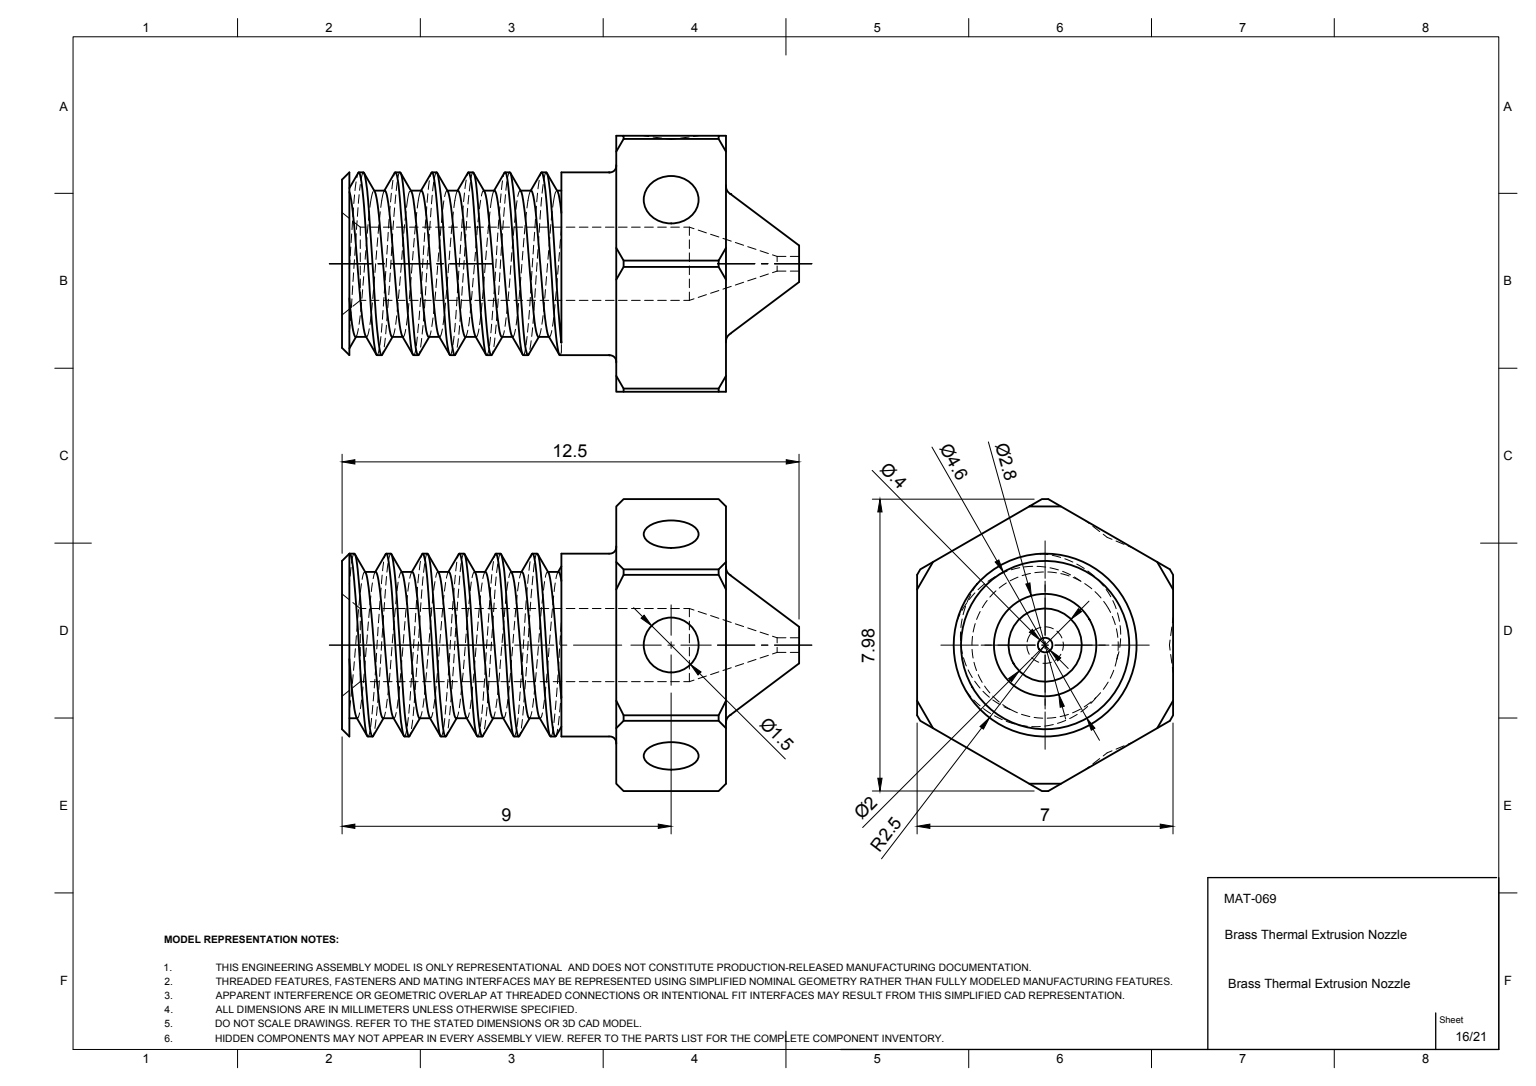
ISO-10303-21;
HEADER;
/* Generated by software containing ST-Developer
 * from STEP Tools, Inc. (www.steptools.com) 
 */

FILE_DESCRIPTION(
/* description */ ('CAx-IF Rec.Pracs.---Representation and Presentation of Product Manufa
cturing Information (PMI)---4.0---2014-10-13'),
/* implementation_level */ '2;1');

FILE_NAME(
/* name */ 'Brass Thermal Extrusion Nozzle.step',
/* time_stamp */ '2026-10-24T15:08:39-07:00',
/* author */ (''),
/* organization */ (''),
/* preprocessor_version */ 'ST-DEVELOPER v20.2',
/* originating_system */ 'Autodesk Translation Framework v15.17.0.0',
/* authorisation */ '');

FILE_SCHEMA (('AP242_MANAGED_MODEL_BASED_3D_ENGINEERING_MIM_LF { 1 0 10303 442 2 1 4 }'));
ENDSEC;

DATA;
#10=MECHANICAL_DESIGN_GEOMETRIC_PRESENTATION_REPRESENTATION('',(#833),#50081);
#110=B_SPLINE_SURFACE_WITH_KNOTS('',3,3,((#42024,#42025,#42026,#42027,#42028,
#42029,#42030,#42031,#42032,#42033),(#42034,#42035,#42036,#42037,#42038,
#42039,#42040,#42041,#42042,#42043),(#42044,#42045,#42046,#42047,#42048,
#42049,#42050,#42051,#42052,#42053),(#42054,#42055,#42056,#42057,#42058,
#42059,#42060,#42061,#42062,#42063),(#42064,#42065,#42066,#42067,#42068,
#42069,#42070,#42071,#42072,#42073),(#42074,#42075,#42076,#42077,#42078,
#42079,#42080,#42081,#42082,#42083),(#42084,#42085,#42086,#42087,#42088,
#42089,#42090,#42091,#42092,#42093)),.UNSPECIFIED.,.F.,.T.,.F.,(4,1,1,1,
4),(4,1,1,1,1,1,1,4),(-5.25936583692706E-5,0.285714285714286,0.5,0.785714285714286,
1.0342278679463),(-3.14159265358979,-2.24399475256414,-1.34639685153848,
-0.448798950512828,0.448798950512828,1.34639685153848,2.24399475256414,
3.14159265358979),.UNSPECIFIED.);
#111=B_SPLINE_SURFACE_WITH_KNOTS('',3,3,((#43523,#43524,#43525,#43526,#43527,
#43528,#43529,#43530,#43531,#43532),(#43533,#43534,#43535,#43536,#43537,
#43538,#43539,#43540,#43541,#43542),(#43543,#43544,#43545,#43546,#43547,
#43548,#43549,#43550,#43551,#43552),(#43553,#43554,#43555,#43556,#43557,
#43558,#43559,#43560,#43561,#43562),(#43563,#43564,#43565,#43566,#43567,
#43568,#43569,#43570,#43571,#43572),(#43573,#43574,#43575,#43576,#43577,
#43578,#43579,#43580,#43581,#43582),(#43583,#43584,#43585,#43586,#43587,
#43588,#43589,#43590,#43591,#43592)),.UNSPECIFIED.,.F.,.T.,.F.,(4,1,1,1,
4),(4,1,1,1,1,1,1,4),(0.,0.285714285714286,0.5,0.785714285714286,1.0345115737164),
(-9.42477796076937,-8.52718005974372,-7.62958215871806,-6.73198425769241,
-5.83438635666675,-4.9367884556411,-4.03919055461544,-3.14159265358979),
 .UNSPECIFIED.);
#112=B_SPLINE_SURFACE_WITH_KNOTS('',3,3,((#43768,#43769,#43770,#43771,#43772,
#43773,#43774,#43775,#43776,#43777),(#43778,#43779,#43780,#43781,#43782,
#43783,#43784,#43785,#43786,#43787),(#43788,#43789,#43790,#43791,#43792,
#43793,#43794,#43795,#43796,#43797),(#43798,#43799,#43800,#43801,#43802,
#43803,#43804,#43805,#43806,#43807),(#43808,#43809,#43810,#43811,#43812,
#43813,#43814,#43815,#43816,#43817),(#43818,#43819,#43820,#43821,#43822,
#43823,#43824,#43825,#43826,#43827),(#43828,#43829,#43830,#43831,#43832,
#43833,#43834,#43835,#43836,#43837)),.UNSPECIFIED.,.F.,.T.,.F.,(4,1,1,1,
4),(4,1,1,1,1,1,1,4),(-0.0291943928156984,0.285714285714286,0.571428571428571,
0.785714285714286,1.),(-3.14159265358979,-2.24399475256414,-1.34639685153848,
-0.448798950512828,0.448798950512828,1.34639685153848,2.24399475256414,
3.14159265358979),.UNSPECIFIED.);
#113=B_SPLINE_SURFACE_WITH_KNOTS('',3,3,((#43991,#43992,#43993,#43994,#43995,
#43996,#43997,#43998,#43999,#44000,#44001,#44002,#44003,#44004,#44005,#44006,
#44007,#44008,#44009,#44010,#44011,#44012,#44013,#44014,#44015,#44016,#44017,
#44018,#44019,#44020,#44021,#44022,#44023,#44024,#44025,#44026,#44027,#44028,
#44029,#44030,#44031,#44032),(#44033,#44034,#44035,#44036,#44037,#44038,
#44039,#44040,#44041,#44042,#44043,#44044,#44045,#44046,#44047,#44048,#44049,
#44050,#44051,#44052,#44053,#44054,#44055,#44056,#44057,#44058,#44059,#44060,
#44061,#44062,#44063,#44064,#44065,#44066,#44067,#44068,#44069,#44070,#44071,
#44072,#44073,#44074),(#44075,#44076,#44077,#44078,#44079,#44080,#44081,
#44082,#44083,#44084,#44085,#44086,#44087,#44088,#44089,#44090,#44091,#44092,
#44093,#44094,#44095,#44096,#44097,#44098,#44099,#44100,#44101,#44102,#44103,
#44104,#44105,#44106,#44107,#44108,#44109,#44110,#44111,#44112,#44113,#44114,
#44115,#44116),(#44117,#44118,#44119,#44120,#44121,#44122,#44123,#44124,
#44125,#44126,#44127,#44128,#44129,#44130,#44131,#44132,#44133,#44134,#44135,
#44136,#44137,#44138,#44139,#44140,#44141,#44142,#44143,#44144,#44145,#44146,
#44147,#44148,#44149,#44150,#44151,#44152,#44153,#44154,#44155,#44156,#44157,
#44158)),.UNSPECIFIED.,.F.,.F.,.F.,(4,4),(4,1,1,1,1,1,1,1,1,1,1,1,1,1,1,
1,1,1,1,1,1,1,1,1,1,1,1,1,1,1,1,1,1,1,1,1,1,1,1,4),(-0.000319347032471544,
0.058673081183855),(8.32512525661541,9.30615063831745,10.287080744622,11.2680108509265,
12.248940957231,13.2298710635355,14.21080116984,15.1917312761445,16.172661382449,
17.1535914887535,18.134521595058,19.1154517013625,20.096381807667,21.0773119139715,
22.0582420202761,23.0391721265806,24.0201022328851,25.0010323391896,25.9819624454941,
26.9628925517986,27.9438226581031,28.9247527644076,29.9056828707121,30.8866129770166,
31.8675430833211,32.8484731896256,33.8294032959301,34.8103334022347,35.7912635085392,
36.7721936148437,37.7531237211482,38.7340538274527,39.7149839337572,40.6959140400617,
41.6768441463662,42.6577742526707,43.6387043589752,44.6196344652797,45.6005645715842,
46.5816623403953),.UNSPECIFIED.);
#114=B_SPLINE_SURFACE_WITH_KNOTS('',3,3,((#44258,#44259,#44260,#44261,#44262,
#44263,#44264,#44265,#44266,#44267,#44268,#44269,#44270,#44271,#44272,#44273,
#44274,#44275,#44276,#44277,#44278,#44279,#44280,#44281,#44282,#44283,#44284,
#44285,#44286,#44287,#44288,#44289,#44290,#44291,#44292,#44293,#44294,#44295,
#44296,#44297,#44298,#44299),(#44300,#44301,#44302,#44303,#44304,#44305,
#44306,#44307,#44308,#44309,#44310,#44311,#44312,#44313,#44314,#44315,#44316,
#44317,#44318,#44319,#44320,#44321,#44322,#44323,#44324,#44325,#44326,#44327,
#44328,#44329,#44330,#44331,#44332,#44333,#44334,#44335,#44336,#44337,#44338,
#44339,#44340,#44341),(#44342,#44343,#44344,#44345,#44346,#44347,#44348,
#44349,#44350,#44351,#44352,#44353,#44354,#44355,#44356,#44357,#44358,#44359,
#44360,#44361,#44362,#44363,#44364,#44365,#44366,#44367,#44368,#44369,#44370,
#44371,#44372,#44373,#44374,#44375,#44376,#44377,#44378,#44379,#44380,#44381,
#44382,#44383),(#44384,#44385,#44386,#44387,#44388,#44389,#44390,#44391,
#44392,#44393,#44394,#44395,#44396,#44397,#44398,#44399,#44400,#44401,#44402,
#44403,#44404,#44405,#44406,#44407,#44408,#44409,#44410,#44411,#44412,#44413,
#44414,#44415,#44416,#44417,#44418,#44419,#44420,#44421,#44422,#44423,#44424,
#44425)),.UNSPECIFIED.,.F.,.F.,.F.,(4,4),(4,1,1,1,1,1,1,1,1,1,1,1,1,1,1,
1,1,1,1,1,1,1,1,1,1,1,1,1,1,1,1,1,1,1,1,1,1,1,1,4),(-0.000918461422766351,
0.0581489398467419),(12.0088396942433,12.9901384178654,13.9710685241699,
14.9519986304744,15.9329287367789,16.9138588430834,17.8947889493879,18.8757190556924,
19.8566491619969,20.8375792683014,21.8185093746059,22.7994394809105,23.780369587215,
24.7612996935195,25.742229799824,26.7231599061285,27.704090012433,28.6850201187375,
29.665950225042,30.6468803313465,31.627810437651,32.6087405439555,33.58967065026,
34.5706007565645,35.5515308628691,36.5324609691736,37.5133910754781,38.4943211817826,
39.4752512880871,40.4561813943916,41.4371115006961,42.4180416070006,43.3989717133051,
44.3799018196096,45.3608319259141,46.3417620322186,47.3226921385232,48.3036222448277,
49.2845523511322,50.2660355937093),.UNSPECIFIED.);
#457=B_SPLINE_CURVE_WITH_KNOTS('',3,(#40497,#40498,#40499,#40500,#40501,
#40502,#40503,#40504,#40505,#40506,#40507,#40508,#40509,#40510,#40511,#40512,
#40513,#40514,#40515,#40516,#40517,#40518,#40519,#40520,#40521,#40522,#40523,
#40524,#40525,#40526,#40527,#40528,#40529,#40530,#40531,#40532,#40533,#40534,
#40535,#40536,#40537,#40538,#40539,#40540,#40541,#40542,#40543,#40544,#40545,
#40546),.UNSPECIFIED.,.F.,.F.,(4,2,2,2,2,2,2,2,2,2,2,2,2,2,2,2,2,2,2,2,
2,2,2,2,4),(0.000209493712794322,0.0422872913938982,0.0542226665498989,
0.0656299001912059,0.0761984914852202,0.0887188350368748,0.144055532882821,
0.166979316880622,0.181775163552867,0.188803136528792,0.194952964302586,
0.204776397594916,0.236321457818492,0.28877412063129,0.301515346905665,
0.312233055563606,0.323797735338658,0.344187219178032,0.372232761612485,
0.42043174817154,0.429529383616972,0.435416861196921,0.440637222272047,
0.447327481728966,0.472483010091814),.UNSPECIFIED.);
#458=B_SPLINE_CURVE_WITH_KNOTS('',3,(#40549,#40550,#40551,#40552,#40553,
#40554,#40555,#40556,#40557,#40558,#40559,#40560,#40561,#40562,#40563,#40564,
#40565,#40566,#40567,#40568,#40569,#40570,#40571,#40572,#40573,#40574,#40575,
#40576,#40577,#40578),.UNSPECIFIED.,.F.,.F.,(4,2,2,2,2,2,2,2,2,2,2,2,2,
2,4),(9.99999999571378E-7,0.00565775487530941,0.0129173728394934,0.0519474282669346,
0.0924692038786361,0.106536967386471,0.118140574424233,0.132780272231367,
0.172415521622109,0.222944405297024,0.236545301367104,0.243410862645757,
0.249272230574711,0.258478354896224,0.275556593261106),.UNSPECIFIED.);
#459=B_SPLINE_CURVE_WITH_KNOTS('',3,(#40584,#40585,#40586,#40587,#40588,
#40589,#40590,#40591,#40592,#40593,#40594,#40595,#40596,#40597,#40598,#40599,
#40600,#40601,#40602,#40603,#40604,#40605,#40606,#40607,#40608,#40609,#40610,
#40611,#40612,#40613,#40614,#40615,#40616,#40617,#40618,#40619,#40620,#40621,
#40622,#40623,#40624,#40625,#40626,#40627,#40628,#40629,#40630,#40631,#40632,
#40633,#40634,#40635,#40636,#40637,#40638,#40639,#40640,#40641,#40642,#40643,
#40644,#40645,#40646,#40647,#40648,#40649,#40650,#40651,#40652,#40653,#40654,
#40655,#40656,#40657,#40658,#40659,#40660,#40661,#40662,#40663,#40664,#40665,
#40666,#40667,#40668,#40669,#40670,#40671,#40672,#40673,#40674,#40675,#40676,
#40677,#40678,#40679,#40680,#40681,#40682,#40683,#40684,#40685,#40686,#40687,
#40688,#40689,#40690,#40691,#40692,#40693,#40694,#40695,#40696,#40697,#40698,
#40699,#40700,#40701,#40702,#40703,#40704,#40705,#40706,#40707,#40708,#40709,
#40710,#40711,#40712,#40713,#40714,#40715,#40716,#40717,#40718,#40719,#40720,
#40721,#40722,#40723,#40724,#40725,#40726,#40727,#40728,#40729,#40730,#40731,
#40732,#40733,#40734,#40735,#40736,#40737,#40738,#40739,#40740,#40741),
 .UNSPECIFIED.,.F.,.F.,(4,2,2,2,2,2,2,2,2,2,2,2,2,2,2,2,2,2,2,2,2,2,2,2,
2,2,2,2,2,2,2,2,2,2,2,2,2,2,2,2,2,2,2,2,2,2,2,2,2,2,2,2,2,2,2,2,2,2,2,2,
2,2,2,2,2,2,2,2,2,2,2,2,2,2,2,2,2,2,4),(6.30435270860889,6.33486878320123,
6.34366974614675,6.34966324284323,6.35703713755435,6.37420620250057,6.40375264025194,
6.4470390695231,6.46203191150256,6.47264308026978,6.48406809681009,6.50407751685343,
6.53144912706435,6.58091498964814,6.58971900104101,6.59571521178631,6.60309649351356,
6.62029862705322,6.64995101906424,6.693024043224,6.708012300807,6.71862649719076,
6.73006138331729,6.75011057786636,6.7775645954391,6.82685633546438,6.83568099086117,
6.84167591283988,6.8490295334854,6.8660798204813,6.89526589896446,6.93907381839847,
6.9540616271593,6.96466389709236,6.97607323881813,6.99603127669263,7.02329568207772,
7.07302291161279,7.08179288524694,7.087779399277,7.09516137744094,7.11239908891738,
7.14215363461921,7.18521725183071,7.20021562855414,7.21082892841909,7.22225457039669,
7.24226256268532,7.26963720002217,7.31902650273789,7.3278387071296,7.3338469765065,
7.34126629547086,7.35864634523377,7.3888709987462,7.43087825960643,7.44583940029455,
7.45646854729715,7.46795493496144,7.48821541141176,7.51611323660128,7.56446287865684,
7.57339841015601,7.57939406940583,7.586623356302,7.60299394716167,7.63017917440611,
7.67742899532298,7.69229453732945,7.70282865451226,7.71416963637204,7.73398882738903,
7.76099878006726,7.81118536759106,7.81992573892269,7.82589410585711,7.83325762804537,
7.84165606901659,7.87995889022397),.UNSPECIFIED.);
#460=B_SPLINE_CURVE_WITH_KNOTS('',3,(#40742,#40743,#40744,#40745),
 .UNSPECIFIED.,.F.,.F.,(4,4),(1.01357413598985E-6,0.000209493712794322),
 .UNSPECIFIED.);
#461=B_SPLINE_CURVE_WITH_KNOTS('',3,(#40746,#40747,#40748,#40749,#40750,
#40751,#40752,#40753,#40754,#40755,#40756,#40757,#40758,#40759,#40760,#40761,
#40762,#40763,#40764,#40765,#40766,#40767,#40768,#40769,#40770,#40771,#40772,
#40773,#40774,#40775,#40776,#40777,#40778,#40779,#40780,#40781,#40782,#40783,
#40784,#40785,#40786,#40787,#40788,#40789,#40790,#40791,#40792,#40793,#40794,
#40795,#40796,#40797,#40798,#40799,#40800,#40801,#40802,#40803,#40804,#40805,
#40806,#40807,#40808,#40809,#40810,#40811,#40812,#40813,#40814,#40815,#40816,
#40817,#40818,#40819,#40820,#40821,#40822,#40823,#40824,#40825,#40826,#40827,
#40828,#40829,#40830,#40831,#40832,#40833,#40834,#40835,#40836,#40837,#40838,
#40839,#40840,#40841,#40842,#40843,#40844,#40845,#40846,#40847,#40848,#40849,
#40850,#40851,#40852,#40853,#40854,#40855,#40856,#40857,#40858,#40859,#40860,
#40861,#40862,#40863,#40864,#40865,#40866,#40867,#40868,#40869,#40870,#40871,
#40872,#40873,#40874,#40875,#40876,#40877,#40878,#40879,#40880,#40881,#40882,
#40883,#40884,#40885,#40886,#40887,#40888,#40889,#40890,#40891,#40892,#40893,
#40894,#40895,#40896,#40897,#40898,#40899,#40900,#40901),.UNSPECIFIED.,
 .F.,.F.,(4,2,2,2,2,2,2,2,2,2,2,2,2,2,2,2,2,2,2,2,2,2,2,2,2,2,2,2,2,2,2,
2,2,2,2,2,2,2,2,2,2,2,2,2,2,2,2,2,2,2,2,2,2,2,2,2,2,2,2,2,2,2,2,2,2,2,2,
2,2,2,2,2,2,2,2,2,2,4),(0.275556593261106,0.302257716093375,0.332145449002062,
0.353019638320446,0.364182811346166,0.374094054396295,0.387016365935024,
0.424468399690209,0.474784838723073,0.486382245753939,0.49262015904604,
0.498086515168979,0.507668815230086,0.549849706736197,0.580898810950735,
0.602581422114444,0.614391844510637,0.625103828088379,0.639873751023731,
0.68612813271093,0.712253967143993,0.728243775062982,0.73554602991629,0.741707481959803,
0.751244469819963,0.794030213469046,0.824223859030593,0.845430043251126,
0.857061734857099,0.867632782348189,0.882182911159433,0.941047537998989,
0.96150213928913,0.97527996369794,0.982123309918813,0.98815353536044,0.997879223181914,
1.04633441080135,1.07317249406427,1.09290377583721,1.10421640948278,1.11473376705714,
1.12958982902173,1.17659174660286,1.20386064199112,1.22025213524982,1.22747630986562,
1.23345821413433,1.24235725539788,1.29095061193003,1.3187384153877,1.33893993740818,
1.35040225813014,1.36101160205548,1.37594642745454,1.41769551255673,1.4480412350592,
1.46544943938522,1.47286386661574,1.47885850768789,1.4876337927126,1.5372593554286,
1.56452795041183,1.58447799162328,1.59587951676874,1.60647281319572,1.62144445402929,
1.66411223318268,1.69407854731155,1.7113737724098,1.7187549102345,1.72472703980151,
1.73345363173632,1.78346592748571,1.81060244195952,1.83049217765482,1.84187542645257,
1.85022063120531),.UNSPECIFIED.);
#462=B_SPLINE_CURVE_WITH_KNOTS('',3,(#40906,#40907,#40908,#40909,#40910,
#40911,#40912,#40913,#40914,#40915,#40916,#40917,#40918,#40919,#40920,#40921,
#40922,#40923,#40924,#40925,#40926,#40927,#40928,#40929,#40930,#40931,#40932,
#40933,#40934,#40935,#40936,#40937,#40938,#40939,#40940,#40941,#40942,#40943,
#40944,#40945,#40946,#40947,#40948,#40949,#40950,#40951,#40952,#40953,#40954,
#40955,#40956,#40957,#40958,#40959,#40960,#40961,#40962,#40963,#40964,#40965,
#40966,#40967,#40968,#40969,#40970,#40971,#40972,#40973,#40974,#40975,#40976,
#40977,#40978,#40979,#40980,#40981,#40982,#40983,#40984,#40985,#40986,#40987,
#40988,#40989,#40990,#40991,#40992,#40993,#40994,#40995,#40996,#40997,#40998,
#40999,#41000,#41001,#41002,#41003,#41004,#41005,#41006,#41007,#41008,#41009,
#41010,#41011,#41012,#41013,#41014,#41015,#41016,#41017,#41018,#41019,#41020,
#41021,#41022,#41023,#41024,#41025,#41026,#41027,#41028,#41029,#41030,#41031,
#41032,#41033,#41034,#41035,#41036,#41037,#41038,#41039,#41040,#41041,#41042,
#41043,#41044,#41045,#41046,#41047,#41048,#41049,#41050,#41051,#41052,#41053,
#41054,#41055,#41056,#41057,#41058,#41059,#41060,#41061,#41062,#41063),
 .UNSPECIFIED.,.F.,.F.,(4,2,2,2,2,2,2,2,2,2,2,2,2,2,2,2,2,2,2,2,2,2,2,2,
2,2,2,2,2,2,2,2,2,2,2,2,2,2,2,2,2,2,2,2,2,2,2,2,2,2,2,2,2,2,2,2,2,2,2,2,
2,2,2,2,2,2,2,2,2,2,2,2,2,2,2,2,2,2,4),(4.72819048267577,4.73950795185586,
4.75012210979889,4.76155086895958,4.78156836809081,4.80895190741352,4.85843117911358,
4.86723766046422,4.87323362414742,4.88060942980026,4.89778064245953,4.92732947790588,
4.97061576111725,4.98561061430102,4.99622420623809,5.00765283970181,5.02767158171161,
5.05505859474814,5.10452501033381,5.11333238041157,5.119328288513,5.12670325752487,
5.14386935222794,5.17340318557322,5.21670622262401,5.23170062699955,5.24231393095466,
5.25374230849599,5.27376083811829,5.30114790257251,5.35061005460223,5.35941738370218,
5.3654130554825,5.37278737207586,5.38995088389089,5.41947774454824,5.46278794072297,
5.47778169663862,5.4883943710803,5.49982188080286,5.51983816805462,5.54722109224304,
5.59668877283127,5.6054948237148,5.61149004333747,5.61886426512492,5.63602890233187,
5.6655599240848,5.70886382307828,5.72385725358769,5.73446957571265,5.74589658496825,
5.76591167794044,5.79329281107251,5.84275834566241,5.85156409224043,5.85755945109383,
5.86493479128113,5.88210548756745,5.91165646761162,5.95492013716683,5.9699124918867,
5.98052501497582,5.99195326255171,6.0119740552566,6.03936750252539,6.08880259339068,
6.09761148824992,6.10360662335611,6.11097785502081,6.1281262103999,6.15760933171281,
6.20097342104773,6.21596522841018,6.22657577246508,6.23800016613919,6.25800788400909,
6.28537444195454,6.30435270860889),.UNSPECIFIED.);
#463=B_SPLINE_CURVE_WITH_KNOTS('',3,(#41064,#41065,#41066,#41067,#41068,
#41069,#41070,#41071,#41072,#41073,#41074,#41075,#41076,#41077,#41078,#41079,
#41080,#41081,#41082,#41083,#41084,#41085,#41086,#41087,#41088,#41089,#41090,
#41091,#41092,#41093,#41094,#41095,#41096,#41097,#41098,#41099,#41100,#41101,
#41102,#41103,#41104,#41105,#41106,#41107,#41108,#41109,#41110,#41111,#41112,
#41113,#41114,#41115,#41116,#41117,#41118,#41119,#41120,#41121,#41122,#41123,
#41124,#41125,#41126,#41127,#41128,#41129,#41130,#41131,#41132,#41133,#41134,
#41135,#41136,#41137,#41138,#41139,#41140,#41141,#41142,#41143,#41144,#41145,
#41146,#41147,#41148,#41149,#41150,#41151,#41152,#41153,#41154,#41155,#41156,
#41157,#41158,#41159,#41160,#41161,#41162,#41163,#41164,#41165,#41166,#41167,
#41168,#41169,#41170,#41171,#41172,#41173,#41174,#41175,#41176,#41177,#41178,
#41179,#41180,#41181,#41182,#41183,#41184,#41185,#41186,#41187,#41188,#41189,
#41190,#41191,#41192,#41193,#41194,#41195,#41196,#41197,#41198,#41199,#41200,
#41201,#41202,#41203,#41204,#41205,#41206,#41207,#41208,#41209,#41210,#41211,
#41212,#41213,#41214,#41215,#41216,#41217,#41218,#41219),.UNSPECIFIED.,
 .F.,.F.,(4,2,2,2,2,2,2,2,2,2,2,2,2,2,2,2,2,2,2,2,2,2,2,2,2,2,2,2,2,2,2,
2,2,2,2,2,2,2,2,2,2,2,2,2,2,2,2,2,2,2,2,2,2,2,2,2,2,2,2,2,2,2,2,2,2,2,2,
2,2,2,2,2,2,2,2,2,2,4),(1.85022063120531,1.85245803545648,1.86742343567781,
1.91092677999263,1.94025068089833,1.95733584714856,1.9646854274236,1.97066601700574,
1.97945105943726,2.02899469267185,2.05633207510499,2.07631803047564,2.08772733025059,
2.09832096608194,2.11328308319158,2.15603372225511,2.18584052738125,2.20308163037672,
2.21045914351855,2.21644079802621,2.22520415870899,2.27492501537538,2.30217744978419,
2.32212212808228,2.33352104296743,2.34411139064825,2.35907813354066,2.40202494263366,
2.43173414326021,2.448944807865,2.45631516411609,2.46229382809607,2.47105314309451,
2.5208064963315,2.54805044763132,2.56799158078089,2.57938927809238,2.58997869927616,
2.60494442056477,2.64798095380983,2.67761542931793,2.69480159722625,2.70216859579123,
2.7081487224768,2.71691624692997,2.76660392905713,2.79387563535955,2.81382999658193,
2.82523127782325,2.83582222281463,2.85078748140468,2.89371885123636,2.92342331327636,
2.94063208540719,2.94800303400513,2.95398316784399,2.96274709136088,3.0124644483609,
3.03972253770116,3.05967032655013,3.07106994252096,3.08166033426212,3.09662625340397,
3.13959336916278,3.1692785866773,3.18648130065975,3.19385096254273,3.19983073143358,
3.20859451245861,3.2583134518259,3.28557185055764,3.3055198931902,3.31691956705066,
3.32750995083086,3.34247577477007,3.38545424338359,3.41512952594777,3.42490669701472),
 .UNSPECIFIED.);
#464=B_SPLINE_CURVE_WITH_KNOTS('',3,(#41224,#41225,#41226,#41227,#41228,
#41229,#41230,#41231,#41232,#41233,#41234,#41235,#41236,#41237,#41238,#41239,
#41240,#41241,#41242,#41243,#41244,#41245,#41246,#41247,#41248,#41249,#41250,
#41251,#41252,#41253,#41254,#41255,#41256,#41257,#41258,#41259,#41260,#41261,
#41262,#41263,#41264,#41265,#41266,#41267,#41268,#41269,#41270,#41271,#41272,
#41273,#41274,#41275,#41276,#41277,#41278,#41279,#41280,#41281,#41282,#41283,
#41284,#41285,#41286,#41287,#41288,#41289,#41290,#41291,#41292,#41293,#41294,
#41295,#41296,#41297,#41298,#41299,#41300,#41301,#41302,#41303,#41304,#41305,
#41306,#41307,#41308,#41309,#41310,#41311,#41312,#41313,#41314,#41315,#41316,
#41317,#41318,#41319,#41320,#41321,#41322,#41323,#41324,#41325,#41326,#41327,
#41328,#41329,#41330,#41331,#41332,#41333,#41334,#41335,#41336,#41337,#41338,
#41339,#41340,#41341,#41342,#41343,#41344,#41345,#41346,#41347,#41348,#41349,
#41350,#41351,#41352,#41353,#41354,#41355,#41356,#41357,#41358,#41359,#41360,
#41361,#41362,#41363,#41364,#41365,#41366,#41367,#41368,#41369,#41370,#41371,
#41372,#41373,#41374,#41375,#41376,#41377,#41378,#41379),.UNSPECIFIED.,
 .F.,.F.,(4,2,2,2,2,2,2,2,2,2,2,2,2,2,2,2,2,2,2,2,2,2,2,2,2,2,2,2,2,2,2,
2,2,2,2,2,2,2,2,2,2,2,2,2,2,2,2,2,2,2,2,2,2,2,2,2,2,2,2,2,2,2,2,2,2,2,2,
2,2,2,2,2,2,2,2,2,2,4),(3.15163477931716,3.15298897800685,3.16238915291939,
3.20652316777823,3.23631453510694,3.25737596078581,3.26897275867627,3.27952566483782,
3.29407041532064,3.35235036865309,3.3728309815977,3.3866151299212,3.39346659347139,
3.39954852935888,3.40941344026376,3.44468995601634,3.47940486850441,3.5023744208504,
3.51426586598204,3.52474840048023,3.53842769924747,3.59544554110014,3.61777418371048,
3.6323332685606,3.63931464019944,3.64534505137541,3.65487513183864,3.69766251601296,
3.72811334463534,3.74944920047817,3.76109086059298,3.77163275342468,3.78607775600029,
3.8449932390036,3.86524842884655,3.87893564142306,3.88577126146191,3.8918620139421,
3.90177670873891,3.93886568365411,3.98643481968158,4.00130483072224,4.01190269193801,
4.02337820046101,4.04367536038818,4.07168373699399,4.11973819691762,4.12870546523491,
4.13471998074014,4.14200401683087,4.15852421519058,4.18610554687911,4.23240953690924,
4.24734931712728,4.25795632477907,4.26940615582526,4.28954829302094,4.31720844817241,
4.3660547580922,4.37493356713054,4.3809377544045,4.38827163283667,4.4051410940172,
4.43376174987304,4.47841465989933,4.49340541599483,4.50401914264897,4.5154505679836,
4.53548223967792,4.56289658186719,4.61230833309369,4.62112304563995,4.6271200943582,
4.6344914860604,4.65162945556555,4.68107395400867,4.7245115038362,4.72819048267577),
 .UNSPECIFIED.);
#465=B_SPLINE_CURVE_WITH_KNOTS('',3,(#41380,#41381,#41382,#41383,#41384,
#41385,#41386,#41387,#41388,#41389,#41390,#41391,#41392,#41393,#41394,#41395,
#41396,#41397,#41398,#41399,#41400,#41401,#41402,#41403,#41404,#41405,#41406,
#41407,#41408,#41409,#41410,#41411,#41412,#41413,#41414,#41415,#41416,#41417,
#41418,#41419,#41420,#41421,#41422,#41423,#41424,#41425,#41426,#41427,#41428,
#41429,#41430,#41431,#41432,#41433,#41434,#41435,#41436,#41437,#41438,#41439,
#41440,#41441,#41442,#41443,#41444,#41445,#41446,#41447,#41448,#41449,#41450,
#41451,#41452,#41453,#41454,#41455,#41456,#41457,#41458,#41459,#41460,#41461,
#41462,#41463,#41464,#41465,#41466,#41467,#41468,#41469,#41470,#41471,#41472,
#41473,#41474,#41475,#41476,#41477,#41478,#41479,#41480,#41481,#41482,#41483,
#41484,#41485,#41486,#41487,#41488,#41489,#41490,#41491,#41492,#41493,#41494,
#41495,#41496,#41497,#41498,#41499,#41500,#41501,#41502,#41503,#41504,#41505,
#41506,#41507,#41508,#41509,#41510,#41511,#41512,#41513,#41514,#41515,#41516,
#41517,#41518,#41519,#41520,#41521,#41522,#41523,#41524,#41525,#41526,#41527,
#41528,#41529,#41530,#41531,#41532,#41533,#41534,#41535,#41536,#41537,#41538,
#41539),.UNSPECIFIED.,.F.,.F.,(4,2,2,2,2,2,2,2,2,2,2,2,2,2,2,2,2,2,2,2,
2,2,2,2,2,2,2,2,2,2,2,2,2,2,2,2,2,2,2,2,2,2,2,2,2,2,2,2,2,2,2,2,2,2,2,2,
2,2,2,2,2,2,2,2,2,2,2,2,2,2,2,2,2,2,2,2,2,2,2,4),(3.42490669701472,3.43232900937426,
3.43969829801849,3.44567833743907,3.45444340772131,3.50415231677713,3.53141504241583,
3.55136514504334,3.56276536765941,3.5733559672353,3.58832164819124,3.63127353358472,
3.66096759078479,3.6781731340077,3.68554337761954,3.69152334799716,3.70028723094562,
3.75000664143778,3.77726495614238,3.79721303103668,3.80861285460821,3.81920347093602,
3.83416980904366,3.87717038552534,3.90683077511809,3.92402561123087,3.9313943222146,
3.9373744942306,3.94614063170833,3.9958408787074,4.02310765778037,4.04305960357326,
4.05446010444556,4.06505052396108,4.08001514446103,4.1228808607337,4.15263751223124,
4.16986304230536,4.17723603423089,4.18321554998337,4.19197490861075,4.24173491283261,
4.26897644454247,4.28891702452145,4.30031571146024,4.31090697332087,4.32587722245906,
4.36937895902415,4.39868650088571,4.41576813047898,4.4231211723634,4.42910412598506,
4.43646726570338,4.45971562472414,4.50520763102599,4.53139557445127,4.54371433568145,
4.5541180054599,4.56730274768906,4.60218149192356,4.65148806356465,4.66391775308509,
4.67052045405102,4.67679960714132,4.68750057680989,4.7015915514247,4.74262703357355,
4.77468881107418,4.78787526656112,4.79827946517432,4.81059788314442,4.83678448185971,
4.88228453828832,4.90548434936197,4.91284436066545,4.91882714926359,4.92618309784467,
4.94328338218393,4.97264560048608,4.99969446742076),.UNSPECIFIED.);
#466=B_SPLINE_CURVE_WITH_KNOTS('',3,(#41544,#41545,#41546,#41547,#41548,
#41549,#41550,#41551,#41552,#41553,#41554,#41555,#41556,#41557,#41558,#41559,
#41560,#41561,#41562,#41563,#41564,#41565,#41566,#41567,#41568,#41569,#41570,
#41571,#41572,#41573,#41574,#41575,#41576,#41577,#41578,#41579,#41580,#41581,
#41582,#41583,#41584,#41585,#41586,#41587,#41588,#41589,#41590,#41591,#41592,
#41593,#41594,#41595,#41596,#41597,#41598,#41599,#41600,#41601,#41602,#41603,
#41604,#41605,#41606,#41607,#41608,#41609,#41610,#41611,#41612,#41613,#41614,
#41615,#41616,#41617,#41618,#41619,#41620,#41621,#41622,#41623,#41624,#41625,
#41626,#41627,#41628,#41629,#41630,#41631,#41632,#41633,#41634,#41635,#41636,
#41637,#41638,#41639,#41640,#41641,#41642,#41643,#41644,#41645,#41646,#41647,
#41648,#41649,#41650,#41651,#41652,#41653,#41654,#41655,#41656,#41657,#41658,
#41659,#41660,#41661,#41662,#41663,#41664,#41665,#41666,#41667,#41668,#41669,
#41670,#41671,#41672,#41673,#41674,#41675,#41676,#41677,#41678,#41679,#41680,
#41681,#41682,#41683,#41684,#41685,#41686,#41687,#41688,#41689,#41690,#41691,
#41692,#41693,#41694,#41695,#41696,#41697,#41698,#41699),.UNSPECIFIED.,
 .F.,.F.,(4,2,2,2,2,2,2,2,2,2,2,2,2,2,2,2,2,2,2,2,2,2,2,2,2,2,2,2,2,2,2,
2,2,2,2,2,2,2,2,2,2,2,2,2,2,2,2,2,2,2,2,2,2,2,2,2,2,2,2,2,2,2,2,2,2,2,2,
2,2,2,2,2,2,2,2,2,2,4),(1.57573377077494,1.62765792826645,1.64959536187562,
1.66399107840287,1.67094216055766,1.67697668986032,1.68655851418989,1.72842730949596,
1.75932678332557,1.78083900036542,1.79250216644476,1.80302743167571,1.81739114789624,
1.87670562810885,1.89678969429371,1.91039884999513,1.91721772124075,1.92331003450725,
1.93325191685743,1.97089147230866,2.00397410831103,2.0263397248044,2.03813683621378,
2.04863311602486,2.06272342571438,2.1176522354464,2.14083124951818,2.15572836792034,
2.16276251929583,2.16877142344457,2.17816783765395,2.22229373429271,2.25207163880422,
2.27312448195018,2.28471713128469,2.29526654080658,2.30980688182928,2.36806871883366,
2.38854354444909,2.40232357767318,2.4091727629334,2.41525246645886,2.42511327097463,
2.4584377159878,2.49440636690439,2.5178117205551,2.52976442851919,2.54023191880453,
2.55379343767083,2.6116463098907,2.63362193023033,2.6480349291388,2.65499078921074,
2.66102769979372,2.67061121068673,2.7125346838191,2.74342068747608,2.76493078745306,
2.77659726502315,2.78712790206586,2.80150309322966,2.86079835467284,2.88090211573173,
2.89452170521694,2.90134430867959,2.90743827759055,2.91738134281159,2.95499587952527,
2.98811449016284,3.01049649694549,3.02229829801593,3.03279684452293,3.04688704308136,
3.10187416891229,3.12504668052472,3.13994304117261,3.14697820988748,3.15163477931716),
 .UNSPECIFIED.);
#467=B_SPLINE_CURVE_WITH_KNOTS('',3,(#41700,#41701,#41702,#41703,#41704,
#41705,#41706,#41707,#41708,#41709,#41710,#41711,#41712,#41713,#41714,#41715,
#41716,#41717,#41718,#41719,#41720,#41721,#41722,#41723,#41724,#41725,#41726,
#41727,#41728,#41729,#41730,#41731,#41732,#41733,#41734,#41735,#41736,#41737,
#41738,#41739,#41740,#41741,#41742,#41743,#41744,#41745,#41746,#41747,#41748,
#41749,#41750,#41751,#41752,#41753,#41754,#41755,#41756,#41757,#41758,#41759,
#41760,#41761,#41762,#41763,#41764,#41765,#41766,#41767,#41768,#41769,#41770,
#41771,#41772,#41773,#41774,#41775,#41776,#41777,#41778,#41779,#41780,#41781,
#41782,#41783,#41784,#41785,#41786,#41787,#41788,#41789,#41790,#41791,#41792,
#41793,#41794,#41795,#41796,#41797,#41798,#41799,#41800,#41801,#41802,#41803,
#41804,#41805,#41806,#41807,#41808,#41809,#41810,#41811,#41812,#41813,#41814,
#41815,#41816,#41817,#41818,#41819,#41820,#41821,#41822,#41823,#41824,#41825,
#41826,#41827,#41828,#41829,#41830,#41831,#41832,#41833,#41834,#41835,#41836,
#41837,#41838,#41839,#41840,#41841,#41842,#41843,#41844,#41845,#41846,#41847,
#41848,#41849,#41850,#41851,#41852,#41853,#41854,#41855,#41856,#41857),
 .UNSPECIFIED.,.F.,.F.,(4,2,2,2,2,2,2,2,2,2,2,2,2,2,2,2,2,2,2,2,2,2,2,2,
2,2,2,2,2,2,2,2,2,2,2,2,2,2,2,2,2,2,2,2,2,2,2,2,2,2,2,2,2,2,2,2,2,2,2,2,
2,2,2,2,2,2,2,2,2,2,2,2,2,2,2,2,2,2,4),(4.99969446742076,5.01612222627699,
5.03109516348412,5.04168706966171,5.05308518898519,5.07302229762032,5.1002546627482,
5.14997692512985,5.15873609088758,5.1647157027327,5.17208878556789,5.1893137796041,
5.2190661229799,5.26198773137693,5.27695508294564,5.28754590343637,5.29894534460231,
5.31889228788194,5.34614704355636,5.3958124203372,5.40457756099,5.41055759285015,
5.41792650755612,5.43512281958154,5.46478613974075,5.50782924203427,5.52279756377833,
5.53338817485161,5.5447866086011,5.56472941162079,5.59197565421998,5.64165680760733,
5.65041958749698,5.65639916459359,5.66376897940814,5.68097325410772,5.71066239908315,
5.75366657805781,5.76863392821428,5.77922407496883,5.79062219761345,5.81056502390953,
5.83781199515832,5.88748687860816,5.89624982930673,5.90222928343406,5.90959871406835,
5.92680106382864,5.95648509297602,5.99949210260467,6.01445893700445,6.02504880009767,
6.03644671594783,6.05638954826976,6.08363702364114,6.13330675622669,6.14206979428491,
6.14804903332223,6.1554177543789,6.17261703184667,6.20229247583851,6.24530894913595,
6.26027522555275,6.27086448881313,6.28226153981436,6.30220205280319,6.32944519668532,
6.37912113982749,6.38788283983767,6.39386163221232,6.40123032730111,6.41843116490278,
6.44811212107449,6.49112058930372,6.50608651709517,6.51667543994895,6.52807202836461,
6.54801148982236,6.57429106571742),.UNSPECIFIED.);
#468=B_SPLINE_CURVE_WITH_KNOTS('',3,(#41860,#41861,#41862,#41863,#41864,
#41865,#41866,#41867,#41868,#41869,#41870,#41871,#41872,#41873,#41874,#41875,
#41876,#41877,#41878,#41879,#41880,#41881,#41882,#41883,#41884,#41885,#41886,
#41887,#41888,#41889),.UNSPECIFIED.,.T.,.F.,(4,2,2,2,2,2,2,2,2,2,2,2,2,
2,4),(0.,0.125,0.14292295086177,0.25,0.285800104977707,0.375,0.42861930011293,
0.5,0.571377117830905,0.625,0.714197774307772,0.75,0.857087735980742,0.875,
1.),.UNSPECIFIED.);
#469=B_SPLINE_CURVE_WITH_KNOTS('',3,(#41895,#41896,#41897,#41898,#41899,
#41900,#41901,#41902,#41903,#41904,#41905,#41906,#41907,#41908,#41909,#41910,
#41911,#41912,#41913,#41914,#41915,#41916,#41917,#41918,#41919),
 .UNSPECIFIED.,.F.,.F.,(4,3,3,3,3,3,3,3,4),(8.08098624460284E-14,0.185589856128629,
0.25,0.432168172320759,0.5,0.682168172320751,0.75,0.935589856128578,1.),
 .UNSPECIFIED.);
#470=B_SPLINE_CURVE_WITH_KNOTS('',3,(#41923,#41924,#41925,#41926,#41927,
#41928,#41929,#41930,#41931,#41932,#41933,#41934,#41935,#41936,#41937,#41938,
#41939,#41940,#41941,#41942,#41943,#41944,#41945,#41946,#41947,#41948,#41949,
#41950,#41951,#41952,#41953,#41954,#41955,#41956,#41957,#41958,#41959,#41960,
#41961,#41962,#41963,#41964,#41965,#41966,#41967,#41968,#41969,#41970,#41971,
#41972,#41973,#41974,#41975,#41976,#41977,#41978,#41979,#41980,#41981,#41982,
#41983,#41984,#41985,#41986,#41987,#41988,#41989,#41990,#41991,#41992,#41993,
#41994,#41995,#41996,#41997,#41998,#41999,#42000,#42001,#42002,#42003,#42004,
#42005,#42006,#42007,#42008,#42009,#42010,#42011,#42012,#42013,#42014,#42015,
#42016,#42017,#42018,#42019,#42020,#42021,#42022),.UNSPECIFIED.,.F.,.F.,
(4,2,2,2,2,2,2,2,2,2,2,2,2,2,2,2,2,2,2,2,2,2,2,2,2,2,2,2,2,2,2,2,2,2,2,
2,2,2,2,2,2,2,2,2,2,2,2,2,2,4),(8.14853860778369,8.16952826439388,8.21130376441472,
8.22623517802908,8.2368405400259,8.2482970281195,8.26848496361379,8.29624866877044,
8.34478884818763,8.35368295116283,8.35966224525979,8.36688375521984,8.38327081527719,
8.41053459302116,8.45755714724689,8.47240884484075,8.48292186841738,8.49422859899152,
8.51394716165414,8.54076356003648,8.58918975381341,8.59889384251938,8.60491862652603,
8.61176490778234,8.62557233139796,8.64610175919149,8.70476844526811,8.71934725585207,
8.72991779791933,8.74152915216654,8.76263341682554,8.79259020149926,8.83575324613513,
8.84524474377202,8.85139811770872,8.85871560890523,8.87482363784368,8.90129418975491,
8.94695055904045,8.96175119473661,8.97246257761506,8.98425125307571,9.00582359482735,
9.03661281625652,9.079277716991,9.08877611000028,9.09422577303682,9.10048321199873,
9.10729564609716,9.13371097451824),.UNSPECIFIED.);
#471=B_SPLINE_CURVE_WITH_KNOTS('',3,(#42096,#42097,#42098,#42099,#42100,
#42101,#42102),.UNSPECIFIED.,.F.,.F.,(4,1,1,1,4),(-1.00000000003634,-0.785714285714286,
-0.5,-0.285714285714286,0.),.UNSPECIFIED.);
#472=B_SPLINE_CURVE_WITH_KNOTS('',3,(#42106,#42107,#42108,#42109,#42110,
#42111,#42112,#42113,#42114,#42115,#42116,#42117,#42118),.UNSPECIFIED.,
 .F.,.F.,(4,3,3,3,4),(-1.00728892207246,-0.785714285714271,-0.499999999999975,
-0.285714285714254,-0.00388490843767506),.UNSPECIFIED.);
#473=B_SPLINE_CURVE_WITH_KNOTS('',3,(#42119,#42120,#42121,#42122,#42123,
#42124,#42125,#42126,#42127,#42128,#42129,#42130,#42131,#42132,#42133,#42134),
 .UNSPECIFIED.,.F.,.F.,(4,2,2,2,2,2,2,4),(0.,0.125,0.142930238992666,0.25,
0.285797996648243,0.375,0.428625070295843,0.5),.UNSPECIFIED.);
#474=B_SPLINE_CURVE_WITH_KNOTS('',3,(#42136,#42137,#42138,#42139,#42140,
#42141,#42142,#42143,#42144,#42145,#42146,#42147,#42148,#42149,#42150,#42151,
#42152,#42153,#42154,#42155,#42156,#42157,#42158,#42159,#42160,#42161,#42162,
#42163,#42164,#42165,#42166,#42167,#42168,#42169,#42170,#42171,#42172,#42173,
#42174,#42175,#42176,#42177,#42178,#42179,#42180,#42181,#42182,#42183,#42184,
#42185,#42186,#42187,#42188,#42189,#42190,#42191,#42192,#42193,#42194,#42195,
#42196,#42197,#42198,#42199,#42200,#42201,#42202,#42203,#42204,#42205,#42206,
#42207,#42208,#42209,#42210,#42211,#42212,#42213,#42214,#42215,#42216,#42217,
#42218,#42219,#42220,#42221,#42222,#42223,#42224,#42225,#42226,#42227,#42228,
#42229,#42230,#42231,#42232,#42233,#42234,#42235,#42236,#42237,#42238,#42239,
#42240,#42241,#42242,#42243,#42244,#42245,#42246,#42247,#42248,#42249,#42250,
#42251,#42252,#42253,#42254,#42255,#42256,#42257,#42258,#42259,#42260,#42261,
#42262,#42263,#42264,#42265,#42266,#42267,#42268,#42269,#42270,#42271,#42272,
#42273,#42274,#42275,#42276,#42277,#42278,#42279,#42280,#42281,#42282,#42283,
#42284,#42285,#42286,#42287,#42288,#42289,#42290,#42291,#42292,#42293),
 .UNSPECIFIED.,.F.,.F.,(4,2,2,2,2,2,2,2,2,2,2,2,2,2,2,2,2,2,2,2,2,2,2,2,
2,2,2,2,2,2,2,2,2,2,2,2,2,2,2,2,2,2,2,2,2,2,2,2,2,2,2,2,2,2,2,2,2,2,2,2,
2,2,2,2,2,2,2,2,2,2,2,2,2,2,2,2,2,2,4),(0.000492563516689082,0.0341773825702078,
0.0575679327368054,0.0695405979140284,0.080049251897907,0.0937029164043512,
0.151407163606198,0.173705220541313,0.188260994861637,0.195239466532897,
0.201229835610513,0.210651604612185,0.254192847398101,0.284228886612211,
0.305357526206893,0.316905967924253,0.327360354313765,0.341661949166553,
0.401357262672953,0.421409295931973,0.434990789447019,0.441773538848331,
0.447845020942935,0.457705587063812,0.491936437561936,0.527323937432171,
0.550541172588345,0.562482488398015,0.572980379233105,0.586646844990631,
0.643384374021231,0.665625338642604,0.680145545196282,0.687132637128509,
0.693179422881149,0.702781210952997,0.744025731518034,0.77522830088162,
0.796856261903557,0.808537183417919,0.819058257864295,0.833383886246761,
0.893022300843321,0.913019973709865,0.92659117754553,0.933400964082066,
0.939487126547021,0.949422006253815,0.9876332057857,1.02034457517022,1.0425628713401,
1.05432752661319,1.06481341692,1.0789159362931,1.13367863289971,1.15693108349076,
1.17185362339831,1.17888626616877,1.1848894220167,1.19426317033574,1.23857413766376,
1.26825527692179,1.28926748143279,1.30085452805911,1.31140795327241,1.32597043241504,
1.3840113167314,1.40453338966003,1.4183327500512,1.42518637685489,1.43126538812174,
1.4411230076461,1.47423916106134,1.51032084223349,1.53376037562423,1.54571514203592,
1.55617812384814,1.56972476147254,1.57573377077494),.UNSPECIFIED.);
#475=B_SPLINE_CURVE_WITH_KNOTS('',3,(#42294,#42295,#42296,#42297,#42298,
#42299,#42300,#42301,#42302,#42303,#42304,#42305,#42306,#42307,#42308,#42309,
#42310,#42311,#42312,#42313,#42314,#42315,#42316,#42317,#42318,#42319,#42320,
#42321,#42322,#42323,#42324,#42325,#42326,#42327,#42328,#42329,#42330,#42331,
#42332,#42333,#42334,#42335,#42336,#42337,#42338,#42339,#42340,#42341,#42342,
#42343,#42344,#42345,#42346,#42347,#42348,#42349,#42350,#42351,#42352,#42353,
#42354,#42355,#42356,#42357,#42358,#42359,#42360,#42361,#42362,#42363,#42364,
#42365,#42366,#42367,#42368,#42369,#42370,#42371,#42372,#42373,#42374,#42375,
#42376,#42377,#42378,#42379,#42380,#42381,#42382,#42383,#42384,#42385,#42386,
#42387,#42388,#42389,#42390,#42391,#42392,#42393,#42394,#42395,#42396,#42397,
#42398,#42399,#42400,#42401,#42402,#42403,#42404,#42405,#42406,#42407,#42408,
#42409,#42410,#42411,#42412,#42413,#42414,#42415,#42416,#42417,#42418,#42419,
#42420,#42421,#42422,#42423,#42424,#42425,#42426,#42427,#42428,#42429,#42430,
#42431,#42432,#42433,#42434,#42435,#42436,#42437,#42438,#42439,#42440,#42441,
#42442,#42443,#42444,#42445,#42446,#42447,#42448,#42449,#42450,#42451,#42452,
#42453),.UNSPECIFIED.,.F.,.F.,(4,2,2,2,2,2,2,2,2,2,2,2,2,2,2,2,2,2,2,2,
2,2,2,2,2,2,2,2,2,2,2,2,2,2,2,2,2,2,2,2,2,2,2,2,2,2,2,2,2,2,2,2,2,2,2,2,
2,2,2,2,2,2,2,2,2,2,2,2,2,2,2,2,2,2,2,2,2,2,2,4),(6.57429106571742,6.57525312780825,
6.62492647305338,6.63368794510889,6.63966689284873,6.64703667225612,6.664243319311,
6.69394354699268,6.73691334989607,6.75187810133236,6.76246721858811,6.7738650909055,
6.79381047113821,6.82106484856978,6.8707067458127,6.87947153249801,6.88545027371608,
6.89281584938557,6.90999927630054,6.93962843610894,6.98270214150769,6.99766683268721,
7.00825406798716,7.01964798195614,7.03957951401267,7.0668053321817,7.11651096144781,
7.12526727912624,7.13124435902373,7.13861302368273,7.15582021492245,7.18552258815762,
7.2285057924792,7.24347103047062,7.25405883896717,7.26545357522281,7.2853879155563,
7.31262115632881,7.36229296993982,7.37105299601105,7.37703285822145,7.38440845393583,
7.40164566696,7.43144510282038,7.47422987238597,7.48919000344632,7.49978074330808,
7.51118546323947,7.53116031983854,7.55847739348733,7.60797073119219,7.61675207961588,
7.62273067714667,7.63007813321545,7.64715914178237,7.67647586609909,7.72001071707904,
7.73497347848119,7.74555282386888,7.7569311847097,7.77680955932541,7.80392574551293,
7.85388397829139,7.86260685946152,7.86857681560139,7.87595541755871,7.89324468633585,
7.92319870849767,7.96590180693535,7.98087055981519,7.99146026296552,8.00285641024184,
8.02279382133068,8.05003986018625,8.09961288982266,8.10838377760247,8.1143759906819,
8.12178784521217,8.13919108703434,8.14853860778369),.UNSPECIFIED.);
#476=B_SPLINE_CURVE_WITH_KNOTS('',3,(#42457,#42458,#42459,#42460,#42461,
#42462,#42463,#42464,#42465,#42466,#42467,#42468,#42469,#42470,#42471,#42472,
#42473,#42474,#42475,#42476,#42477,#42478,#42479,#42480,#42481,#42482,#42483,
#42484,#42485,#42486,#42487,#42488,#42489,#42490,#42491,#42492,#42493,#42494,
#42495,#42496,#42497,#42498,#42499,#42500,#42501,#42502,#42503,#42504,#42505,
#42506,#42507,#42508,#42509,#42510,#42511,#42512,#42513,#42514,#42515,#42516,
#42517,#42518,#42519,#42520,#42521,#42522,#42523,#42524,#42525,#42526,#42527,
#42528,#42529,#42530,#42531,#42532,#42533,#42534,#42535,#42536,#42537,#42538,
#42539,#42540,#42541,#42542,#42543,#42544,#42545,#42546,#42547,#42548,#42549,
#42550,#42551,#42552,#42553,#42554,#42555,#42556,#42557,#42558,#42559,#42560,
#42561,#42562,#42563,#42564,#42565,#42566,#42567,#42568,#42569,#42570,#42571,
#42572,#42573,#42574,#42575,#42576,#42577,#42578,#42579,#42580,#42581,#42582,
#42583,#42584,#42585,#42586,#42587,#42588,#42589,#42590,#42591,#42592,#42593,
#42594,#42595,#42596,#42597,#42598,#42599,#42600,#42601,#42602,#42603,#42604,
#42605,#42606,#42607,#42608,#42609,#42610,#42611,#42612,#42613,#42614,#42615,
#42616,#42617,#42618,#42619,#42620,#42621,#42622,#42623,#42624,#42625,#42626,
#42627,#42628,#42629,#42630,#42631,#42632,#42633,#42634,#42635,#42636,#42637,
#42638,#42639,#42640,#42641,#42642,#42643,#42644,#42645,#42646,#42647,#42648,
#42649,#42650,#42651,#42652,#42653,#42654,#42655,#42656,#42657,#42658,#42659,
#42660,#42661,#42662,#42663,#42664,#42665,#42666,#42667,#42668,#42669,#42670,
#42671,#42672,#42673,#42674,#42675,#42676,#42677,#42678,#42679,#42680,#42681,
#42682,#42683,#42684,#42685,#42686,#42687,#42688,#42689,#42690,#42691,#42692,
#42693,#42694,#42695,#42696,#42697,#42698,#42699,#42700,#42701,#42702,#42703,
#42704,#42705,#42706,#42707,#42708,#42709,#42710,#42711,#42712,#42713,#42714,
#42715,#42716,#42717,#42718,#42719,#42720,#42721,#42722,#42723,#42724,#42725,
#42726,#42727,#42728,#42729,#42730,#42731,#42732,#42733,#42734,#42735,#42736,
#42737,#42738,#42739,#42740,#42741,#42742,#42743,#42744,#42745,#42746,#42747,
#42748,#42749,#42750,#42751,#42752,#42753,#42754,#42755,#42756,#42757,#42758,
#42759,#42760,#42761,#42762,#42763,#42764,#42765,#42766,#42767,#42768,#42769,
#42770,#42771,#42772,#42773,#42774,#42775,#42776,#42777,#42778,#42779,#42780,
#42781,#42782,#42783,#42784,#42785,#42786,#42787,#42788,#42789,#42790,#42791,
#42792,#42793,#42794,#42795,#42796,#42797,#42798,#42799,#42800,#42801,#42802,
#42803,#42804,#42805,#42806,#42807,#42808,#42809,#42810,#42811,#42812,#42813,
#42814,#42815,#42816,#42817,#42818,#42819,#42820,#42821,#42822,#42823,#42824,
#42825,#42826,#42827,#42828,#42829,#42830,#42831,#42832,#42833,#42834,#42835,
#42836,#42837,#42838,#42839,#42840,#42841,#42842,#42843,#42844,#42845,#42846,
#42847,#42848,#42849,#42850,#42851,#42852,#42853,#42854,#42855,#42856,#42857,
#42858,#42859,#42860,#42861,#42862,#42863,#42864,#42865,#42866,#42867,#42868,
#42869,#42870,#42871,#42872,#42873,#42874,#42875,#42876,#42877,#42878,#42879,
#42880,#42881,#42882,#42883,#42884,#42885,#42886,#42887,#42888,#42889,#42890,
#42891,#42892,#42893,#42894,#42895,#42896,#42897,#42898,#42899,#42900,#42901,
#42902,#42903,#42904,#42905,#42906,#42907,#42908,#42909,#42910,#42911,#42912,
#42913,#42914,#42915,#42916,#42917,#42918,#42919,#42920,#42921,#42922,#42923,
#42924,#42925,#42926,#42927,#42928,#42929,#42930,#42931,#42932,#42933,#42934,
#42935,#42936,#42937,#42938,#42939,#42940,#42941,#42942,#42943,#42944,#42945,
#42946,#42947,#42948,#42949,#42950,#42951,#42952,#42953,#42954,#42955,#42956,
#42957,#42958,#42959,#42960,#42961,#42962,#42963,#42964,#42965,#42966,#42967,
#42968,#42969,#42970,#42971,#42972,#42973,#42974,#42975,#42976,#42977,#42978,
#42979,#42980,#42981,#42982,#42983,#42984,#42985,#42986,#42987,#42988,#42989,
#42990,#42991,#42992,#42993,#42994,#42995,#42996,#42997,#42998,#42999,#43000,
#43001,#43002,#43003,#43004,#43005,#43006,#43007,#43008,#43009,#43010,#43011,
#43012),.UNSPECIFIED.,.F.,.F.,(4,2,2,2,2,2,2,2,2,2,2,2,2,2,2,2,2,2,2,2,
2,2,2,2,2,2,2,2,2,2,2,2,2,2,2,2,2,2,2,2,2,2,2,2,2,2,2,2,2,2,2,2,2,2,2,2,
2,2,2,2,2,2,2,2,2,2,2,2,2,2,2,2,2,2,2,2,2,2,2,2,2,2,2,2,2,2,2,2,2,2,2,2,
2,2,2,2,2,2,2,2,2,2,2,2,2,2,2,2,2,2,2,2,2,2,2,2,2,2,2,2,2,2,2,2,2,2,2,2,
2,2,2,2,2,2,2,2,2,2,2,2,2,2,2,2,2,2,2,2,2,2,2,2,2,2,2,2,2,2,2,2,2,2,2,2,
2,2,2,2,2,2,2,2,2,2,2,2,2,2,2,2,2,2,2,2,2,2,2,2,2,2,2,2,2,2,2,2,2,2,2,2,
2,2,2,2,2,2,2,2,2,2,2,2,2,2,2,2,2,2,2,2,2,2,2,2,2,2,2,2,2,2,2,2,2,2,2,2,
2,2,2,2,2,2,2,2,2,2,2,2,2,2,2,2,2,2,2,2,2,2,2,2,2,2,2,2,2,2,2,2,2,2,2,2,
2,2,2,2,2,4),(-5.04396562385481,-4.9980997399527,-4.98517304167195,-4.97475139559582,
-4.96166371518258,-4.921775707794,-4.89290076511485,-4.88456488860594,-4.8785680730564,
-4.87008445784522,-4.83672939119426,-4.80028885219112,-4.78769996080878,
-4.77726507703883,-4.76400838452873,-4.73054630709276,-4.70650394910092,
-4.69619601034013,-4.68780851051061,-4.68181156156318,-4.67337915758532,
-4.63945495070001,-4.60358755870111,-4.59096148088791,-4.58052971024975,
-4.56732186964725,-4.53109971760608,-4.50881566590829,-4.49888645340053,
-4.49071720534244,-4.48471608964361,-4.47604780804978,-4.449005747584,-4.42070634761022,
-4.40666120058398,-4.39407596545333,-4.38364158980256,-4.37038253566392,
-4.33664883357748,-4.31279127262899,-4.30252191157765,-4.29415656481433,
-4.28815973320411,-4.27970570955559,-4.24601432125875,-4.20997688873402,
-4.19734388266647,-4.18691194094929,-4.17371104356827,-4.1373312314936,
-4.11513893028465,-4.10523004910812,-4.09707249032982,-4.09107049916221,
-4.08238714555653,-4.05800788480088,-4.02801990766354,-4.01362476225451,
-4.00083425924956,-3.99040814439592,-3.97716614184849,-3.93912396593494,
-3.90886908488587,-3.90050508873323,-3.89450792470256,-3.88605161859358,
-3.85237892225237,-3.8161886131112,-3.80360056947496,-3.79316571460693,
-3.77990845723896,-3.74538679304435,-3.7220542950279,-3.71189576584705,
-3.70359387915126,-3.69759597423091,-3.6890744283436,-3.6561820560895,-3.62025958972076,
-3.60735638871829,-3.59693228420076,-3.58381383094242,-3.54424147308057,
-3.51462519149695,-3.5065095921122,-3.5005051263756,-3.49177010707168,-3.45349842000022,
-3.42710425054575,-3.41273120962491,-3.40223261938362,-3.39019823640823,
-3.36569740343653,-3.36147034427012,-3.3312092116069,-3.31975449511956,
-3.3107256902233,-3.3047578718194,-3.29704216671289,-3.27225427536476,-3.24121717728329,
-3.22661595293402,-3.21370516322041,-3.20328097974073,-3.19017015830589,
-3.15050920248891,-3.12150449765795,-3.11314613088155,-3.10714867910601,
-3.09868585411656,-3.06508118920166,-3.02882775500764,-3.01624126270455,
-3.00580589278111,-2.99254559742156,-2.95879977160056,-2.93494661651809,
-2.9246777145481,-2.91631240787225,-2.91031506206288,-2.90185953622638,
-2.86817471840147,-2.8319924711787,-2.81940412294166,-2.80896896003358,
-2.79571122867243,-2.76225320730671,-2.73820079857532,-2.72789038512483,
-2.71950135489018,-2.71350420950499,-2.70507313391826,-2.67112288763767,
-2.63526778873467,-2.62264100548169,-2.61220811636895,-2.59899810347981,
-2.56279740603495,-2.54049800602625,-2.53056489713006,-2.5223931372204,
-2.51639138478821,-2.50772378236512,-2.48256899715478,-2.43843788980511,
-2.42580407415773,-2.41547151391196,-2.40210417538893,-2.37329609545325,
-2.33491239210544,-2.32618692988061,-2.32018294755467,-2.31205947587147,
-2.28219692540875,-2.24302609734378,-2.22987849102719,-2.21945384116751,
-2.20657735072229,-2.17223538648604,-2.13721553536805,-2.12888216918187,
-2.12288452532769,-2.11439581859475,-2.10391216418375,-2.07900238538826,
-2.0467674883918,-2.03354220280478,-2.0231084357258,-2.01049363347507,-1.97501370751928,
-1.94048055212601,-1.93209907102176,-1.92610170015708,-1.91766255644763,
-1.88821372113992,-1.84940963752081,-1.83623016330586,-1.82580453163593,
-1.81295620316917,-1.77753687330015,-1.74377447611805,-1.7353200520767,
-1.72932199350505,-1.72095323761138,-1.71068045451249,-1.68680241944228,
-1.6531429601866,-1.63988492492727,-1.62944829646414,-1.61685643626237,
-1.58091333839126,-1.54687011339687,-1.53844096501795,-1.53244338339867,
-1.52405137812602,-1.51373760576268,-1.4896619176958,-1.45627914048263,
-1.44302413175325,-1.432589131087,-1.41999897114718,-1.40594419482603,-1.3776177180808,
-1.35055266625314,-1.34188042274638,-1.33587876477466,-1.32771234378527,
-1.31779034355513,-1.29553657129119,-1.25928909807849,-1.24608278548942,
-1.23564916667892,-1.22301736637024,-1.18711148810971,-1.15317872555741,
-1.14473908814109,-1.13873846837883,-1.13034569787102,-1.10070203595733,
-1.0620413769319,-1.04885022177276,-1.03841875808444,-1.02556551691472,
-0.988322305896801,-0.956665726743883,-0.948072596609712,-0.942074562471509,
-0.933844274676115,-0.904768749791148,-0.864856542057289,-0.851776633085321,
-0.841361068612671,-0.828444460549937,-0.813826751526624,-0.782708281311359,
-0.757983219586049,-0.750266579081623,-0.744303167463873,-0.735295079569443,
-0.723880916128707,-0.693868839046441,-0.665207196242956,-0.653033399552585,
-0.642552720577251,-0.62842387841274,-0.611669104989387,-0.565617573062991,
-0.55561770717174,-0.549543765701532,-0.542170263894716,-0.522951951329844,
-0.476594372838271,-0.461268813403962,-0.450642607100512,-0.438951849204563,
-0.415321945435501,-0.370261879634943,-0.359532031488147,-0.353921591201462,
-0.347213117971576,-0.333193810459605,-0.3102448063465,-0.274955635025903,
-0.261740926979313,-0.251374343263263,-0.238931025985625,-0.202432263450545,
-0.168717182801042,-0.160282113829637,-0.154303257202801,-0.1459900731177,
-0.135821813315604,-0.112500651658126,-0.077610350198274,-0.0642890983207978,
-0.053806453088995,-0.0411553443408391,-0.000209718449385024),
 .UNSPECIFIED.);
#477=B_SPLINE_CURVE_WITH_KNOTS('',3,(#43014,#43015,#43016,#43017,#43018,
#43019,#43020,#43021,#43022,#43023,#43024,#43025,#43026),.UNSPECIFIED.,
 .F.,.F.,(4,3,3,3,4),(0.,0.465944417146252,0.5,0.965944417145535,0.99999951939385),
 .UNSPECIFIED.);
#478=B_SPLINE_CURVE_WITH_KNOTS('',3,(#43030,#43031,#43032,#43033,#43034,
#43035,#43036,#43037,#43038,#43039,#43040,#43041,#43042,#43043,#43044,#43045,
#43046,#43047,#43048,#43049,#43050,#43051,#43052,#43053,#43054,#43055,#43056,
#43057,#43058,#43059,#43060,#43061,#43062,#43063,#43064,#43065,#43066,#43067,
#43068,#43069,#43070,#43071,#43072,#43073,#43074,#43075,#43076,#43077,#43078,
#43079,#43080,#43081,#43082,#43083,#43084,#43085,#43086,#43087,#43088,#43089,
#43090,#43091,#43092,#43093),.UNSPECIFIED.,.F.,.F.,(4,3,3,3,3,3,3,3,3,3,
3,3,3,3,3,3,3,3,3,3,3,4),(0.,0.107672209678887,0.125,0.170875355635446,
0.231002904544599,0.25,0.341726464788695,0.356352682078381,0.375,0.481320543933706,
0.5,0.512656877147315,0.606320543933732,0.625,0.683466200655585,0.731352682078384,
0.75,0.854340962716065,0.856002904544577,0.875,0.98267220967895,1.),
 .UNSPECIFIED.);
#479=B_SPLINE_CURVE_WITH_KNOTS('',3,(#43095,#43096,#43097,#43098,#43099,
#43100,#43101,#43102,#43103,#43104,#43105,#43106,#43107,#43108,#43109,#43110,
#43111,#43112,#43113,#43114,#43115,#43116,#43117,#43118,#43119,#43120,#43121,
#43122,#43123,#43124,#43125,#43126,#43127,#43128,#43129,#43130,#43131,#43132,
#43133,#43134,#43135,#43136,#43137,#43138,#43139,#43140,#43141,#43142,#43143),
 .UNSPECIFIED.,.F.,.F.,(4,3,3,3,3,3,3,3,3,3,3,3,3,3,3,3,4),(0.,0.0980957321441499,
0.125,0.221288934213747,0.25,0.346645006971691,0.375,0.471626821224367,
0.5,0.596626821224286,0.625,0.721645006972078,0.75,0.846288934213863,0.875,
0.973095732143744,1.),.UNSPECIFIED.);
#480=B_SPLINE_CURVE_WITH_KNOTS('',3,(#43145,#43146,#43147,#43148,#43149,
#43150,#43151,#43152,#43153,#43154,#43155,#43156,#43157,#43158,#43159,#43160,
#43161,#43162,#43163,#43164,#43165,#43166,#43167,#43168,#43169,#43170,#43171,
#43172,#43173,#43174,#43175,#43176,#43177,#43178,#43179,#43180,#43181,#43182,
#43183,#43184,#43185,#43186,#43187,#43188,#43189,#43190,#43191,#43192,#43193),
 .UNSPECIFIED.,.F.,.F.,(4,3,3,3,3,3,3,3,3,3,3,3,3,3,3,3,4),(3.47866587965213E-7,
0.0980732301818695,0.125,0.221270685953323,0.25,0.346629928815369,0.375,
0.471532576649637,0.5,0.596793963593996,0.625,0.721485590978993,0.75,0.846265350404548,
0.875,0.973064073364032,0.999998966090638),.UNSPECIFIED.);
#481=B_SPLINE_CURVE_WITH_KNOTS('',3,(#43195,#43196,#43197,#43198,#43199,
#43200,#43201,#43202,#43203,#43204,#43205,#43206,#43207,#43208,#43209,#43210,
#43211,#43212,#43213,#43214,#43215,#43216,#43217,#43218,#43219,#43220,#43221,
#43222,#43223,#43224,#43225,#43226,#43227,#43228,#43229,#43230,#43231,#43232,
#43233,#43234,#43235,#43236,#43237,#43238,#43239,#43240,#43241,#43242,#43243),
 .UNSPECIFIED.,.F.,.F.,(4,3,3,3,3,3,3,3,3,3,3,3,3,3,3,3,4),(0.,0.0980882716237501,
0.125,0.221281359117661,0.25,0.346637434313584,0.375,0.471619261957286,
0.5,0.596619261956614,0.625,0.721637434313737,0.75,0.84628135911775,0.875,
0.973088271625478,1.),.UNSPECIFIED.);
#482=B_SPLINE_CURVE_WITH_KNOTS('',3,(#43245,#43246,#43247,#43248,#43249,
#43250,#43251,#43252,#43253,#43254,#43255,#43256,#43257,#43258,#43259,#43260,
#43261,#43262,#43263,#43264,#43265,#43266,#43267,#43268,#43269,#43270,#43271,
#43272,#43273,#43274,#43275,#43276,#43277,#43278,#43279,#43280,#43281,#43282,
#43283,#43284,#43285,#43286,#43287,#43288,#43289,#43290,#43291,#43292,#43293),
 .UNSPECIFIED.,.F.,.F.,(4,3,3,3,3,3,3,3,3,3,3,3,3,3,3,3,4),(0.,0.0980731050085886,
0.125,0.221265959541012,0.25,0.346622039677989,0.375,0.471603894557442,
0.5,0.596603894557873,0.625,0.721622039678259,0.75,0.846265959541324,0.875,
0.973073105008618,1.),.UNSPECIFIED.);
#483=B_SPLINE_CURVE_WITH_KNOTS('',3,(#43295,#43296,#43297,#43298,#43299,
#43300,#43301,#43302,#43303,#43304,#43305,#43306,#43307,#43308,#43309,#43310,
#43311,#43312,#43313,#43314,#43315,#43316,#43317,#43318,#43319,#43320,#43321,
#43322,#43323,#43324,#43325,#43326,#43327,#43328,#43329,#43330,#43331,#43332,
#43333,#43334,#43335,#43336,#43337,#43338,#43339,#43340,#43341,#43342,#43343),
 .UNSPECIFIED.,.F.,.F.,(4,3,3,3,3,3,3,3,3,3,3,3,3,3,3,3,4),(3.58622363903863E-7,
0.111115124155117,0.125,0.234490512890156,0.25,0.359836869680777,0.375,
0.484801042762829,0.5,0.609801042765287,0.625,0.734836869676075,0.75,0.859490512890428,
0.875,0.986114767852758,0.999999885501399),.UNSPECIFIED.);
#484=B_SPLINE_CURVE_WITH_KNOTS('',3,(#43347,#43348,#43349,#43350,#43351,
#43352,#43353,#43354,#43355,#43356,#43357,#43358,#43359,#43360,#43361,#43362,
#43363,#43364,#43365,#43366,#43367,#43368,#43369,#43370,#43371,#43372,#43373,
#43374,#43375,#43376,#43377,#43378,#43379,#43380),.UNSPECIFIED.,.F.,.F.,
(4,3,3,3,3,3,3,3,3,3,3,4),(3.20858793336893E-13,0.16551266710415,0.25,0.265228163927209,
0.411286989585918,0.5,0.530572838575572,0.661286989585927,0.75,0.795852056859227,
0.915512667103842,1.),.UNSPECIFIED.);
#485=B_SPLINE_CURVE_WITH_KNOTS('',3,(#43381,#43382,#43383,#43384,#43385,
#43386,#43387,#43388,#43389,#43390,#43391,#43392,#43393,#43394,#43395,#43396,
#43397,#43398,#43399,#43400,#43401,#43402,#43403,#43404,#43405,#43406,#43407,
#43408,#43409,#43410,#43411,#43412,#43413,#43414,#43415,#43416,#43417,#43418,
#43419,#43420,#43421,#43422,#43423,#43424,#43425,#43426,#43427,#43428,#43429,
#43430,#43431,#43432,#43433,#43434,#43435,#43436,#43437,#43438,#43439,#43440,
#43441,#43442,#43443,#43444,#43445,#43446,#43447,#43448,#43449,#43450,#43451,
#43452,#43453,#43454,#43455,#43456,#43457,#43458,#43459,#43460,#43461,#43462,
#43463,#43464,#43465,#43466,#43467,#43468,#43469,#43470,#43471,#43472,#43473,
#43474,#43475,#43476,#43477,#43478,#43479,#43480,#43481,#43482,#43483,#43484,
#43485,#43486,#43487,#43488,#43489,#43490,#43491,#43492,#43493,#43494,#43495,
#43496,#43497,#43498,#43499,#43500,#43501,#43502,#43503,#43504,#43505,#43506,
#43507,#43508,#43509,#43510,#43511,#43512,#43513,#43514,#43515,#43516,#43517,
#43518,#43519,#43520,#43521,#43522),.UNSPECIFIED.,.F.,.F.,(4,2,2,2,2,2,
2,2,2,2,2,2,2,2,2,2,2,2,2,2,2,2,2,2,2,2,2,2,2,2,2,2,2,2,2,2,2,2,2,2,2,2,
2,2,2,2,2,2,2,2,2,2,2,2,2,2,2,2,2,2,2,2,2,2,2,2,2,2,2,2,4),(-1.26096989666227,
-1.22707058127239,-1.21883665098304,-1.21289954999642,-1.20452617599143,
-1.17050362623785,-1.13505788761883,-1.12240658005665,-1.11212247487635,
-1.09914117067393,-1.05877205797667,-1.03006717083556,-1.02178707012923,
-1.01585312011901,-1.00753612548882,-0.972574059078231,-0.937995783116275,
-0.925203432258212,-0.914816294073501,-0.901684245354329,-0.86289631062092,
-0.83290071502599,-0.82478680774899,-0.818805855652598,-0.810142260707499,
-0.786096075401545,-0.755904654055759,-0.73597095185452,-0.724797129082856,
-0.714207929993758,-0.697763307221352,-0.65614157148257,-0.641239193444398,
-0.630465011268126,-0.62487137855747,-0.618203007845375,-0.604447950817056,
-0.582238896381285,-0.545920399853265,-0.532768230208396,-0.522410230839679,
-0.509928389110634,-0.472994950077797,-0.439951546199994,-0.431462167963196,
-0.425506067265656,-0.417314381788017,-0.388017161369834,-0.348366600927986,
-0.335298804060168,-0.324936578735646,-0.312152912192802,-0.297732041447513,
-0.267499207795241,-0.243457877537951,-0.234795503786561,-0.22882907817729,
-0.220770488928708,-0.19100223684165,-0.151594040354065,-0.138510634584796,
-0.128153541750447,-0.115399159575225,-0.101026582114009,-0.0710352414085446,
-0.0446772738205007,-0.0369488222373959,-0.0309729674374409,-0.0248730602270775,
-0.0160319166381245,-2.50941038643732E-5),.UNSPECIFIED.);
#486=B_SPLINE_CURVE_WITH_KNOTS('',3,(#43593,#43594,#43595,#43596,#43597,
#43598,#43599,#43600,#43601,#43602,#43603,#43604,#43605,#43606,#43607,#43608),
 .UNSPECIFIED.,.F.,.F.,(4,2,2,2,2,2,2,4),(0.500000149075164,0.571383311424569,
0.625,0.714192063098084,0.75,0.857080176928947,0.875,1.),.UNSPECIFIED.);
#487=B_SPLINE_CURVE_WITH_KNOTS('',3,(#43838,#43839,#43840,#43841,#43842,
#43843,#43844),.UNSPECIFIED.,.F.,.F.,(4,1,1,1,4),(-1.,-0.785714285714286,
-0.571428571428571,-0.285714285714286,3.18349790973116E-11),
 .UNSPECIFIED.);
#488=B_SPLINE_CURVE_WITH_KNOTS('',3,(#43883,#43884,#43885,#43886,#43887,
#43888),.UNSPECIFIED.,.F.,.F.,(4,2,4),(0.000117088579411485,0.000909402471215065,
0.00174490984546788),.UNSPECIFIED.);
#489=B_SPLINE_CURVE_WITH_KNOTS('',3,(#43890,#43891,#43892,#43893,#43894,
#43895,#43896,#43897,#43898,#43899,#43900,#43901,#43902,#43903,#43904,#43905,
#43906,#43907,#43908,#43909,#43910,#43911,#43912,#43913,#43914,#43915,#43916,
#43917,#43918,#43919,#43920,#43921,#43922,#43923,#43924,#43925,#43926,#43927,
#43928,#43929,#43930,#43931,#43932,#43933,#43934,#43935),.UNSPECIFIED.,
 .F.,.F.,(4,3,3,3,3,3,3,3,3,3,3,3,3,3,3,4),(-0.409631076264667,-0.385380122364829,
-0.3409735646143,-0.331279738066214,-0.326505129564108,-0.260525143680311,
-0.251715173498639,-0.247659301762696,-0.223884696358354,-0.211563155315766,
-0.163804628915719,-0.160094298147174,-0.0805484267240998,-0.0768764939308757,
-0.0110461773969077,0.),.UNSPECIFIED.);
#490=B_SPLINE_CURVE_WITH_KNOTS('',3,(#43936,#43937,#43938,#43939,#43940,
#43941,#43942,#43943,#43944,#43945,#43946,#43947,#43948,#43949,#43950,#43951,
#43952,#43953,#43954,#43955,#43956,#43957,#43958,#43959,#43960,#43961,#43962,
#43963,#43964,#43965,#43966,#43967,#43968,#43969,#43970,#43971,#43972,#43973,
#43974,#43975,#43976,#43977,#43978,#43979,#43980,#43981,#43982,#43983,#43984,
#43985,#43986,#43987,#43988,#43989,#43990),.UNSPECIFIED.,.F.,.F.,(4,3,3,
3,3,3,3,3,3,3,3,3,3,3,3,3,3,3,4),(-0.413257902153422,-0.390922947181097,
-0.368527860933955,-0.351784161114064,-0.345070111406328,-0.3408068417481,
-0.279278028382547,-0.273184383320329,-0.269298985732011,-0.245026600124572,
-0.234578262374825,-0.197920862117467,-0.187270004319717,-0.183437118834528,
-0.0991669299111112,-0.0951172833893305,-0.0912706016525077,-0.0138375730600328,
0.),.UNSPECIFIED.);
#491=B_SPLINE_CURVE_WITH_KNOTS('',3,(#44159,#44160,#44161,#44162,#44163,
#44164,#44165,#44166,#44167,#44168,#44169,#44170,#44171,#44172,#44173,#44174,
#44175,#44176,#44177,#44178,#44179,#44180,#44181,#44182,#44183,#44184,#44185,
#44186,#44187,#44188,#44189,#44190,#44191,#44192,#44193,#44194,#44195,#44196,
#44197,#44198,#44199,#44200,#44201,#44202,#44203,#44204,#44205,#44206,#44207),
 .UNSPECIFIED.,.F.,.F.,(4,3,3,3,3,3,3,3,3,3,3,3,3,3,3,3,4),(-0.41325790215343,
-0.351784145825427,-0.345070539488157,-0.340806885032473,-0.279278049754355,
-0.273184457928296,-0.269298995380588,-0.245026610762357,-0.234578262374832,
-0.187269997389303,-0.183437116025571,-0.109052973926965,-0.0991668215785101,
-0.0951172236224628,-0.0912705901101731,-0.0138375948482117,0.),
 .UNSPECIFIED.);
#492=B_SPLINE_CURVE_WITH_KNOTS('',3,(#44209,#44210,#44211,#44212,#44213,
#44214,#44215,#44216,#44217,#44218,#44219,#44220,#44221,#44222,#44223,#44224,
#44225,#44226,#44227,#44228,#44229,#44230,#44231,#44232,#44233,#44234,#44235,
#44236,#44237,#44238,#44239,#44240,#44241,#44242,#44243,#44244,#44245,#44246,
#44247,#44248,#44249,#44250,#44251,#44252,#44253,#44254,#44255,#44256,#44257),
 .UNSPECIFIED.,.F.,.F.,(4,3,3,3,3,3,3,3,3,3,3,3,3,3,3,3,4),(-0.409631140621061,
-0.385380121304351,-0.340973570999351,-0.326505126071581,-0.260525176777292,
-0.251715206634708,-0.247659319036372,-0.223884748477094,-0.211563155315756,
-0.163804641724133,-0.160094308683559,-0.136551760510434,-0.113090562557914,
-0.0805484427544219,-0.0768765013185619,-0.0110460447264667,0.),
 .UNSPECIFIED.);
#647=CONICAL_SURFACE('',#10696,0.00125,0.643501108793284);
#648=CONICAL_SURFACE('',#10727,0.00075,1.43824479449822);
#649=CONICAL_SURFACE('',#10728,0.00075,1.43824479449822);
#650=CONICAL_SURFACE('',#10729,0.00075,1.43824479449822);
#651=CONICAL_SURFACE('',#10730,0.0006,0.321750554396642);
#652=CONICAL_SURFACE('',#10736,0.0012,0.674740942223553);
#653=CONICAL_SURFACE('',#10742,0.0024,0.785398163397448);
#753=FACE_BOUND('',#2016,.T.);
#754=FACE_BOUND('',#2020,.T.);
#755=FACE_BOUND('',#2023,.T.);
#756=FACE_BOUND('',#2031,.T.);
#757=FACE_BOUND('',#2037,.T.);
#758=FACE_BOUND('',#2055,.T.);
#759=FACE_BOUND('',#2063,.T.);
#793=SHAPE_REPRESENTATION_RELATIONSHIP('SRR','None',#50161,#813);
#813=ADVANCED_BREP_SHAPE_REPRESENTATION('',(#853),#50074);
#833=STYLED_ITEM('',(#50259),#853);
#853=MANIFOLD_SOLID_BREP('Body1',#9878);
#1008=PLANE('',#10695);
#1009=PLANE('',#10698);
#1010=PLANE('',#10699);
#1011=PLANE('',#10701);
#1012=PLANE('',#10702);
#1013=PLANE('',#10704);
#1014=PLANE('',#10705);
#1015=PLANE('',#10706);
#1016=PLANE('',#10707);
#1017=PLANE('',#10708);
#1018=PLANE('',#10709);
#1019=PLANE('',#10710);
#1020=PLANE('',#10712);
#1021=PLANE('',#10713);
#1022=PLANE('',#10714);
#1023=PLANE('',#10715);
#1024=PLANE('',#10716);
#1025=PLANE('',#10718);
#1026=PLANE('',#10719);
#1027=PLANE('',#10720);
#1028=PLANE('',#10721);
#1029=PLANE('',#10722);
#1030=PLANE('',#10723);
#1031=PLANE('',#10724);
#1032=PLANE('',#10725);
#1033=PLANE('',#10726);
#1034=PLANE('',#10739);
#1035=PLANE('',#10745);
#1036=PLANE('',#10746);
#1037=PLANE('',#10747);
#1421=FACE_OUTER_BOUND('',#2005,.T.);
#1422=FACE_OUTER_BOUND('',#2006,.T.);
#1423=FACE_OUTER_BOUND('',#2007,.T.);
#1424=FACE_OUTER_BOUND('',#2008,.T.);
#1425=FACE_OUTER_BOUND('',#2009,.T.);
#1426=FACE_OUTER_BOUND('',#2010,.T.);
#1427=FACE_OUTER_BOUND('',#2011,.T.);
#1428=FACE_OUTER_BOUND('',#2012,.T.);
#1429=FACE_OUTER_BOUND('',#2013,.T.);
#1430=FACE_OUTER_BOUND('',#2014,.T.);
#1431=FACE_OUTER_BOUND('',#2015,.T.);
#1432=FACE_OUTER_BOUND('',#2017,.T.);
#1433=FACE_OUTER_BOUND('',#2018,.T.);
#1434=FACE_OUTER_BOUND('',#2019,.T.);
#1435=FACE_OUTER_BOUND('',#2021,.T.);
#1436=FACE_OUTER_BOUND('',#2022,.T.);
#1437=FACE_OUTER_BOUND('',#2024,.T.);
#1438=FACE_OUTER_BOUND('',#2025,.T.);
#1439=FACE_OUTER_BOUND('',#2026,.T.);
#1440=FACE_OUTER_BOUND('',#2027,.T.);
#1441=FACE_OUTER_BOUND('',#2028,.T.);
#1442=FACE_OUTER_BOUND('',#2029,.T.);
#1443=FACE_OUTER_BOUND('',#2030,.T.);
#1444=FACE_OUTER_BOUND('',#2032,.T.);
#1445=FACE_OUTER_BOUND('',#2033,.T.);
#1446=FACE_OUTER_BOUND('',#2034,.T.);
#1447=FACE_OUTER_BOUND('',#2035,.T.);
#1448=FACE_OUTER_BOUND('',#2036,.T.);
#1449=FACE_OUTER_BOUND('',#2038,.T.);
#1450=FACE_OUTER_BOUND('',#2039,.T.);
#1451=FACE_OUTER_BOUND('',#2040,.T.);
#1452=FACE_OUTER_BOUND('',#2041,.T.);
#1453=FACE_OUTER_BOUND('',#2042,.T.);
#1454=FACE_OUTER_BOUND('',#2043,.T.);
#1455=FACE_OUTER_BOUND('',#2044,.T.);
#1456=FACE_OUTER_BOUND('',#2045,.T.);
#1457=FACE_OUTER_BOUND('',#2046,.T.);
#1458=FACE_OUTER_BOUND('',#2047,.T.);
#1459=FACE_OUTER_BOUND('',#2048,.T.);
#1460=FACE_OUTER_BOUND('',#2049,.T.);
#1461=FACE_OUTER_BOUND('',#2050,.T.);
#1462=FACE_OUTER_BOUND('',#2051,.T.);
#1463=FACE_OUTER_BOUND('',#2052,.T.);
#1464=FACE_OUTER_BOUND('',#2053,.T.);
#1465=FACE_OUTER_BOUND('',#2054,.T.);
#1466=FACE_OUTER_BOUND('',#2056,.T.);
#1467=FACE_OUTER_BOUND('',#2057,.T.);
#1468=FACE_OUTER_BOUND('',#2058,.T.);
#1469=FACE_OUTER_BOUND('',#2059,.T.);
#1470=FACE_OUTER_BOUND('',#2060,.T.);
#1471=FACE_OUTER_BOUND('',#2061,.T.);
#1472=FACE_OUTER_BOUND('',#2062,.T.);
#2005=EDGE_LOOP('',(#7988,#7989,#7990,#7991));
#2006=EDGE_LOOP('',(#7992,#7993,#7994,#7995,#7996));
#2007=EDGE_LOOP('',(#7997,#7998,#7999,#8000));
#2008=EDGE_LOOP('',(#8001,#8002,#8003,#8004));
#2009=EDGE_LOOP('',(#8005,#8006,#8007,#8008));
#2010=EDGE_LOOP('',(#8009,#8010,#8011,#8012,#8013,#8014,#8015,#8016));
#2011=EDGE_LOOP('',(#8017,#8018,#8019,#8020));
#2012=EDGE_LOOP('',(#8021,#8022,#8023,#8024));
#2013=EDGE_LOOP('',(#8025,#8026,#8027,#8028,#8029,#8030,#8031,#8032,#8033,
#8034,#8035,#8036));
#2014=EDGE_LOOP('',(#8037,#8038,#8039,#8040));
#2015=EDGE_LOOP('',(#8041,#8042,#8043,#8044,#8045,#8046,#8047,#8048,#8049,
#8050,#8051,#8052));
#2016=EDGE_LOOP('',(#8053,#8054));
#2017=EDGE_LOOP('',(#8055,#8056,#8057,#8058,#8059));
#2018=EDGE_LOOP('',(#8060,#8061,#8062,#8063));
#2019=EDGE_LOOP('',(#8064,#8065,#8066,#8067,#8068,#8069,#8070,#8071));
#2020=EDGE_LOOP('',(#8072));
#2021=EDGE_LOOP('',(#8073,#8074,#8075,#8076));
#2022=EDGE_LOOP('',(#8077,#8078,#8079,#8080,#8081,#8082,#8083,#8084));
#2023=EDGE_LOOP('',(#8085));
#2024=EDGE_LOOP('',(#8086,#8087,#8088,#8089));
#2025=EDGE_LOOP('',(#8090,#8091,#8092,#8093));
#2026=EDGE_LOOP('',(#8094,#8095,#8096,#8097,#8098,#8099,#8100,#8101));
#2027=EDGE_LOOP('',(#8102,#8103,#8104,#8105));
#2028=EDGE_LOOP('',(#8106,#8107,#8108,#8109));
#2029=EDGE_LOOP('',(#8110,#8111,#8112,#8113));
#2030=EDGE_LOOP('',(#8114,#8115,#8116,#8117,#8118,#8119,#8120,#8121,#8122,
#8123,#8124,#8125));
#2031=EDGE_LOOP('',(#8126));
#2032=EDGE_LOOP('',(#8127,#8128,#8129,#8130));
#2033=EDGE_LOOP('',(#8131,#8132,#8133,#8134));
#2034=EDGE_LOOP('',(#8135,#8136,#8137,#8138));
#2035=EDGE_LOOP('',(#8139,#8140,#8141,#8142));
#2036=EDGE_LOOP('',(#8143,#8144,#8145,#8146,#8147,#8148,#8149,#8150));
#2037=EDGE_LOOP('',(#8151));
#2038=EDGE_LOOP('',(#8152,#8153,#8154,#8155));
#2039=EDGE_LOOP('',(#8156,#8157,#8158,#8159));
#2040=EDGE_LOOP('',(#8160,#8161,#8162,#8163,#8164,#8165,#8166,#8167));
#2041=EDGE_LOOP('',(#8168,#8169,#8170,#8171));
#2042=EDGE_LOOP('',(#8172,#8173,#8174,#8175));
#2043=EDGE_LOOP('',(#8176,#8177,#8178,#8179,#8180,#8181,#8182,#8183));
#2044=EDGE_LOOP('',(#8184,#8185,#8186,#8187));
#2045=EDGE_LOOP('',(#8188,#8189,#8190,#8191));
#2046=EDGE_LOOP('',(#8192,#8193,#8194,#8195));
#2047=EDGE_LOOP('',(#8196,#8197,#8198,#8199));
#2048=EDGE_LOOP('',(#8200,#8201,#8202));
#2049=EDGE_LOOP('',(#8203,#8204,#8205));
#2050=EDGE_LOOP('',(#8206,#8207,#8208));
#2051=EDGE_LOOP('',(#8209,#8210,#8211,#8212,#8213));
#2052=EDGE_LOOP('',(#8214,#8215,#8216,#8217));
#2053=EDGE_LOOP('',(#8218,#8219,#8220,#8221));
#2054=EDGE_LOOP('',(#8222));
#2055=EDGE_LOOP('',(#8223));
#2056=EDGE_LOOP('',(#8224,#8225,#8226,#8227,#8228));
#2057=EDGE_LOOP('',(#8229,#8230,#8231,#8232,#8233,#8234,#8235));
#2058=EDGE_LOOP('',(#8236,#8237,#8238,#8239,#8240));
#2059=EDGE_LOOP('',(#8241,#8242,#8243,#8244,#8245,#8246,#8247,#8248,#8249,
#8250,#8251,#8252,#8253,#8254,#8255));
#2060=EDGE_LOOP('',(#8256,#8257,#8258,#8259,#8260));
#2061=EDGE_LOOP('',(#8261,#8262,#8263,#8264,#8265,#8266,#8267,#8268,#8269,
#8270,#8271,#8272,#8273,#8274,#8275));
#2062=EDGE_LOOP('',(#8276));
#2063=EDGE_LOOP('',(#8277));
#2536=LINE('',#40495,#3114);
#2537=LINE('',#40582,#3115);
#2538=LINE('',#40905,#3116);
#2539=LINE('',#41223,#3117);
#2540=LINE('',#41543,#3118);
#2541=LINE('',#41891,#3119);
#2542=LINE('',#41921,#3120);
#2543=LINE('',#43613,#3121);
#2544=LINE('',#43615,#3122);
#2545=LINE('',#43617,#3123);
#2546=LINE('',#43619,#3124);
#2547=LINE('',#43621,#3125);
#2548=LINE('',#43623,#3126);
#2549=LINE('',#43625,#3127);
#2550=LINE('',#43627,#3128);
#2551=LINE('',#43629,#3129);
#2552=LINE('',#43631,#3130);
#2553=LINE('',#43633,#3131);
#2554=LINE('',#43634,#3132);
#2555=LINE('',#43637,#3133);
#2556=LINE('',#43641,#3134);
#2557=LINE('',#43643,#3135);
#2558=LINE('',#43644,#3136);
#2559=LINE('',#43647,#3137);
#2560=LINE('',#43649,#3138);
#2561=LINE('',#43651,#3139);
#2562=LINE('',#43653,#3140);
#2563=LINE('',#43655,#3141);
#2564=LINE('',#43656,#3142);
#2565=LINE('',#43661,#3143);
#2566=LINE('',#43663,#3144);
#2567=LINE('',#43664,#3145);
#2568=LINE('',#43667,#3146);
#2569=LINE('',#43669,#3147);
#2570=LINE('',#43671,#3148);
#2571=LINE('',#43673,#3149);
#2572=LINE('',#43675,#3150);
#2573=LINE('',#43676,#3151);
#2574=LINE('',#43681,#3152);
#2575=LINE('',#43682,#3153);
#2576=LINE('',#43685,#3154);
#2577=LINE('',#43687,#3155);
#2578=LINE('',#43688,#3156);
#2579=LINE('',#43691,#3157);
#2580=LINE('',#43693,#3158);
#2581=LINE('',#43695,#3159);
#2582=LINE('',#43697,#3160);
#2583=LINE('',#43699,#3161);
#2584=LINE('',#43700,#3162);
#2585=LINE('',#43703,#3163);
#2586=LINE('',#43704,#3164);
#2587=LINE('',#43707,#3165);
#2588=LINE('',#43708,#3166);
#2589=LINE('',#43711,#3167);
#2590=LINE('',#43713,#3168);
#2591=LINE('',#43714,#3169);
#2592=LINE('',#43717,#3170);
#2593=LINE('',#43718,#3171);
#2594=LINE('',#43720,#3172);
#2595=LINE('',#43722,#3173);
#2596=LINE('',#43723,#3174);
#2597=LINE('',#43725,#3175);
#2598=LINE('',#43727,#3176);
#2599=LINE('',#43728,#3177);
#2600=LINE('',#43733,#3178);
#2601=LINE('',#43734,#3179);
#2602=LINE('',#43737,#3180);
#2603=LINE('',#43738,#3181);
#2604=LINE('',#43741,#3182);
#2605=LINE('',#43742,#3183);
#2606=LINE('',#43745,#3184);
#2607=LINE('',#43746,#3185);
#2608=LINE('',#43749,#3186);
#2609=LINE('',#43750,#3187);
#2610=LINE('',#43751,#3188);
#2611=LINE('',#43756,#3189);
#2612=LINE('',#43758,#3190);
#2613=LINE('',#43761,#3191);
#2614=LINE('',#43763,#3192);
#2615=LINE('',#43766,#3193);
#2616=LINE('',#43847,#3194);
#2617=LINE('',#43850,#3195);
#2618=LINE('',#43853,#3196);
#2619=LINE('',#43858,#3197);
#2620=LINE('',#43865,#3198);
#2621=LINE('',#43870,#3199);
#2622=LINE('',#43876,#3200);
#2623=LINE('',#43881,#3201);
#3114=VECTOR('',#12478,0.0025);
#3115=VECTOR('',#12483,0.0025);
#3116=VECTOR('',#12486,0.0025);
#3117=VECTOR('',#12489,0.0025);
#3118=VECTOR('',#12492,0.0025);
#3119=VECTOR('',#12495,0.0025);
#3120=VECTOR('',#12498,0.0025);
#3121=VECTOR('',#12515,1.);
#3122=VECTOR('',#12516,1.);
#3123=VECTOR('',#12517,1.);
#3124=VECTOR('',#12518,1.);
#3125=VECTOR('',#12519,1.);
#3126=VECTOR('',#12520,1.);
#3127=VECTOR('',#12521,1.);
#3128=VECTOR('',#12522,1.);
#3129=VECTOR('',#12523,1.);
#3130=VECTOR('',#12524,1.);
#3131=VECTOR('',#12525,1.);
#3132=VECTOR('',#12526,1.);
#3133=VECTOR('',#12529,0.00125);
#3134=VECTOR('',#12534,1.);
#3135=VECTOR('',#12535,1.);
#3136=VECTOR('',#12536,1.);
#3137=VECTOR('',#12539,1.);
#3138=VECTOR('',#12540,1.);
#3139=VECTOR('',#12541,1.);
#3140=VECTOR('',#12542,1.);
#3141=VECTOR('',#12543,1.);
#3142=VECTOR('',#12544,1.);
#3143=VECTOR('',#12549,1.);
#3144=VECTOR('',#12550,1.);
#3145=VECTOR('',#12551,1.);
#3146=VECTOR('',#12554,1.);
#3147=VECTOR('',#12555,1.);
#3148=VECTOR('',#12556,1.);
#3149=VECTOR('',#12557,1.);
#3150=VECTOR('',#12558,1.);
#3151=VECTOR('',#12559,1.);
#3152=VECTOR('',#12564,1.);
#3153=VECTOR('',#12565,1.);
#3154=VECTOR('',#12568,1.);
#3155=VECTOR('',#12569,1.);
#3156=VECTOR('',#12570,1.);
#3157=VECTOR('',#12573,1.);
#3158=VECTOR('',#12574,1.);
#3159=VECTOR('',#12575,1.);
#3160=VECTOR('',#12576,1.);
#3161=VECTOR('',#12577,1.);
#3162=VECTOR('',#12578,1.);
#3163=VECTOR('',#12581,1.);
#3164=VECTOR('',#12582,1.);
#3165=VECTOR('',#12585,1.);
#3166=VECTOR('',#12586,1.);
#3167=VECTOR('',#12589,1.);
#3168=VECTOR('',#12590,1.);
#3169=VECTOR('',#12591,1.);
#3170=VECTOR('',#12594,1.);
#3171=VECTOR('',#12595,1.);
#3172=VECTOR('',#12596,1.);
#3173=VECTOR('',#12597,1.);
#3174=VECTOR('',#12598,1.);
#3175=VECTOR('',#12599,1.);
#3176=VECTOR('',#12600,1.);
#3177=VECTOR('',#12601,1.);
#3178=VECTOR('',#12606,1.);
#3179=VECTOR('',#12607,1.);
#3180=VECTOR('',#12610,1.);
#3181=VECTOR('',#12611,1.);
#3182=VECTOR('',#12614,1.);
#3183=VECTOR('',#12615,1.);
#3184=VECTOR('',#12618,1.);
#3185=VECTOR('',#12619,1.);
#3186=VECTOR('',#12622,1.);
#3187=VECTOR('',#12623,1.);
#3188=VECTOR('',#12624,1.);
#3189=VECTOR('',#12631,1.);
#3190=VECTOR('',#12634,1.);
#3191=VECTOR('',#12639,1.);
#3192=VECTOR('',#12642,1.);
#3193=VECTOR('',#12647,1.);
#3194=VECTOR('',#12652,0.00075);
#3195=VECTOR('',#12655,0.00075);
#3196=VECTOR('',#12658,0.00075);
#3197=VECTOR('',#12663,0.0006);
#3198=VECTOR('',#12672,0.0002);
#3199=VECTOR('',#12677,0.0012);
#3200=VECTOR('',#12686,0.001);
#3201=VECTOR('',#12691,0.0024);
#3632=CIRCLE('',#10681,0.00250000000001);
#3633=CIRCLE('',#10687,0.00250000000001);
#3634=CIRCLE('',#10688,0.00250000000001);
#3635=CIRCLE('',#10689,0.00215000000001);
#3636=CIRCLE('',#10692,0.00200000000001);
#3637=CIRCLE('',#10693,0.00200000000001);
#3638=CIRCLE('',#10694,0.00215000000001);
#3639=CIRCLE('',#10697,0.00050000000001);
#3640=CIRCLE('',#10700,0.00075000000001366);
#3641=CIRCLE('',#10703,0.00075000000001);
#3642=CIRCLE('',#10711,0.00270000000001);
#3643=CIRCLE('',#10717,0.00075000000001366);
#3644=CIRCLE('',#10731,0.00020000000001);
#3645=CIRCLE('',#10732,0.00100000000001);
#3646=CIRCLE('',#10733,0.00100000000001);
#3647=CIRCLE('',#10735,0.00020000000001);
#3648=CIRCLE('',#10737,0.00100000000001);
#3649=CIRCLE('',#10738,0.00140000000001);
#3650=CIRCLE('',#10740,0.00230000000001);
#3651=CIRCLE('',#10743,0.00250000000001);
#3652=CIRCLE('',#10744,0.00250000000001);
#4387=VERTEX_POINT('',#40493);
#4388=VERTEX_POINT('',#40494);
#4389=VERTEX_POINT('',#40496);
#4390=VERTEX_POINT('',#40547);
#4391=VERTEX_POINT('',#40580);
#4392=VERTEX_POINT('',#40581);
#4393=VERTEX_POINT('',#40583);
#4394=VERTEX_POINT('',#40903);
#4395=VERTEX_POINT('',#40904);
#4396=VERTEX_POINT('',#41221);
#4397=VERTEX_POINT('',#41222);
#4398=VERTEX_POINT('',#41541);
#4399=VERTEX_POINT('',#41542);
#4400=VERTEX_POINT('',#41859);
#4401=VERTEX_POINT('',#41890);
#4402=VERTEX_POINT('',#41892);
#4403=VERTEX_POINT('',#41894);
#4404=VERTEX_POINT('',#41920);
#4405=VERTEX_POINT('',#41922);
#4406=VERTEX_POINT('',#42094);
#4407=VERTEX_POINT('',#42095);
#4408=VERTEX_POINT('',#42103);
#4409=VERTEX_POINT('',#42105);
#4410=VERTEX_POINT('',#42455);
#4411=VERTEX_POINT('',#42456);
#4412=VERTEX_POINT('',#43013);
#4413=VERTEX_POINT('',#43027);
#4414=VERTEX_POINT('',#43029);
#4415=VERTEX_POINT('',#43094);
#4416=VERTEX_POINT('',#43144);
#4417=VERTEX_POINT('',#43194);
#4418=VERTEX_POINT('',#43244);
#4419=VERTEX_POINT('',#43294);
#4420=VERTEX_POINT('',#43344);
#4421=VERTEX_POINT('',#43346);
#4422=VERTEX_POINT('',#43611);
#4423=VERTEX_POINT('',#43612);
#4424=VERTEX_POINT('',#43614);
#4425=VERTEX_POINT('',#43616);
#4426=VERTEX_POINT('',#43618);
#4427=VERTEX_POINT('',#43620);
#4428=VERTEX_POINT('',#43622);
#4429=VERTEX_POINT('',#43624);
#4430=VERTEX_POINT('',#43626);
#4431=VERTEX_POINT('',#43628);
#4432=VERTEX_POINT('',#43630);
#4433=VERTEX_POINT('',#43632);
#4434=VERTEX_POINT('',#43636);
#4435=VERTEX_POINT('',#43640);
#4436=VERTEX_POINT('',#43642);
#4437=VERTEX_POINT('',#43646);
#4438=VERTEX_POINT('',#43648);
#4439=VERTEX_POINT('',#43650);
#4440=VERTEX_POINT('',#43652);
#4441=VERTEX_POINT('',#43654);
#4442=VERTEX_POINT('',#43657);
#4443=VERTEX_POINT('',#43660);
#4444=VERTEX_POINT('',#43662);
#4445=VERTEX_POINT('',#43666);
#4446=VERTEX_POINT('',#43668);
#4447=VERTEX_POINT('',#43670);
#4448=VERTEX_POINT('',#43672);
#4449=VERTEX_POINT('',#43674);
#4450=VERTEX_POINT('',#43677);
#4451=VERTEX_POINT('',#43680);
#4452=VERTEX_POINT('',#43684);
#4453=VERTEX_POINT('',#43686);
#4454=VERTEX_POINT('',#43690);
#4455=VERTEX_POINT('',#43692);
#4456=VERTEX_POINT('',#43694);
#4457=VERTEX_POINT('',#43696);
#4458=VERTEX_POINT('',#43698);
#4459=VERTEX_POINT('',#43702);
#4460=VERTEX_POINT('',#43706);
#4461=VERTEX_POINT('',#43710);
#4462=VERTEX_POINT('',#43712);
#4463=VERTEX_POINT('',#43716);
#4464=VERTEX_POINT('',#43719);
#4465=VERTEX_POINT('',#43721);
#4466=VERTEX_POINT('',#43724);
#4467=VERTEX_POINT('',#43726);
#4468=VERTEX_POINT('',#43729);
#4469=VERTEX_POINT('',#43732);
#4470=VERTEX_POINT('',#43736);
#4471=VERTEX_POINT('',#43740);
#4472=VERTEX_POINT('',#43744);
#4473=VERTEX_POINT('',#43748);
#4474=VERTEX_POINT('',#43752);
#4475=VERTEX_POINT('',#43846);
#4476=VERTEX_POINT('',#43849);
#4477=VERTEX_POINT('',#43852);
#4478=VERTEX_POINT('',#43855);
#4479=VERTEX_POINT('',#43857);
#4480=VERTEX_POINT('',#43859);
#4481=VERTEX_POINT('',#43863);
#4482=VERTEX_POINT('',#43867);
#4483=VERTEX_POINT('',#43869);
#4484=VERTEX_POINT('',#43873);
#4485=VERTEX_POINT('',#43878);
#4486=VERTEX_POINT('',#43879);
#5647=EDGE_CURVE('',#4387,#4388,#2536,.T.);
#5648=EDGE_CURVE('',#4387,#4389,#457,.T.);
#5649=EDGE_CURVE('',#4390,#4389,#3632,.T.);
#5650=EDGE_CURVE('',#4390,#4388,#458,.T.);
#5651=EDGE_CURVE('',#4391,#4392,#2537,.T.);
#5652=EDGE_CURVE('',#4391,#4393,#459,.T.);
#5653=EDGE_CURVE('',#4393,#4387,#460,.T.);
#5654=EDGE_CURVE('',#4388,#4392,#461,.T.);
#5655=EDGE_CURVE('',#4394,#4395,#2538,.T.);
#5656=EDGE_CURVE('',#4394,#4391,#462,.T.);
#5657=EDGE_CURVE('',#4392,#4395,#463,.T.);
#5658=EDGE_CURVE('',#4396,#4397,#2539,.T.);
#5659=EDGE_CURVE('',#4396,#4394,#464,.T.);
#5660=EDGE_CURVE('',#4395,#4397,#465,.T.);
#5661=EDGE_CURVE('',#4398,#4399,#2540,.T.);
#5662=EDGE_CURVE('',#4398,#4396,#466,.T.);
#5663=EDGE_CURVE('',#4397,#4399,#467,.T.);
#5664=EDGE_CURVE('',#4400,#4400,#468,.F.);
#5665=EDGE_CURVE('',#4400,#4401,#2541,.T.);
#5666=EDGE_CURVE('',#4401,#4402,#3633,.T.);
#5667=EDGE_CURVE('',#4402,#4403,#469,.T.);
#5668=EDGE_CURVE('',#4403,#4404,#2542,.T.);
#5669=EDGE_CURVE('',#4404,#4405,#470,.T.);
#5670=EDGE_CURVE('',#4405,#4401,#3634,.T.);
#5671=EDGE_CURVE('',#4406,#4407,#471,.T.);
#5672=EDGE_CURVE('',#4406,#4408,#3635,.T.);
#5673=EDGE_CURVE('',#4408,#4409,#472,.T.);
#5674=EDGE_CURVE('',#4409,#4407,#473,.F.);
#5675=EDGE_CURVE('',#4403,#4398,#474,.T.);
#5676=EDGE_CURVE('',#4399,#4404,#475,.T.);
#5677=EDGE_CURVE('',#4410,#4411,#476,.T.);
#5678=EDGE_CURVE('',#4411,#4412,#477,.T.);
#5679=EDGE_CURVE('',#4413,#4412,#3636,.T.);
#5680=EDGE_CURVE('',#4414,#4413,#478,.F.);
#5681=EDGE_CURVE('',#4415,#4414,#479,.F.);
#5682=EDGE_CURVE('',#4416,#4415,#480,.F.);
#5683=EDGE_CURVE('',#4417,#4416,#481,.F.);
#5684=EDGE_CURVE('',#4418,#4417,#482,.F.);
#5685=EDGE_CURVE('',#4419,#4418,#483,.F.);
#5686=EDGE_CURVE('',#4420,#4419,#3637,.T.);
#5687=EDGE_CURVE('',#4420,#4421,#484,.T.);
#5688=EDGE_CURVE('',#4421,#4410,#485,.T.);
#5689=EDGE_CURVE('',#4407,#4409,#486,.F.);
#5690=EDGE_CURVE('',#4408,#4406,#3638,.T.);
#5691=EDGE_CURVE('',#4422,#4423,#2543,.T.);
#5692=EDGE_CURVE('',#4422,#4424,#2544,.T.);
#5693=EDGE_CURVE('',#4425,#4424,#2545,.T.);
#5694=EDGE_CURVE('',#4425,#4426,#2546,.T.);
#5695=EDGE_CURVE('',#4427,#4426,#2547,.T.);
#5696=EDGE_CURVE('',#4427,#4428,#2548,.T.);
#5697=EDGE_CURVE('',#4429,#4428,#2549,.T.);
#5698=EDGE_CURVE('',#4429,#4430,#2550,.T.);
#5699=EDGE_CURVE('',#4431,#4430,#2551,.T.);
#5700=EDGE_CURVE('',#4431,#4432,#2552,.T.);
#5701=EDGE_CURVE('',#4433,#4432,#2553,.T.);
#5702=EDGE_CURVE('',#4433,#4423,#2554,.T.);
#5703=EDGE_CURVE('',#4407,#4434,#2555,.T.);
#5704=EDGE_CURVE('',#4434,#4434,#3639,.T.);
#5705=EDGE_CURVE('',#4423,#4435,#2556,.T.);
#5706=EDGE_CURVE('',#4435,#4436,#2557,.T.);
#5707=EDGE_CURVE('',#4436,#4422,#2558,.T.);
#5708=EDGE_CURVE('',#4437,#4433,#2559,.T.);
#5709=EDGE_CURVE('',#4438,#4437,#2560,.T.);
#5710=EDGE_CURVE('',#4439,#4438,#2561,.T.);
#5711=EDGE_CURVE('',#4439,#4440,#2562,.T.);
#5712=EDGE_CURVE('',#4441,#4440,#2563,.T.);
#5713=EDGE_CURVE('',#4435,#4441,#2564,.T.);
#5714=EDGE_CURVE('',#4442,#4442,#3640,.T.);
#5715=EDGE_CURVE('',#4424,#4443,#2565,.T.);
#5716=EDGE_CURVE('',#4443,#4444,#2566,.T.);
#5717=EDGE_CURVE('',#4444,#4425,#2567,.T.);
#5718=EDGE_CURVE('',#4445,#4444,#2568,.T.);
#5719=EDGE_CURVE('',#4446,#4445,#2569,.T.);
#5720=EDGE_CURVE('',#4446,#4447,#2570,.T.);
#5721=EDGE_CURVE('',#4448,#4447,#2571,.T.);
#5722=EDGE_CURVE('',#4449,#4448,#2572,.T.);
#5723=EDGE_CURVE('',#4426,#4449,#2573,.T.);
#5724=EDGE_CURVE('',#4450,#4450,#3641,.T.);
#5725=EDGE_CURVE('',#4449,#4451,#2574,.T.);
#5726=EDGE_CURVE('',#4451,#4427,#2575,.T.);
#5727=EDGE_CURVE('',#4428,#4452,#2576,.T.);
#5728=EDGE_CURVE('',#4452,#4453,#2577,.T.);
#5729=EDGE_CURVE('',#4453,#4429,#2578,.T.);
#5730=EDGE_CURVE('',#4454,#4453,#2579,.T.);
#5731=EDGE_CURVE('',#4455,#4454,#2580,.T.);
#5732=EDGE_CURVE('',#4455,#4456,#2581,.T.);
#5733=EDGE_CURVE('',#4457,#4456,#2582,.T.);
#5734=EDGE_CURVE('',#4458,#4457,#2583,.T.);
#5735=EDGE_CURVE('',#4430,#4458,#2584,.T.);
#5736=EDGE_CURVE('',#4458,#4459,#2585,.T.);
#5737=EDGE_CURVE('',#4459,#4431,#2586,.T.);
#5738=EDGE_CURVE('',#4432,#4460,#2587,.T.);
#5739=EDGE_CURVE('',#4460,#4437,#2588,.T.);
#5740=EDGE_CURVE('',#4438,#4461,#2589,.T.);
#5741=EDGE_CURVE('',#4461,#4462,#2590,.T.);
#5742=EDGE_CURVE('',#4462,#4439,#2591,.T.);
#5743=EDGE_CURVE('',#4463,#4462,#2592,.T.);
#5744=EDGE_CURVE('',#4456,#4463,#2593,.T.);
#5745=EDGE_CURVE('',#4464,#4455,#2594,.T.);
#5746=EDGE_CURVE('',#4465,#4464,#2595,.T.);
#5747=EDGE_CURVE('',#4447,#4465,#2596,.T.);
#5748=EDGE_CURVE('',#4466,#4446,#2597,.T.);
#5749=EDGE_CURVE('',#4467,#4466,#2598,.T.);
#5750=EDGE_CURVE('',#4440,#4467,#2599,.T.);
#5751=EDGE_CURVE('',#4468,#4468,#3642,.T.);
#5752=EDGE_CURVE('',#4463,#4469,#2600,.T.);
#5753=EDGE_CURVE('',#4469,#4457,#2601,.T.);
#5754=EDGE_CURVE('',#4454,#4470,#2602,.T.);
#5755=EDGE_CURVE('',#4470,#4464,#2603,.T.);
#5756=EDGE_CURVE('',#4465,#4471,#2604,.T.);
#5757=EDGE_CURVE('',#4471,#4448,#2605,.T.);
#5758=EDGE_CURVE('',#4445,#4472,#2606,.T.);
#5759=EDGE_CURVE('',#4472,#4466,#2607,.T.);
#5760=EDGE_CURVE('',#4473,#4436,#2608,.T.);
#5761=EDGE_CURVE('',#4467,#4473,#2609,.T.);
#5762=EDGE_CURVE('',#4443,#4472,#2610,.T.);
#5763=EDGE_CURVE('',#4474,#4474,#3643,.T.);
#5764=EDGE_CURVE('',#4471,#4451,#2611,.T.);
#5765=EDGE_CURVE('',#4452,#4470,#2612,.T.);
#5766=EDGE_CURVE('',#4469,#4459,#2613,.T.);
#5767=EDGE_CURVE('',#4460,#4461,#2614,.T.);
#5768=EDGE_CURVE('',#4473,#4441,#2615,.T.);
#5769=EDGE_CURVE('',#4400,#4468,#487,.T.);
#5770=EDGE_CURVE('',#4475,#4450,#2616,.T.);
#5771=EDGE_CURVE('',#4476,#4474,#2617,.T.);
#5772=EDGE_CURVE('',#4477,#4442,#2618,.T.);
#5773=EDGE_CURVE('',#4478,#4478,#3644,.T.);
#5774=EDGE_CURVE('',#4478,#4479,#2619,.T.);
#5775=EDGE_CURVE('',#4480,#4479,#3645,.T.);
#5776=EDGE_CURVE('',#4479,#4480,#3646,.T.);
#5777=EDGE_CURVE('',#4481,#4481,#3647,.T.);
#5778=EDGE_CURVE('',#4481,#4478,#2620,.T.);
#5779=EDGE_CURVE('',#4482,#4482,#3648,.T.);
#5780=EDGE_CURVE('',#4482,#4483,#2621,.T.);
#5781=EDGE_CURVE('',#4483,#4483,#3649,.T.);
#5782=EDGE_CURVE('',#4484,#4484,#3650,.T.);
#5783=EDGE_CURVE('',#4482,#4480,#2622,.T.);
#5784=EDGE_CURVE('',#4485,#4486,#3651,.T.);
#5785=EDGE_CURVE('',#4486,#4484,#2623,.T.);
#5786=EDGE_CURVE('',#4486,#4390,#3652,.T.);
#5787=EDGE_CURVE('',#4389,#4485,#488,.T.);
#5788=EDGE_CURVE('',#4405,#4413,#489,.T.);
#5789=EDGE_CURVE('',#4412,#4402,#490,.T.);
#5790=EDGE_CURVE('',#4419,#4390,#491,.T.);
#5791=EDGE_CURVE('',#4485,#4420,#492,.T.);
#7988=ORIENTED_EDGE('',*,*,#5647,.F.);
#7989=ORIENTED_EDGE('',*,*,#5648,.T.);
#7990=ORIENTED_EDGE('',*,*,#5649,.F.);
#7991=ORIENTED_EDGE('',*,*,#5650,.T.);
#7992=ORIENTED_EDGE('',*,*,#5651,.F.);
#7993=ORIENTED_EDGE('',*,*,#5652,.T.);
#7994=ORIENTED_EDGE('',*,*,#5653,.T.);
#7995=ORIENTED_EDGE('',*,*,#5647,.T.);
#7996=ORIENTED_EDGE('',*,*,#5654,.T.);
#7997=ORIENTED_EDGE('',*,*,#5655,.F.);
#7998=ORIENTED_EDGE('',*,*,#5656,.T.);
#7999=ORIENTED_EDGE('',*,*,#5651,.T.);
#8000=ORIENTED_EDGE('',*,*,#5657,.T.);
#8001=ORIENTED_EDGE('',*,*,#5658,.F.);
#8002=ORIENTED_EDGE('',*,*,#5659,.T.);
#8003=ORIENTED_EDGE('',*,*,#5655,.T.);
#8004=ORIENTED_EDGE('',*,*,#5660,.T.);
#8005=ORIENTED_EDGE('',*,*,#5661,.F.);
#8006=ORIENTED_EDGE('',*,*,#5662,.T.);
#8007=ORIENTED_EDGE('',*,*,#5658,.T.);
#8008=ORIENTED_EDGE('',*,*,#5663,.T.);
#8009=ORIENTED_EDGE('',*,*,#5664,.F.);
#8010=ORIENTED_EDGE('',*,*,#5665,.T.);
#8011=ORIENTED_EDGE('',*,*,#5666,.T.);
#8012=ORIENTED_EDGE('',*,*,#5667,.T.);
#8013=ORIENTED_EDGE('',*,*,#5668,.T.);
#8014=ORIENTED_EDGE('',*,*,#5669,.T.);
#8015=ORIENTED_EDGE('',*,*,#5670,.T.);
#8016=ORIENTED_EDGE('',*,*,#5665,.F.);
#8017=ORIENTED_EDGE('',*,*,#5671,.F.);
#8018=ORIENTED_EDGE('',*,*,#5672,.T.);
#8019=ORIENTED_EDGE('',*,*,#5673,.T.);
#8020=ORIENTED_EDGE('',*,*,#5674,.T.);
#8021=ORIENTED_EDGE('',*,*,#5668,.F.);
#8022=ORIENTED_EDGE('',*,*,#5675,.T.);
#8023=ORIENTED_EDGE('',*,*,#5661,.T.);
#8024=ORIENTED_EDGE('',*,*,#5676,.T.);
#8025=ORIENTED_EDGE('',*,*,#5677,.T.);
#8026=ORIENTED_EDGE('',*,*,#5678,.T.);
#8027=ORIENTED_EDGE('',*,*,#5679,.F.);
#8028=ORIENTED_EDGE('',*,*,#5680,.F.);
#8029=ORIENTED_EDGE('',*,*,#5681,.F.);
#8030=ORIENTED_EDGE('',*,*,#5682,.F.);
#8031=ORIENTED_EDGE('',*,*,#5683,.F.);
#8032=ORIENTED_EDGE('',*,*,#5684,.F.);
#8033=ORIENTED_EDGE('',*,*,#5685,.F.);
#8034=ORIENTED_EDGE('',*,*,#5686,.F.);
#8035=ORIENTED_EDGE('',*,*,#5687,.T.);
#8036=ORIENTED_EDGE('',*,*,#5688,.T.);
#8037=ORIENTED_EDGE('',*,*,#5671,.T.);
#8038=ORIENTED_EDGE('',*,*,#5689,.T.);
#8039=ORIENTED_EDGE('',*,*,#5673,.F.);
#8040=ORIENTED_EDGE('',*,*,#5690,.T.);
#8041=ORIENTED_EDGE('',*,*,#5691,.F.);
#8042=ORIENTED_EDGE('',*,*,#5692,.T.);
#8043=ORIENTED_EDGE('',*,*,#5693,.F.);
#8044=ORIENTED_EDGE('',*,*,#5694,.T.);
#8045=ORIENTED_EDGE('',*,*,#5695,.F.);
#8046=ORIENTED_EDGE('',*,*,#5696,.T.);
#8047=ORIENTED_EDGE('',*,*,#5697,.F.);
#8048=ORIENTED_EDGE('',*,*,#5698,.T.);
#8049=ORIENTED_EDGE('',*,*,#5699,.F.);
#8050=ORIENTED_EDGE('',*,*,#5700,.T.);
#8051=ORIENTED_EDGE('',*,*,#5701,.F.);
#8052=ORIENTED_EDGE('',*,*,#5702,.T.);
#8053=ORIENTED_EDGE('',*,*,#5690,.F.);
#8054=ORIENTED_EDGE('',*,*,#5672,.F.);
#8055=ORIENTED_EDGE('',*,*,#5674,.F.);
#8056=ORIENTED_EDGE('',*,*,#5689,.F.);
#8057=ORIENTED_EDGE('',*,*,#5703,.T.);
#8058=ORIENTED_EDGE('',*,*,#5704,.F.);
#8059=ORIENTED_EDGE('',*,*,#5703,.F.);
#8060=ORIENTED_EDGE('',*,*,#5705,.T.);
#8061=ORIENTED_EDGE('',*,*,#5706,.T.);
#8062=ORIENTED_EDGE('',*,*,#5707,.T.);
#8063=ORIENTED_EDGE('',*,*,#5691,.T.);
#8064=ORIENTED_EDGE('',*,*,#5705,.F.);
#8065=ORIENTED_EDGE('',*,*,#5702,.F.);
#8066=ORIENTED_EDGE('',*,*,#5708,.F.);
#8067=ORIENTED_EDGE('',*,*,#5709,.F.);
#8068=ORIENTED_EDGE('',*,*,#5710,.F.);
#8069=ORIENTED_EDGE('',*,*,#5711,.T.);
#8070=ORIENTED_EDGE('',*,*,#5712,.F.);
#8071=ORIENTED_EDGE('',*,*,#5713,.F.);
#8072=ORIENTED_EDGE('',*,*,#5714,.T.);
#8073=ORIENTED_EDGE('',*,*,#5715,.T.);
#8074=ORIENTED_EDGE('',*,*,#5716,.T.);
#8075=ORIENTED_EDGE('',*,*,#5717,.T.);
#8076=ORIENTED_EDGE('',*,*,#5693,.T.);
#8077=ORIENTED_EDGE('',*,*,#5717,.F.);
#8078=ORIENTED_EDGE('',*,*,#5718,.F.);
#8079=ORIENTED_EDGE('',*,*,#5719,.F.);
#8080=ORIENTED_EDGE('',*,*,#5720,.T.);
#8081=ORIENTED_EDGE('',*,*,#5721,.F.);
#8082=ORIENTED_EDGE('',*,*,#5722,.F.);
#8083=ORIENTED_EDGE('',*,*,#5723,.F.);
#8084=ORIENTED_EDGE('',*,*,#5694,.F.);
#8085=ORIENTED_EDGE('',*,*,#5724,.T.);
#8086=ORIENTED_EDGE('',*,*,#5723,.T.);
#8087=ORIENTED_EDGE('',*,*,#5725,.T.);
#8088=ORIENTED_EDGE('',*,*,#5726,.T.);
#8089=ORIENTED_EDGE('',*,*,#5695,.T.);
#8090=ORIENTED_EDGE('',*,*,#5727,.T.);
#8091=ORIENTED_EDGE('',*,*,#5728,.T.);
#8092=ORIENTED_EDGE('',*,*,#5729,.T.);
#8093=ORIENTED_EDGE('',*,*,#5697,.T.);
#8094=ORIENTED_EDGE('',*,*,#5729,.F.);
#8095=ORIENTED_EDGE('',*,*,#5730,.F.);
#8096=ORIENTED_EDGE('',*,*,#5731,.F.);
#8097=ORIENTED_EDGE('',*,*,#5732,.T.);
#8098=ORIENTED_EDGE('',*,*,#5733,.F.);
#8099=ORIENTED_EDGE('',*,*,#5734,.F.);
#8100=ORIENTED_EDGE('',*,*,#5735,.F.);
#8101=ORIENTED_EDGE('',*,*,#5698,.F.);
#8102=ORIENTED_EDGE('',*,*,#5735,.T.);
#8103=ORIENTED_EDGE('',*,*,#5736,.T.);
#8104=ORIENTED_EDGE('',*,*,#5737,.T.);
#8105=ORIENTED_EDGE('',*,*,#5699,.T.);
#8106=ORIENTED_EDGE('',*,*,#5738,.T.);
#8107=ORIENTED_EDGE('',*,*,#5739,.T.);
#8108=ORIENTED_EDGE('',*,*,#5708,.T.);
#8109=ORIENTED_EDGE('',*,*,#5701,.T.);
#8110=ORIENTED_EDGE('',*,*,#5710,.T.);
#8111=ORIENTED_EDGE('',*,*,#5740,.T.);
#8112=ORIENTED_EDGE('',*,*,#5741,.T.);
#8113=ORIENTED_EDGE('',*,*,#5742,.T.);
#8114=ORIENTED_EDGE('',*,*,#5742,.F.);
#8115=ORIENTED_EDGE('',*,*,#5743,.F.);
#8116=ORIENTED_EDGE('',*,*,#5744,.F.);
#8117=ORIENTED_EDGE('',*,*,#5732,.F.);
#8118=ORIENTED_EDGE('',*,*,#5745,.F.);
#8119=ORIENTED_EDGE('',*,*,#5746,.F.);
#8120=ORIENTED_EDGE('',*,*,#5747,.F.);
#8121=ORIENTED_EDGE('',*,*,#5720,.F.);
#8122=ORIENTED_EDGE('',*,*,#5748,.F.);
#8123=ORIENTED_EDGE('',*,*,#5749,.F.);
#8124=ORIENTED_EDGE('',*,*,#5750,.F.);
#8125=ORIENTED_EDGE('',*,*,#5711,.F.);
#8126=ORIENTED_EDGE('',*,*,#5751,.F.);
#8127=ORIENTED_EDGE('',*,*,#5752,.T.);
#8128=ORIENTED_EDGE('',*,*,#5753,.T.);
#8129=ORIENTED_EDGE('',*,*,#5733,.T.);
#8130=ORIENTED_EDGE('',*,*,#5744,.T.);
#8131=ORIENTED_EDGE('',*,*,#5731,.T.);
#8132=ORIENTED_EDGE('',*,*,#5754,.T.);
#8133=ORIENTED_EDGE('',*,*,#5755,.T.);
#8134=ORIENTED_EDGE('',*,*,#5745,.T.);
#8135=ORIENTED_EDGE('',*,*,#5756,.T.);
#8136=ORIENTED_EDGE('',*,*,#5757,.T.);
#8137=ORIENTED_EDGE('',*,*,#5721,.T.);
#8138=ORIENTED_EDGE('',*,*,#5747,.T.);
#8139=ORIENTED_EDGE('',*,*,#5719,.T.);
#8140=ORIENTED_EDGE('',*,*,#5758,.T.);
#8141=ORIENTED_EDGE('',*,*,#5759,.T.);
#8142=ORIENTED_EDGE('',*,*,#5748,.T.);
#8143=ORIENTED_EDGE('',*,*,#5707,.F.);
#8144=ORIENTED_EDGE('',*,*,#5760,.F.);
#8145=ORIENTED_EDGE('',*,*,#5761,.F.);
#8146=ORIENTED_EDGE('',*,*,#5749,.T.);
#8147=ORIENTED_EDGE('',*,*,#5759,.F.);
#8148=ORIENTED_EDGE('',*,*,#5762,.F.);
#8149=ORIENTED_EDGE('',*,*,#5715,.F.);
#8150=ORIENTED_EDGE('',*,*,#5692,.F.);
#8151=ORIENTED_EDGE('',*,*,#5763,.T.);
#8152=ORIENTED_EDGE('',*,*,#5716,.F.);
#8153=ORIENTED_EDGE('',*,*,#5762,.T.);
#8154=ORIENTED_EDGE('',*,*,#5758,.F.);
#8155=ORIENTED_EDGE('',*,*,#5718,.T.);
#8156=ORIENTED_EDGE('',*,*,#5725,.F.);
#8157=ORIENTED_EDGE('',*,*,#5722,.T.);
#8158=ORIENTED_EDGE('',*,*,#5757,.F.);
#8159=ORIENTED_EDGE('',*,*,#5764,.T.);
#8160=ORIENTED_EDGE('',*,*,#5726,.F.);
#8161=ORIENTED_EDGE('',*,*,#5764,.F.);
#8162=ORIENTED_EDGE('',*,*,#5756,.F.);
#8163=ORIENTED_EDGE('',*,*,#5746,.T.);
#8164=ORIENTED_EDGE('',*,*,#5755,.F.);
#8165=ORIENTED_EDGE('',*,*,#5765,.F.);
#8166=ORIENTED_EDGE('',*,*,#5727,.F.);
#8167=ORIENTED_EDGE('',*,*,#5696,.F.);
#8168=ORIENTED_EDGE('',*,*,#5728,.F.);
#8169=ORIENTED_EDGE('',*,*,#5765,.T.);
#8170=ORIENTED_EDGE('',*,*,#5754,.F.);
#8171=ORIENTED_EDGE('',*,*,#5730,.T.);
#8172=ORIENTED_EDGE('',*,*,#5736,.F.);
#8173=ORIENTED_EDGE('',*,*,#5734,.T.);
#8174=ORIENTED_EDGE('',*,*,#5753,.F.);
#8175=ORIENTED_EDGE('',*,*,#5766,.T.);
#8176=ORIENTED_EDGE('',*,*,#5737,.F.);
#8177=ORIENTED_EDGE('',*,*,#5766,.F.);
#8178=ORIENTED_EDGE('',*,*,#5752,.F.);
#8179=ORIENTED_EDGE('',*,*,#5743,.T.);
#8180=ORIENTED_EDGE('',*,*,#5741,.F.);
#8181=ORIENTED_EDGE('',*,*,#5767,.F.);
#8182=ORIENTED_EDGE('',*,*,#5738,.F.);
#8183=ORIENTED_EDGE('',*,*,#5700,.F.);
#8184=ORIENTED_EDGE('',*,*,#5739,.F.);
#8185=ORIENTED_EDGE('',*,*,#5767,.T.);
#8186=ORIENTED_EDGE('',*,*,#5740,.F.);
#8187=ORIENTED_EDGE('',*,*,#5709,.T.);
#8188=ORIENTED_EDGE('',*,*,#5761,.T.);
#8189=ORIENTED_EDGE('',*,*,#5768,.T.);
#8190=ORIENTED_EDGE('',*,*,#5712,.T.);
#8191=ORIENTED_EDGE('',*,*,#5750,.T.);
#8192=ORIENTED_EDGE('',*,*,#5706,.F.);
#8193=ORIENTED_EDGE('',*,*,#5713,.T.);
#8194=ORIENTED_EDGE('',*,*,#5768,.F.);
#8195=ORIENTED_EDGE('',*,*,#5760,.T.);
#8196=ORIENTED_EDGE('',*,*,#5664,.T.);
#8197=ORIENTED_EDGE('',*,*,#5769,.T.);
#8198=ORIENTED_EDGE('',*,*,#5751,.T.);
#8199=ORIENTED_EDGE('',*,*,#5769,.F.);
#8200=ORIENTED_EDGE('',*,*,#5770,.T.);
#8201=ORIENTED_EDGE('',*,*,#5724,.F.);
#8202=ORIENTED_EDGE('',*,*,#5770,.F.);
#8203=ORIENTED_EDGE('',*,*,#5771,.T.);
#8204=ORIENTED_EDGE('',*,*,#5763,.F.);
#8205=ORIENTED_EDGE('',*,*,#5771,.F.);
#8206=ORIENTED_EDGE('',*,*,#5772,.T.);
#8207=ORIENTED_EDGE('',*,*,#5714,.F.);
#8208=ORIENTED_EDGE('',*,*,#5772,.F.);
#8209=ORIENTED_EDGE('',*,*,#5773,.T.);
#8210=ORIENTED_EDGE('',*,*,#5774,.T.);
#8211=ORIENTED_EDGE('',*,*,#5775,.F.);
#8212=ORIENTED_EDGE('',*,*,#5776,.F.);
#8213=ORIENTED_EDGE('',*,*,#5774,.F.);
#8214=ORIENTED_EDGE('',*,*,#5777,.F.);
#8215=ORIENTED_EDGE('',*,*,#5778,.T.);
#8216=ORIENTED_EDGE('',*,*,#5773,.F.);
#8217=ORIENTED_EDGE('',*,*,#5778,.F.);
#8218=ORIENTED_EDGE('',*,*,#5779,.T.);
#8219=ORIENTED_EDGE('',*,*,#5780,.T.);
#8220=ORIENTED_EDGE('',*,*,#5781,.T.);
#8221=ORIENTED_EDGE('',*,*,#5780,.F.);
#8222=ORIENTED_EDGE('',*,*,#5782,.F.);
#8223=ORIENTED_EDGE('',*,*,#5781,.F.);
#8224=ORIENTED_EDGE('',*,*,#5779,.F.);
#8225=ORIENTED_EDGE('',*,*,#5783,.T.);
#8226=ORIENTED_EDGE('',*,*,#5775,.T.);
#8227=ORIENTED_EDGE('',*,*,#5776,.T.);
#8228=ORIENTED_EDGE('',*,*,#5783,.F.);
#8229=ORIENTED_EDGE('',*,*,#5784,.T.);
#8230=ORIENTED_EDGE('',*,*,#5785,.T.);
#8231=ORIENTED_EDGE('',*,*,#5782,.T.);
#8232=ORIENTED_EDGE('',*,*,#5785,.F.);
#8233=ORIENTED_EDGE('',*,*,#5786,.T.);
#8234=ORIENTED_EDGE('',*,*,#5649,.T.);
#8235=ORIENTED_EDGE('',*,*,#5787,.T.);
#8236=ORIENTED_EDGE('',*,*,#5670,.F.);
#8237=ORIENTED_EDGE('',*,*,#5788,.T.);
#8238=ORIENTED_EDGE('',*,*,#5679,.T.);
#8239=ORIENTED_EDGE('',*,*,#5789,.T.);
#8240=ORIENTED_EDGE('',*,*,#5666,.F.);
#8241=ORIENTED_EDGE('',*,*,#5788,.F.);
#8242=ORIENTED_EDGE('',*,*,#5669,.F.);
#8243=ORIENTED_EDGE('',*,*,#5676,.F.);
#8244=ORIENTED_EDGE('',*,*,#5663,.F.);
#8245=ORIENTED_EDGE('',*,*,#5660,.F.);
#8246=ORIENTED_EDGE('',*,*,#5657,.F.);
#8247=ORIENTED_EDGE('',*,*,#5654,.F.);
#8248=ORIENTED_EDGE('',*,*,#5650,.F.);
#8249=ORIENTED_EDGE('',*,*,#5790,.F.);
#8250=ORIENTED_EDGE('',*,*,#5685,.T.);
#8251=ORIENTED_EDGE('',*,*,#5684,.T.);
#8252=ORIENTED_EDGE('',*,*,#5683,.T.);
#8253=ORIENTED_EDGE('',*,*,#5682,.T.);
#8254=ORIENTED_EDGE('',*,*,#5681,.T.);
#8255=ORIENTED_EDGE('',*,*,#5680,.T.);
#8256=ORIENTED_EDGE('',*,*,#5784,.F.);
#8257=ORIENTED_EDGE('',*,*,#5791,.T.);
#8258=ORIENTED_EDGE('',*,*,#5686,.T.);
#8259=ORIENTED_EDGE('',*,*,#5790,.T.);
#8260=ORIENTED_EDGE('',*,*,#5786,.F.);
#8261=ORIENTED_EDGE('',*,*,#5789,.F.);
#8262=ORIENTED_EDGE('',*,*,#5678,.F.);
#8263=ORIENTED_EDGE('',*,*,#5677,.F.);
#8264=ORIENTED_EDGE('',*,*,#5688,.F.);
#8265=ORIENTED_EDGE('',*,*,#5687,.F.);
#8266=ORIENTED_EDGE('',*,*,#5791,.F.);
#8267=ORIENTED_EDGE('',*,*,#5787,.F.);
#8268=ORIENTED_EDGE('',*,*,#5648,.F.);
#8269=ORIENTED_EDGE('',*,*,#5653,.F.);
#8270=ORIENTED_EDGE('',*,*,#5652,.F.);
#8271=ORIENTED_EDGE('',*,*,#5656,.F.);
#8272=ORIENTED_EDGE('',*,*,#5659,.F.);
#8273=ORIENTED_EDGE('',*,*,#5662,.F.);
#8274=ORIENTED_EDGE('',*,*,#5675,.F.);
#8275=ORIENTED_EDGE('',*,*,#5667,.F.);
#8276=ORIENTED_EDGE('',*,*,#5704,.T.);
#8277=ORIENTED_EDGE('',*,*,#5777,.T.);
#9251=CYLINDRICAL_SURFACE('',#10680,0.0025);
#9252=CYLINDRICAL_SURFACE('',#10682,0.0025);
#9253=CYLINDRICAL_SURFACE('',#10683,0.0025);
#9254=CYLINDRICAL_SURFACE('',#10684,0.0025);
#9255=CYLINDRICAL_SURFACE('',#10685,0.0025);
#9256=CYLINDRICAL_SURFACE('',#10686,0.0025);
#9257=CYLINDRICAL_SURFACE('',#10690,0.0025);
#9258=CYLINDRICAL_SURFACE('',#10691,0.002);
#9259=CYLINDRICAL_SURFACE('',#10734,0.0002);
#9260=CYLINDRICAL_SURFACE('',#10741,0.001);
#9643=ADVANCED_FACE('',(#1421),#9251,.T.);
#9644=ADVANCED_FACE('',(#1422),#9252,.T.);
#9645=ADVANCED_FACE('',(#1423),#9253,.T.);
#9646=ADVANCED_FACE('',(#1424),#9254,.T.);
#9647=ADVANCED_FACE('',(#1425),#9255,.T.);
#9648=ADVANCED_FACE('',(#1426),#9256,.T.);
#9649=ADVANCED_FACE('',(#1427),#110,.T.);
#9650=ADVANCED_FACE('',(#1428),#9257,.T.);
#9651=ADVANCED_FACE('',(#1429),#9258,.T.);
#9652=ADVANCED_FACE('',(#1430),#111,.T.);
#9653=ADVANCED_FACE('',(#1431,#753),#1008,.T.);
#9654=ADVANCED_FACE('',(#1432),#647,.T.);
#9655=ADVANCED_FACE('',(#1433),#1009,.T.);
#9656=ADVANCED_FACE('',(#1434,#754),#1010,.T.);
#9657=ADVANCED_FACE('',(#1435),#1011,.T.);
#9658=ADVANCED_FACE('',(#1436,#755),#1012,.T.);
#9659=ADVANCED_FACE('',(#1437),#1013,.T.);
#9660=ADVANCED_FACE('',(#1438),#1014,.T.);
#9661=ADVANCED_FACE('',(#1439),#1015,.T.);
#9662=ADVANCED_FACE('',(#1440),#1016,.T.);
#9663=ADVANCED_FACE('',(#1441),#1017,.T.);
#9664=ADVANCED_FACE('',(#1442),#1018,.T.);
#9665=ADVANCED_FACE('',(#1443,#756),#1019,.F.);
#9666=ADVANCED_FACE('',(#1444),#1020,.T.);
#9667=ADVANCED_FACE('',(#1445),#1021,.T.);
#9668=ADVANCED_FACE('',(#1446),#1022,.T.);
#9669=ADVANCED_FACE('',(#1447),#1023,.T.);
#9670=ADVANCED_FACE('',(#1448,#757),#1024,.T.);
#9671=ADVANCED_FACE('',(#1449),#1025,.T.);
#9672=ADVANCED_FACE('',(#1450),#1026,.T.);
#9673=ADVANCED_FACE('',(#1451),#1027,.T.);
#9674=ADVANCED_FACE('',(#1452),#1028,.T.);
#9675=ADVANCED_FACE('',(#1453),#1029,.T.);
#9676=ADVANCED_FACE('',(#1454),#1030,.T.);
#9677=ADVANCED_FACE('',(#1455),#1031,.T.);
#9678=ADVANCED_FACE('',(#1456),#1032,.T.);
#9679=ADVANCED_FACE('',(#1457),#1033,.T.);
#9680=ADVANCED_FACE('',(#1458),#112,.T.);
#9681=ADVANCED_FACE('',(#1459),#648,.F.);
#9682=ADVANCED_FACE('',(#1460),#649,.F.);
#9683=ADVANCED_FACE('',(#1461),#650,.F.);
#9684=ADVANCED_FACE('',(#1462),#651,.F.);
#9685=ADVANCED_FACE('',(#1463),#9259,.F.);
#9686=ADVANCED_FACE('',(#1464),#652,.F.);
#9687=ADVANCED_FACE('',(#1465,#758),#1034,.F.);
#9688=ADVANCED_FACE('',(#1466),#9260,.F.);
#9689=ADVANCED_FACE('',(#1467),#653,.T.);
#9690=ADVANCED_FACE('',(#1468),#1035,.F.);
#9691=ADVANCED_FACE('',(#1469),#113,.F.);
#9692=ADVANCED_FACE('',(#1470),#1036,.T.);
#9693=ADVANCED_FACE('',(#1471),#114,.F.);
#9694=ADVANCED_FACE('',(#1472,#759),#1037,.T.);
#9878=CLOSED_SHELL('',(#9643,#9644,#9645,#9646,#9647,#9648,#9649,#9650,
#9651,#9652,#9653,#9654,#9655,#9656,#9657,#9658,#9659,#9660,#9661,#9662,
#9663,#9664,#9665,#9666,#9667,#9668,#9669,#9670,#9671,#9672,#9673,#9674,
#9675,#9676,#9677,#9678,#9679,#9680,#9681,#9682,#9683,#9684,#9685,#9686,
#9687,#9688,#9689,#9690,#9691,#9692,#9693,#9694));
#10679=AXIS2_PLACEMENT_3D('',#40491,#12474,#12475);
#10680=AXIS2_PLACEMENT_3D('',#40492,#12476,#12477);
#10681=AXIS2_PLACEMENT_3D('',#40548,#12479,#12480);
#10682=AXIS2_PLACEMENT_3D('',#40579,#12481,#12482);
#10683=AXIS2_PLACEMENT_3D('',#40902,#12484,#12485);
#10684=AXIS2_PLACEMENT_3D('',#41220,#12487,#12488);
#10685=AXIS2_PLACEMENT_3D('',#41540,#12490,#12491);
#10686=AXIS2_PLACEMENT_3D('',#41858,#12493,#12494);
#10687=AXIS2_PLACEMENT_3D('',#41893,#12496,#12497);
#10688=AXIS2_PLACEMENT_3D('',#42023,#12499,#12500);
#10689=AXIS2_PLACEMENT_3D('',#42104,#12501,#12502);
#10690=AXIS2_PLACEMENT_3D('',#42135,#12503,#12504);
#10691=AXIS2_PLACEMENT_3D('',#42454,#12505,#12506);
#10692=AXIS2_PLACEMENT_3D('',#43028,#12507,#12508);
#10693=AXIS2_PLACEMENT_3D('',#43345,#12509,#12510);
#10694=AXIS2_PLACEMENT_3D('',#43609,#12511,#12512);
#10695=AXIS2_PLACEMENT_3D('',#43610,#12513,#12514);
#10696=AXIS2_PLACEMENT_3D('',#43635,#12527,#12528);
#10697=AXIS2_PLACEMENT_3D('',#43638,#12530,#12531);
#10698=AXIS2_PLACEMENT_3D('',#43639,#12532,#12533);
#10699=AXIS2_PLACEMENT_3D('',#43645,#12537,#12538);
#10700=AXIS2_PLACEMENT_3D('',#43658,#12545,#12546);
#10701=AXIS2_PLACEMENT_3D('',#43659,#12547,#12548);
#10702=AXIS2_PLACEMENT_3D('',#43665,#12552,#12553);
#10703=AXIS2_PLACEMENT_3D('',#43678,#12560,#12561);
#10704=AXIS2_PLACEMENT_3D('',#43679,#12562,#12563);
#10705=AXIS2_PLACEMENT_3D('',#43683,#12566,#12567);
#10706=AXIS2_PLACEMENT_3D('',#43689,#12571,#12572);
#10707=AXIS2_PLACEMENT_3D('',#43701,#12579,#12580);
#10708=AXIS2_PLACEMENT_3D('',#43705,#12583,#12584);
#10709=AXIS2_PLACEMENT_3D('',#43709,#12587,#12588);
#10710=AXIS2_PLACEMENT_3D('',#43715,#12592,#12593);
#10711=AXIS2_PLACEMENT_3D('',#43730,#12602,#12603);
#10712=AXIS2_PLACEMENT_3D('',#43731,#12604,#12605);
#10713=AXIS2_PLACEMENT_3D('',#43735,#12608,#12609);
#10714=AXIS2_PLACEMENT_3D('',#43739,#12612,#12613);
#10715=AXIS2_PLACEMENT_3D('',#43743,#12616,#12617);
#10716=AXIS2_PLACEMENT_3D('',#43747,#12620,#12621);
#10717=AXIS2_PLACEMENT_3D('',#43753,#12625,#12626);
#10718=AXIS2_PLACEMENT_3D('',#43754,#12627,#12628);
#10719=AXIS2_PLACEMENT_3D('',#43755,#12629,#12630);
#10720=AXIS2_PLACEMENT_3D('',#43757,#12632,#12633);
#10721=AXIS2_PLACEMENT_3D('',#43759,#12635,#12636);
#10722=AXIS2_PLACEMENT_3D('',#43760,#12637,#12638);
#10723=AXIS2_PLACEMENT_3D('',#43762,#12640,#12641);
#10724=AXIS2_PLACEMENT_3D('',#43764,#12643,#12644);
#10725=AXIS2_PLACEMENT_3D('',#43765,#12645,#12646);
#10726=AXIS2_PLACEMENT_3D('',#43767,#12648,#12649);
#10727=AXIS2_PLACEMENT_3D('',#43845,#12650,#12651);
#10728=AXIS2_PLACEMENT_3D('',#43848,#12653,#12654);
#10729=AXIS2_PLACEMENT_3D('',#43851,#12656,#12657);
#10730=AXIS2_PLACEMENT_3D('',#43854,#12659,#12660);
#10731=AXIS2_PLACEMENT_3D('',#43856,#12661,#12662);
#10732=AXIS2_PLACEMENT_3D('',#43860,#12664,#12665);
#10733=AXIS2_PLACEMENT_3D('',#43861,#12666,#12667);
#10734=AXIS2_PLACEMENT_3D('',#43862,#12668,#12669);
#10735=AXIS2_PLACEMENT_3D('',#43864,#12670,#12671);
#10736=AXIS2_PLACEMENT_3D('',#43866,#12673,#12674);
#10737=AXIS2_PLACEMENT_3D('',#43868,#12675,#12676);
#10738=AXIS2_PLACEMENT_3D('',#43871,#12678,#12679);
#10739=AXIS2_PLACEMENT_3D('',#43872,#12680,#12681);
#10740=AXIS2_PLACEMENT_3D('',#43874,#12682,#12683);
#10741=AXIS2_PLACEMENT_3D('',#43875,#12684,#12685);
#10742=AXIS2_PLACEMENT_3D('',#43877,#12687,#12688);
#10743=AXIS2_PLACEMENT_3D('',#43880,#12689,#12690);
#10744=AXIS2_PLACEMENT_3D('',#43882,#12692,#12693);
#10745=AXIS2_PLACEMENT_3D('',#43889,#12694,#12695);
#10746=AXIS2_PLACEMENT_3D('',#44208,#12696,#12697);
#10747=AXIS2_PLACEMENT_3D('',#44426,#12698,#12699);
#12474=DIRECTION('axis',(0.,0.,1.));
#12475=DIRECTION('refdir',(1.,0.,0.));
#12476=DIRECTION('center_axis',(0.,-1.,2.77555756156289E-17));
#12477=DIRECTION('ref_axis',(-1.,0.,0.));
#12478=DIRECTION('',(0.,1.,-2.77555756156289E-17));
#12479=DIRECTION('center_axis',(0.,1.,-2.77555756156289E-17));
#12480=DIRECTION('ref_axis',(1.,0.,0.));
#12481=DIRECTION('center_axis',(0.,-1.,2.77555756156289E-17));
#12482=DIRECTION('ref_axis',(-1.,0.,0.));
#12483=DIRECTION('',(0.,1.,-2.77555756156289E-17));
#12484=DIRECTION('center_axis',(0.,-1.,2.77555756156289E-17));
#12485=DIRECTION('ref_axis',(-1.,0.,0.));
#12486=DIRECTION('',(0.,1.,-2.77555756156289E-17));
#12487=DIRECTION('center_axis',(0.,-1.,2.77555756156289E-17));
#12488=DIRECTION('ref_axis',(-1.,0.,0.));
#12489=DIRECTION('',(0.,1.,-2.77555756156289E-17));
#12490=DIRECTION('center_axis',(0.,-1.,2.77555756156289E-17));
#12491=DIRECTION('ref_axis',(-1.,0.,0.));
#12492=DIRECTION('',(0.,1.,-2.77555756156289E-17));
#12493=DIRECTION('center_axis',(0.,-1.,2.77555756156289E-17));
#12494=DIRECTION('ref_axis',(-1.,0.,0.));
#12495=DIRECTION('',(0.,1.,-2.77555756156289E-17));
#12496=DIRECTION('center_axis',(0.,-1.,2.77555756156289E-17));
#12497=DIRECTION('ref_axis',(-1.,0.,0.));
#12498=DIRECTION('',(0.,1.,-2.77555756156289E-17));
#12499=DIRECTION('center_axis',(0.,-1.,2.77555756156289E-17));
#12500=DIRECTION('ref_axis',(-1.,0.,0.));
#12501=DIRECTION('center_axis',(0.,-1.,2.77555756156289E-17));
#12502=DIRECTION('ref_axis',(-1.,0.,0.));
#12503=DIRECTION('center_axis',(0.,-1.,2.77555756156289E-17));
#12504=DIRECTION('ref_axis',(-1.,0.,0.));
#12505=DIRECTION('center_axis',(0.,-1.,2.77555756156289E-17));
#12506=DIRECTION('ref_axis',(-1.,-6.24795276412959E-31,-2.251062219229E-14));
#12507=DIRECTION('center_axis',(0.,-1.,2.77555756156289E-17));
#12508=DIRECTION('ref_axis',(-1.,-1.39402673353861E-28,-5.02251062216718E-12));
#12509=DIRECTION('center_axis',(0.,1.,-2.77555756156289E-17));
#12510=DIRECTION('ref_axis',(-1.,-1.39402673353861E-28,-5.02251062216718E-12));
#12511=DIRECTION('center_axis',(0.,-1.,2.77555756156289E-17));
#12512=DIRECTION('ref_axis',(-1.,0.,0.));
#12513=DIRECTION('center_axis',(0.,-1.,2.77555756156289E-17));
#12514=DIRECTION('ref_axis',(1.,0.,0.));
#12515=DIRECTION('',(0.,-2.77555756156289E-17,-1.));
#12516=DIRECTION('',(-0.500000000000316,2.40370335797894E-17,0.866025403784256));
#12517=DIRECTION('',(0.866025403784258,-1.38777878078232E-17,-0.500000000000314));
#12518=DIRECTION('',(-1.,2.77670126733686E-29,1.0004120634318E-12));
#12519=DIRECTION('',(0.866025403784257,1.38777878078232E-17,0.500000000000315));
#12520=DIRECTION('',(-0.500000000000317,-2.40370335797894E-17,-0.866025403784255));
#12521=DIRECTION('',(0.,2.77555756156289E-17,1.));
#12522=DIRECTION('',(0.500000000000317,-2.40370335797894E-17,-0.866025403784256));
#12523=DIRECTION('',(-0.866025403784254,1.38777878078233E-17,0.50000000000032));
#12524=DIRECTION('',(1.,-2.77708250259577E-29,-1.00054941790939E-12));
#12525=DIRECTION('',(-0.866025403784253,-1.38777878078234E-17,-0.500000000000322));
#12526=DIRECTION('',(0.500000000000318,2.40370335797894E-17,0.866025403784255));
#12527=DIRECTION('center_axis',(0.,1.,-2.77555756156289E-17));
#12528=DIRECTION('ref_axis',(-1.,0.,0.));
#12529=DIRECTION('',(-0.6,-0.8,9.56832684413443E-17));
#12530=DIRECTION('center_axis',(0.,-1.,2.77555756156289E-17));
#12531=DIRECTION('ref_axis',(-1.,0.,0.));
#12532=DIRECTION('center_axis',(0.707106781186548,-0.707106781186548,1.96261557335472E-17));
#12533=DIRECTION('ref_axis',(-5.8813528649299E-33,2.77555756156289E-17,
1.));
#12534=DIRECTION('',(0.447213595500212,0.447213595500212,0.77459666924119));
#12535=DIRECTION('',(0.,2.77555756156289E-17,1.));
#12536=DIRECTION('',(-0.447213595500212,-0.447213595500212,0.77459666924119));
#12537=DIRECTION('center_axis',(0.866025403784438,-1.38777878078144E-17,
-0.5));
#12538=DIRECTION('ref_axis',(-5.88504909690158E-32,1.,-2.77555756156289E-17));
#12539=DIRECTION('',(0.447213595500213,-0.447213595500208,0.774596669241192));
#12540=DIRECTION('',(0.,-1.,2.77555756156289E-17));
#12541=DIRECTION('',(-0.447213595500213,-0.447213595500208,-0.774596669241192));
#12542=DIRECTION('',(0.500000000000318,2.40370335797894E-17,0.866025403784255));
#12543=DIRECTION('',(-0.447213595500212,0.447213595500212,-0.77459666924119));
#12544=DIRECTION('',(0.,1.,-2.77555756156289E-17));
#12545=DIRECTION('center_axis',(-0.866025403781998,1.38777878079318E-17,
0.500000000004228));
#12546=DIRECTION('ref_axis',(0.500000000004228,2.40370335797268E-17,0.866025403781998));
#12547=DIRECTION('center_axis',(0.353553390593272,-0.707106781186546,0.612372435695797));
#12548=DIRECTION('ref_axis',(-0.86602540378444,1.41991444031354E-15,0.499999999999998));
#12549=DIRECTION('',(-0.44721359550021,0.447213595500215,0.774596669241189));
#12550=DIRECTION('',(-0.866025403784258,1.38777878078232E-17,0.500000000000314));
#12551=DIRECTION('',(-0.894427190999716,-0.447213595500357,1.00038097340813E-12));
#12552=DIRECTION('center_axis',(4.12063432796478E-16,2.77555756156289E-17,
1.));
#12553=DIRECTION('ref_axis',(0.,1.,-2.77555756156289E-17));
#12554=DIRECTION('',(0.,-1.,2.77555756156289E-17));
#12555=DIRECTION('',(0.894427190999716,-0.447213595500357,-1.0003561480666E-12));
#12556=DIRECTION('',(-1.,2.77670126733686E-29,1.0004120634318E-12));
#12557=DIRECTION('',(0.894427190999716,0.447213595500357,-1.00038097340813E-12));
#12558=DIRECTION('',(0.,1.,-2.77555756156289E-17));
#12559=DIRECTION('',(-0.894427190999716,0.447213595500357,1.0003561480666E-12));
#12560=DIRECTION('center_axis',(0.,-2.77555756156289E-17,-1.));
#12561=DIRECTION('ref_axis',(-1.,0.,0.));
#12562=DIRECTION('center_axis',(-0.353553390593273,-0.707106781186547,0.612372435695796));
#12563=DIRECTION('ref_axis',(-0.866025403784439,-7.69758259559516E-16,-0.499999999999999));
#12564=DIRECTION('',(-0.866025403784257,-1.38777878078232E-17,-0.500000000000315));
#12565=DIRECTION('',(-0.447213595500212,-0.447213595500213,-0.77459666924119));
#12566=DIRECTION('center_axis',(-0.707106781186548,-0.707106781186548,1.96261557335472E-17));
#12567=DIRECTION('ref_axis',(-5.8813528649299E-33,-2.77555756156289E-17,
-1.));
#12568=DIRECTION('',(-0.447213595500212,0.447213595500212,-0.77459666924119));
#12569=DIRECTION('',(0.,-2.77555756156289E-17,-1.));
#12570=DIRECTION('',(0.447213595500212,-0.447213595500212,-0.77459666924119));
#12571=DIRECTION('center_axis',(-0.866025403784439,-1.38777878078144E-17,
-0.5));
#12572=DIRECTION('ref_axis',(-5.58796234969744E-32,-1.,2.77555756156289E-17));
#12573=DIRECTION('',(0.,-1.,2.77555756156289E-17));
#12574=DIRECTION('',(-0.447213595500212,-0.447213595500212,0.77459666924119));
#12575=DIRECTION('',(0.500000000000317,-2.40370335797894E-17,-0.866025403784256));
#12576=DIRECTION('',(-0.447213595500212,0.44721359550021,0.774596669241191));
#12577=DIRECTION('',(0.,1.,-2.77555756156289E-17));
#12578=DIRECTION('',(0.447213595500212,0.44721359550021,-0.774596669241191));
#12579=DIRECTION('center_axis',(-0.353553390593276,-0.707106781186548,-0.612372435695793));
#12580=DIRECTION('ref_axis',(0.866025403784437,-1.39419548385453E-15,-0.500000000000002));
#12581=DIRECTION('',(0.866025403784254,-1.38777878078233E-17,-0.50000000000032));
#12582=DIRECTION('',(0.894427190999715,-0.44721359550036,-1.00047900164617E-12));
#12583=DIRECTION('center_axis',(0.353553390593277,-0.707106781186548,-0.612372435695793));
#12584=DIRECTION('ref_axis',(0.866025403784437,1.74380243674934E-15,0.500000000000003));
#12585=DIRECTION('',(0.894427190999714,0.447213595500361,-1.0005038269877E-12));
#12586=DIRECTION('',(0.866025403784253,1.38777878078234E-17,0.500000000000322));
#12587=DIRECTION('center_axis',(0.353553390593277,0.707106781186548,-0.612372435695793));
#12588=DIRECTION('ref_axis',(-0.894427190999914,0.447213595499961,1.25683885207554E-16));
#12589=DIRECTION('',(-0.866025403784253,-1.38777878078234E-17,-0.500000000000322));
#12590=DIRECTION('',(-0.894427190999714,0.447213595500361,1.00047900164617E-12));
#12591=DIRECTION('',(0.866025403784253,1.38777878078234E-17,0.500000000000322));
#12592=DIRECTION('center_axis',(0.,-1.,2.77555756156289E-17));
#12593=DIRECTION('ref_axis',(1.,0.,0.));
#12594=DIRECTION('',(1.,-2.77708250259577E-29,-1.00054941790939E-12));
#12595=DIRECTION('',(0.866025403784254,-1.38777878078233E-17,-0.50000000000032));
#12596=DIRECTION('',(0.,-2.77555756156289E-17,-1.));
#12597=DIRECTION('',(-0.500000000000317,-2.40370335797894E-17,-0.866025403784255));
#12598=DIRECTION('',(-0.866025403784257,-1.38777878078232E-17,-0.500000000000315));
#12599=DIRECTION('',(-0.866025403784258,1.38777878078232E-17,0.500000000000314));
#12600=DIRECTION('',(-0.500000000000316,2.40370335797894E-17,0.866025403784256));
#12601=DIRECTION('',(0.,2.77555756156289E-17,1.));
#12602=DIRECTION('center_axis',(0.,1.,0.));
#12603=DIRECTION('ref_axis',(0.809016994374948,0.,0.587785252292472));
#12604=DIRECTION('center_axis',(-0.353553390593277,0.707106781186548,-0.612372435695793));
#12605=DIRECTION('ref_axis',(-0.894427190999914,-0.447213595499961,-7.92695080627049E-18));
#12606=DIRECTION('',(-0.894427190999715,-0.44721359550036,1.0005038269877E-12));
#12607=DIRECTION('',(-0.866025403784254,1.38777878078233E-17,0.50000000000032));
#12608=DIRECTION('center_axis',(-0.707106781186548,0.707106781186548,-1.96261557335472E-17));
#12609=DIRECTION('ref_axis',(-0.707106781186548,-0.707106781186548,1.96261557335472E-17));
#12610=DIRECTION('',(0.,2.77555756156289E-17,1.));
#12611=DIRECTION('',(0.447213595500212,0.447213595500212,0.77459666924119));
#12612=DIRECTION('center_axis',(-0.353553390593273,0.707106781186547,0.612372435695796));
#12613=DIRECTION('ref_axis',(2.2218001674842E-16,-0.654653670707978,0.755928946018454));
#12614=DIRECTION('',(0.447213595500212,-0.447213595500213,0.77459666924119));
#12615=DIRECTION('',(0.866025403784257,1.38777878078232E-17,0.500000000000315));
#12616=DIRECTION('center_axis',(0.353553390593272,0.707106781186546,0.612372435695797));
#12617=DIRECTION('ref_axis',(1.93047492713039E-16,-0.65465367070798,0.755928946018453));
#12618=DIRECTION('',(0.866025403784258,-1.38777878078232E-17,-0.500000000000314));
#12619=DIRECTION('',(0.44721359550021,0.447213595500215,-0.774596669241189));
#12620=DIRECTION('center_axis',(0.866025403784439,1.38777878078144E-17,
0.5));
#12621=DIRECTION('ref_axis',(5.58796234969744E-32,1.,-2.77555756156289E-17));
#12622=DIRECTION('',(0.,-1.,2.77555756156289E-17));
#12623=DIRECTION('',(0.447213595500212,-0.447213595500212,-0.77459666924119));
#12624=DIRECTION('',(0.,1.,-2.77555756156289E-17));
#12625=DIRECTION('center_axis',(-0.866025403781999,-1.38777878079317E-17,
-0.500000000004226));
#12626=DIRECTION('ref_axis',(-0.500000000004226,2.40370335797268E-17,0.866025403781999));
#12627=DIRECTION('center_axis',(0.499999999999999,2.40370335797946E-17,
0.866025403784439));
#12628=DIRECTION('ref_axis',(-2.24770773560686E-32,1.,-2.77555756156289E-17));
#12629=DIRECTION('center_axis',(-0.499999999999999,2.40370335797946E-17,
0.866025403784439));
#12630=DIRECTION('ref_axis',(-0.866025403784439,-1.38777878078144E-17,-0.499999999999999));
#12631=DIRECTION('',(0.,-1.,2.77555756156289E-17));
#12632=DIRECTION('center_axis',(-0.866025403784439,1.38777878078144E-17,
0.5));
#12633=DIRECTION('ref_axis',(-0.5,-2.40370335797945E-17,-0.866025403784439));
#12634=DIRECTION('',(0.,1.,-2.77555756156289E-17));
#12635=DIRECTION('center_axis',(-1.,0.,0.));
#12636=DIRECTION('ref_axis',(0.,-2.77555756156289E-17,-1.));
#12637=DIRECTION('center_axis',(-0.500000000000001,-2.40370335797945E-17,
-0.866025403784438));
#12638=DIRECTION('ref_axis',(9.24446373305873E-33,-1.,2.77555756156289E-17));
#12639=DIRECTION('',(0.,-1.,2.77555756156289E-17));
#12640=DIRECTION('center_axis',(-1.65847312553218E-46,-2.77555756156292E-17,
-1.));
#12641=DIRECTION('ref_axis',(1.,-5.49417910395304E-16,1.52494103565577E-32));
#12642=DIRECTION('',(0.,1.,-2.77555756156289E-17));
#12643=DIRECTION('center_axis',(0.500000000000001,-2.40370335797945E-17,
-0.866025403784438));
#12644=DIRECTION('ref_axis',(9.24446373305873E-33,1.,-2.77555756156289E-17));
#12645=DIRECTION('center_axis',(0.707106781186548,0.707106781186548,-1.96261557335472E-17));
#12646=DIRECTION('ref_axis',(5.8813528649299E-33,2.77555756156289E-17,1.));
#12647=DIRECTION('',(0.,-2.77555756156289E-17,-1.));
#12648=DIRECTION('center_axis',(1.,0.,0.));
#12649=DIRECTION('ref_axis',(0.,-1.,2.77555756156289E-17));
#12650=DIRECTION('center_axis',(0.,2.77555756156289E-17,1.));
#12651=DIRECTION('ref_axis',(-1.,0.,0.));
#12652=DIRECTION('',(0.991227900682634,1.25058687706283E-16,0.132163720091021));
#12653=DIRECTION('center_axis',(0.866025403784439,1.38777878078144E-17,
0.5));
#12654=DIRECTION('ref_axis',(-0.5,2.40370335797945E-17,0.866025403784439));
#12655=DIRECTION('',(0.610071089398797,9.93983693090308E-17,-0.79234668288557));
#12656=DIRECTION('center_axis',(0.866025403784438,-1.38777878078144E-17,
-0.5));
#12657=DIRECTION('ref_axis',(0.5,2.40370335797945E-17,0.866025403784438));
#12658=DIRECTION('',(-0.381156811283838,9.57300891824016E-17,-0.92451040297659));
#12659=DIRECTION('center_axis',(0.,1.,-2.77555756156289E-17));
#12660=DIRECTION('ref_axis',(-1.,0.,0.));
#12661=DIRECTION('center_axis',(0.,-1.,2.77555756156289E-17));
#12662=DIRECTION('ref_axis',(-1.,0.,0.));
#12663=DIRECTION('',(0.316227766016838,0.948683298050514,-6.50579831597291E-17));
#12664=DIRECTION('center_axis',(0.,-1.,2.77555756156289E-17));
#12665=DIRECTION('ref_axis',(1.,0.,0.));
#12666=DIRECTION('center_axis',(0.,-1.,2.77555756156289E-17));
#12667=DIRECTION('ref_axis',(1.,0.,0.));
#12668=DIRECTION('center_axis',(0.,1.,-2.77555756156289E-17));
#12669=DIRECTION('ref_axis',(-1.,0.,0.));
#12670=DIRECTION('center_axis',(0.,1.,-2.77555756156289E-17));
#12671=DIRECTION('ref_axis',(-1.,0.,0.));
#12672=DIRECTION('',(0.,1.,-2.77555756156289E-17));
#12673=DIRECTION('center_axis',(0.,1.,-2.77555756156289E-17));
#12674=DIRECTION('ref_axis',(1.,0.,0.));
#12675=DIRECTION('center_axis',(0.,-1.,2.77555756156289E-17));
#12676=DIRECTION('ref_axis',(1.,0.,0.));
#12677=DIRECTION('',(-0.624695047554425,0.78086880944303,5.48296157566908E-17));
#12678=DIRECTION('center_axis',(0.,1.,-2.77555756156289E-17));
#12679=DIRECTION('ref_axis',(1.,0.,0.));
#12680=DIRECTION('center_axis',(0.,-1.,2.77555756156289E-17));
#12681=DIRECTION('ref_axis',(1.,0.,0.));
#12682=DIRECTION('center_axis',(0.,-1.,2.77555756156289E-17));
#12683=DIRECTION('ref_axis',(1.,0.,0.));
#12684=DIRECTION('center_axis',(0.,-1.,2.77555756156289E-17));
#12685=DIRECTION('ref_axis',(1.,0.,0.));
#12686=DIRECTION('',(0.,-1.,2.77555756156289E-17));
#12687=DIRECTION('center_axis',(0.,-1.,2.77555756156289E-17));
#12688=DIRECTION('ref_axis',(1.,0.,0.));
#12689=DIRECTION('center_axis',(0.,1.,-2.77555756156289E-17));
#12690=DIRECTION('ref_axis',(-1.,0.,0.));
#12691=DIRECTION('',(0.707106781186547,0.707106781186548,6.69694498900021E-17));
#12692=DIRECTION('center_axis',(0.,1.,-2.77555756156289E-17));
#12693=DIRECTION('ref_axis',(-1.,0.,0.));
#12694=DIRECTION('center_axis',(0.,-1.,2.77555756156289E-17));
#12695=DIRECTION('ref_axis',(1.,0.,0.));
#12696=DIRECTION('center_axis',(0.,-1.,2.77555756156289E-17));
#12697=DIRECTION('ref_axis',(1.,0.,0.));
#12698=DIRECTION('center_axis',(0.,-1.,2.77555756156289E-17));
#12699=DIRECTION('ref_axis',(1.,0.,0.));
#40491=CARTESIAN_POINT('',(0.,0.,0.));
#40492=CARTESIAN_POINT('Origin',(0.,-0.0397787743898723,-0.0121758532865581));
#40493=CARTESIAN_POINT('',(0.0025,-0.0342786793591244,-0.0121758532865055));
#40494=CARTESIAN_POINT('',(0.0025,-0.0341527041915604,-0.0121758532865581));
#40495=CARTESIAN_POINT('',(0.0025,-0.0397787743898723,-0.0121758532865581));
#40496=CARTESIAN_POINT('',(-0.000771312791324951,-0.0339793475320778,-0.0145540428435752));
#40497=CARTESIAN_POINT('Ctrl Pts',(0.0025,-0.0342786793591244,-0.0121758532864529));
#40498=CARTESIAN_POINT('Ctrl Pts',(0.00250000000000589,-0.0342689904458182,
-0.012315775198942));
#40499=CARTESIAN_POINT('Ctrl Pts',(0.0024882531961583,-0.03425938869533,
-0.0124554668616244));
#40500=CARTESIAN_POINT('Ctrl Pts',(0.00245824343412142,-0.0342474763671746,
-0.0126325974120151));
#40501=CARTESIAN_POINT('Ctrl Pts',(0.00245068049935161,-0.0342448700864197,
-0.0126715763414618));
#40502=CARTESIAN_POINT('Ctrl Pts',(0.00243407926704808,-0.0342398266543392,
-0.0127474282739024));
#40503=CARTESIAN_POINT('Ctrl Pts',(0.0024251232527868,-0.0342373877758851,
-0.0127843081361286));
#40504=CARTESIAN_POINT('Ctrl Pts',(0.0024062581256887,-0.0342327386782671,
-0.012854939410854));
#40505=CARTESIAN_POINT('Ctrl Pts',(0.00239646964780489,-0.0342305253471382,
-0.012888713407758));
#40506=CARTESIAN_POINT('Ctrl Pts',(0.00237353483867019,-0.0342257364384091,
-0.0129620259747392));
#40507=CARTESIAN_POINT('Ctrl Pts',(0.00236010594404936,-0.0342231702677575,
-0.0130014653944082));
#40508=CARTESIAN_POINT('Ctrl Pts',(0.00228201403663924,-0.0342094074385763,
-0.0132133077892516));
#40509=CARTESIAN_POINT('Ctrl Pts',(0.00219944277765854,-0.0341988025597235,
-0.0133784991150409));
#40510=CARTESIAN_POINT('Ctrl Pts',(0.00205806083183455,-0.0341835935557079,
-0.0135971921576275));
#40511=CARTESIAN_POINT('Ctrl Pts',(0.00201373970870775,-0.0341791135405407,
-0.0136593187322613));
#40512=CARTESIAN_POINT('Ctrl Pts',(0.0019362578023308,-0.0341715671202833,
-0.0137580445391356));
#40513=CARTESIAN_POINT('Ctrl Pts',(0.00190472966789206,-0.0341685641590388,
-0.0137958618265926));
#40514=CARTESIAN_POINT('Ctrl Pts',(0.0018566129956555,-0.0341640369097395,
-0.0138502292345201));
#40515=CARTESIAN_POINT('Ctrl Pts',(0.00184087370293039,-0.0341625642386274,
-0.0138675183084103));
#40516=CARTESIAN_POINT('Ctrl Pts',(0.00181091273694596,-0.0341597704547133,
-0.0138995161157817));
#40517=CARTESIAN_POINT('Ctrl Pts',(0.00179674876761949,-0.0341584531897357,
-0.0139142756312608));
#40518=CARTESIAN_POINT('Ctrl Pts',(0.00175949581676491,-0.0341550009644654,
-0.013952153369971));
#40519=CARTESIAN_POINT('Ctrl Pts',(0.00173613226008321,-0.034152848006073,
-0.0139749953224846));
#40520=CARTESIAN_POINT('Ctrl Pts',(0.00163589223795456,-0.0341436854154029,
-0.0140692265481607));
#40521=CARTESIAN_POINT('Ctrl Pts',(0.001555013442751,-0.034136476184694,
-0.014136194036011));
#40522=CARTESIAN_POINT('Ctrl Pts',(0.0013291054312484,-0.0341172236228441,
-0.0143004472511144));
#40523=CARTESIAN_POINT('Ctrl Pts',(0.00117766921487138,-0.0341052282652209,
-0.0143879862814541));
#40524=CARTESIAN_POINT('Ctrl Pts',(0.000979632848000693,-0.0340909598460285,
-0.0144763131149805));
#40525=CARTESIAN_POINT('Ctrl Pts',(0.000940495075546564,-0.034088201164009,
-0.0144925891993804));
#40526=CARTESIAN_POINT('Ctrl Pts',(0.000867704679218025,-0.0340831794288103,
-0.0145207114094512));
#40527=CARTESIAN_POINT('Ctrl Pts',(0.0008341765775287,-0.0340809077905754,
-0.0145328472763923));
#40528=CARTESIAN_POINT('Ctrl Pts',(0.000763952075201242,-0.0340762311916867,
-0.0145565795024953));
#40529=CARTESIAN_POINT('Ctrl Pts',(0.000727224320919134,-0.0340738305391452,
-0.0145680541811659));
#40530=CARTESIAN_POINT('Ctrl Pts',(0.000625046771656675,-0.0340672651317129,
-0.0145974061125373));
#40531=CARTESIAN_POINT('Ctrl Pts',(0.000559110111740278,-0.0340631556915915,
-0.0146134747813474));
#40532=CARTESIAN_POINT('Ctrl Pts',(0.000401109210603117,-0.0340535311559656,
-0.0146452296313665));
#40533=CARTESIAN_POINT('Ctrl Pts',(0.000308660024066335,-0.0340480770336272,
-0.014658480624984));
#40534=CARTESIAN_POINT('Ctrl Pts',(5.58935546999585E-5,-0.0340333072623739,
-0.0146803692307144));
#40535=CARTESIAN_POINT('Ctrl Pts',(-0.000104838370947314,-0.0340240796632803,
-0.0146787958023007));
#40536=CARTESIAN_POINT('Ctrl Pts',(-0.000294387272717696,-0.0340123627511266,
-0.0146586444962111));
#40537=CARTESIAN_POINT('Ctrl Pts',(-0.000324421993547556,-0.0340104803134344,
-0.014654898715805));
#40538=CARTESIAN_POINT('Ctrl Pts',(-0.000373766720059421,-0.03400733424197,
-0.0146478326555677));
#40539=CARTESIAN_POINT('Ctrl Pts',(-0.000393119631909072,-0.0340060867513739,
-0.0146448288749355));
#40540=CARTESIAN_POINT('Ctrl Pts',(-0.000429560748455838,-0.0340037086988993,
-0.014638733526942));
#40541=CARTESIAN_POINT('Ctrl Pts',(-0.000446656034600929,-0.0340025809444483,
-0.0146356906499663));
#40542=CARTESIAN_POINT('Ctrl Pts',(-0.00048558309599664,-0.0339999873585239,
-0.0146283426737115));
#40543=CARTESIAN_POINT('Ctrl Pts',(-0.000507391694341714,-0.0339985158478622,
-0.0146239236953516));
#40544=CARTESIAN_POINT('Ctrl Pts',(-0.000610902259790336,-0.0339914527156919,
-0.01460150731064));
#40545=CARTESIAN_POINT('Ctrl Pts',(-0.000691719849745892,-0.033985704795299,
-0.0145797085697862));
#40546=CARTESIAN_POINT('Ctrl Pts',(-0.00077128512462153,-0.0339799013909928,
-0.0145539027512534));
#40547=CARTESIAN_POINT('',(0.00113497624934891,-0.0339787743898723,-0.014403369597029));
#40548=CARTESIAN_POINT('Origin',(0.,-0.0339787743898823,-0.0121758532865581));
#40549=CARTESIAN_POINT('Ctrl Pts',(0.00113497624934886,-0.0339787743898723,
-0.014403369597029));
#40550=CARTESIAN_POINT('Ctrl Pts',(0.00115174305302593,-0.0339799723697356,
-0.0143948264838489));
#40551=CARTESIAN_POINT('Ctrl Pts',(0.00116840353974554,-0.033981179169348,
-0.0143860992538718));
#40552=CARTESIAN_POINT('Ctrl Pts',(0.00120623568276769,-0.0339839550642577,
-0.0143657342481842));
#40553=CARTESIAN_POINT('Ctrl Pts',(0.00122733150122625,-0.0339855287333036,
-0.0143539810279024));
#40554=CARTESIAN_POINT('Ctrl Pts',(0.00136073400405712,-0.0339956332509063,
-0.0142771044776625));
#40555=CARTESIAN_POINT('Ctrl Pts',(0.00146798869649448,-0.034004448180033,
-0.0142036252280775));
#40556=CARTESIAN_POINT('Ctrl Pts',(0.00167396607523132,-0.0340223545464033,
-0.01403757293468));
#40557=CARTESIAN_POINT('Ctrl Pts',(0.00177188415327335,-0.0340314110851452,
-0.0139446369443402));
#40558=CARTESIAN_POINT('Ctrl Pts',(0.00189306870728335,-0.0340432617355753,
-0.0138094017792567));
#40559=CARTESIAN_POINT('Ctrl Pts',(0.00192331473162106,-0.0340462837571465,
-0.0137736801397658));
#40560=CARTESIAN_POINT('Ctrl Pts',(0.00197664900583011,-0.0340517359007246,
-0.0137069799400376));
#40561=CARTESIAN_POINT('Ctrl Pts',(0.00200005576914848,-0.0340541762926233,
-0.0136762756519943));
#40562=CARTESIAN_POINT('Ctrl Pts',(0.00205136640329276,-0.0340596418664449,
-0.0136056323496693));
#40563=CARTESIAN_POINT('Ctrl Pts',(0.00207883326513204,-0.0340626516850083,
-0.0135653945751912));
#40564=CARTESIAN_POINT('Ctrl Pts',(0.00217624493939696,-0.0340736790003726,
-0.0134133305290349));
#40565=CARTESIAN_POINT('Ctrl Pts',(0.00223848717160619,-0.0340814420427912,
-0.0132968227129049));
#40566=CARTESIAN_POINT('Ctrl Pts',(0.00235851704548095,-0.0340988979417139,
-0.0130218272845133));
#40567=CARTESIAN_POINT('Ctrl Pts',(0.0024100572343524,-0.0341084849121217,
-0.0128613378466486));
#40568=CARTESIAN_POINT('Ctrl Pts',(0.0024545293322669,-0.0341213685515389,
-0.0126526484567885));
#40569=CARTESIAN_POINT('Ctrl Pts',(0.00246275705248113,-0.0341241409621192,
-0.0126081437409061));
#40570=CARTESIAN_POINT('Ctrl Pts',(0.00247331312517072,-0.0341283990194741,
-0.0125408791313476));
#40571=CARTESIAN_POINT('Ctrl Pts',(0.00247654466224529,-0.0341298417895595,
-0.0125182684277932));
#40572=CARTESIAN_POINT('Ctrl Pts',(0.00248195972464071,-0.034132547103682,
-0.0124762798085279));
#40573=CARTESIAN_POINT('Ctrl Pts',(0.0024842270701644,-0.0341338054021254,
-0.0124569154713321));
#40574=CARTESIAN_POINT('Ctrl Pts',(0.00248947277206638,-0.0341370706641842,
-0.0124070738843198));
#40575=CARTESIAN_POINT('Ctrl Pts',(0.00249211791730572,-0.0341390940066405,
-0.0123765663429026));
#40576=CARTESIAN_POINT('Ctrl Pts',(0.00249806805641862,-0.0341449339347089,
-0.0122893525724859));
#40577=CARTESIAN_POINT('Ctrl Pts',(0.0025,-0.0341488010148688,-0.0122325976807982));
#40578=CARTESIAN_POINT('Ctrl Pts',(0.0025,-0.0341527041915604,-0.0121758532865581));
#40579=CARTESIAN_POINT('Origin',(0.,-0.0397787743898723,-0.0121758532865581));
#40580=CARTESIAN_POINT('',(0.0025,-0.0352796511099541,-0.0121758532865581));
#40581=CARTESIAN_POINT('',(0.0025,-0.0351559292844039,-0.0121758532867805));
#40582=CARTESIAN_POINT('',(0.0025,-0.0397787743898723,-0.0121758532865581));
#40583=CARTESIAN_POINT('',(0.00249999913488366,-0.0342788233790735,-0.0121737734834589));
#40584=CARTESIAN_POINT('Ctrl Pts',(0.0025,-0.0352796511099541,-0.0121758532865581));
#40585=CARTESIAN_POINT('Ctrl Pts',(0.0025,-0.0352737283576379,-0.0122771833963633));
#40586=CARTESIAN_POINT('Ctrl Pts',(0.00249383929029918,-0.0352677434542228,
-0.0123784711776437));
#40587=CARTESIAN_POINT('Ctrl Pts',(0.00247798453785767,-0.0352596957712184,
-0.0125081910504146));
#40588=CARTESIAN_POINT('Ctrl Pts',(0.0024739263012976,-0.0352578733696817,
-0.0125371623558298));
#40589=CARTESIAN_POINT('Ctrl Pts',(0.00246625181006756,-0.0352547661812909,
-0.012585729857012));
#40590=CARTESIAN_POINT('Ctrl Pts',(0.00246290802346204,-0.0352534952910727,
-0.0126053656031181));
#40591=CARTESIAN_POINT('Ctrl Pts',(0.00245492731469495,-0.0352506316714374,
-0.0126490683004793));
#40592=CARTESIAN_POINT('Ctrl Pts',(0.00245017084734073,-0.0352490333102353,
-0.0126731090348513));
#40593=CARTESIAN_POINT('Ctrl Pts',(0.00243316671274258,-0.0352436613680692,
-0.0127528758109736));
#40594=CARTESIAN_POINT('Ctrl Pts',(0.00241936555138658,-0.0352398204035837,
-0.0128082492058634));
#40595=CARTESIAN_POINT('Ctrl Pts',(0.00237669656419295,-0.0352292423937706,
-0.0129574868825818));
#40596=CARTESIAN_POINT('Ctrl Pts',(0.00234417392000077,-0.035222425284202,
-0.0130502017176979));
#40597=CARTESIAN_POINT('Ctrl Pts',(0.0022507778016247,-0.0352056799802343,
-0.0132734335079112));
#40598=CARTESIAN_POINT('Ctrl Pts',(0.00218391902487044,-0.0351958229917732,
-0.0134010841390569));
#40599=CARTESIAN_POINT('Ctrl Pts',(0.00207961062791622,-0.0351830183298481,
-0.0135642704148632));
#40600=CARTESIAN_POINT('Ctrl Pts',(0.00205152600405622,-0.0351797661256388,
-0.0136054420740379));
#40601=CARTESIAN_POINT('Ctrl Pts',(0.00200149225271985,-0.0351742874609104,
-0.0136742766385462));
#40602=CARTESIAN_POINT('Ctrl Pts',(0.00198015446319433,-0.0351720395367643,
-0.0137023631235021));
#40603=CARTESIAN_POINT('Ctrl Pts',(0.00193462116135819,-0.035167417151577,
-0.0137597355675134));
#40604=CARTESIAN_POINT('Ctrl Pts',(0.00191033808636,-0.0351650468422292,
-0.0137889406221594));
#40605=CARTESIAN_POINT('Ctrl Pts',(0.00184171873199297,-0.0351585918204036,
-0.0138677446077711));
#40606=CARTESIAN_POINT('Ctrl Pts',(0.00179605271034649,-0.0351545604975022,
-0.0139161463236));
#40607=CARTESIAN_POINT('Ctrl Pts',(0.00168346872446355,-0.0351451479767051,
-0.0140263163891485));
#40608=CARTESIAN_POINT('Ctrl Pts',(0.00161500103908194,-0.0351398245317568,
-0.0140863646356792));
#40609=CARTESIAN_POINT('Ctrl Pts',(0.00141402858550948,-0.0351249456416134,
-0.0142440824138003));
#40610=CARTESIAN_POINT('Ctrl Pts',(0.00127496011407219,-0.0351154935490178,
-0.0143325897878295));
#40611=CARTESIAN_POINT('Ctrl Pts',(0.00110211596984762,-0.035103566079878,
-0.0144200005206734));
#40612=CARTESIAN_POINT('Ctrl Pts',(0.00107577231503863,-0.0351017429892431,
-0.0144327472083214));
#40613=CARTESIAN_POINT('Ctrl Pts',(0.00103112294808702,-0.035098634490036,
-0.0144533920129587));
#40614=CARTESIAN_POINT('Ctrl Pts',(0.00101293599230588,-0.035097362978955,
-0.0144615387040784));
#40615=CARTESIAN_POINT('Ctrl Pts',(0.000972145703499203,-0.0350944971059487,
-0.0144792278873622));
#40616=CARTESIAN_POINT('Ctrl Pts',(0.00094949746231122,-0.0350928970920234,
-0.0144886559759031));
#40617=CARTESIAN_POINT('Ctrl Pts',(0.000873621012950118,-0.0350875161348841,
-0.0145189397930628));
#40618=CARTESIAN_POINT('Ctrl Pts',(0.000819819391895106,-0.0350836676083418,
-0.0145383018546116));
#40619=CARTESIAN_POINT('Ctrl Pts',(0.00067160987331214,-0.0350730578694784,
-0.0145859669385363));
#40620=CARTESIAN_POINT('Ctrl Pts',(0.000576115457086386,-0.0350662162401795,
-0.0146105601551931));
#40621=CARTESIAN_POINT('Ctrl Pts',(0.000338965597307982,-0.0350494977406898,
-0.0146568981415619));
#40622=CARTESIAN_POINT('Ctrl Pts',(0.00019639562575315,-0.0350396915727571,
-0.0146722346199108));
#40623=CARTESIAN_POINT('Ctrl Pts',(3.48141957141785E-6,-0.0350269350471675,
-0.0146763470457643));
#40624=CARTESIAN_POINT('Ctrl Pts',(-4.63416875190967E-5,-0.0350236838617148,
-0.0146759201192626));
#40625=CARTESIAN_POINT('Ctrl Pts',(-0.00013137431303332,-0.0350182055133934,
-0.0146726483072451));
#40626=CARTESIAN_POINT('Ctrl Pts',(-0.000166595580792309,-0.0350159569371864,
-0.0146705457924425));
#40627=CARTESIAN_POINT('Ctrl Pts',(-0.000239647539862756,-0.0350113318197795,
-0.0146646308536982));
#40628=CARTESIAN_POINT('Ctrl Pts',(-0.000277459625399993,-0.0350089594621896,
-0.0146606995831));
#40629=CARTESIAN_POINT('Ctrl Pts',(-0.000381286172679116,-0.0350024942746665,
-0.0146475051500353));
#40630=CARTESIAN_POINT('Ctrl Pts',(-0.000447044344062764,-0.0349984550887338,
-0.0146364618499308));
#40631=CARTESIAN_POINT('Ctrl Pts',(-0.000601625458324209,-0.0349890187403755,
-0.0146040991616407));
#40632=CARTESIAN_POINT('Ctrl Pts',(-0.000689876192816882,-0.0349836797591199,
-0.0145805161311376));
#40633=CARTESIAN_POINT('Ctrl Pts',(-0.000932425387999368,-0.0349688188016036,
-0.0145012443159997));
#40634=CARTESIAN_POINT('Ctrl Pts',(-0.00108280541376209,-0.0349593977567418,
-0.0144351408233916));
#40635=CARTESIAN_POINT('Ctrl Pts',(-0.00125118423705539,-0.0349475026601224,
-0.0143404314239675));
#40636=CARTESIAN_POINT('Ctrl Pts',(-0.0012764952656036,-0.0349456754142555,
-0.01432560214918));
#40637=CARTESIAN_POINT('Ctrl Pts',(-0.00131855085643177,-0.034942562968225,
-0.0142999579646947));
#40638=CARTESIAN_POINT('Ctrl Pts',(-0.0013354371943393,-0.0349412917973962,
-0.0142893822109742));
#40639=CARTESIAN_POINT('Ctrl Pts',(-0.00137275373997812,-0.0349384322130194,
-0.0142653854200478));
#40640=CARTESIAN_POINT('Ctrl Pts',(-0.0013931152808018,-0.0349368382684344,
-0.014251865587376));
#40641=CARTESIAN_POINT('Ctrl Pts',(-0.00146001580243708,-0.0349314968683617,
-0.0142060170070799));
#40642=CARTESIAN_POINT('Ctrl Pts',(-0.00150565126222838,-0.0349276829321327,
-0.0141724063642376));
#40643=CARTESIAN_POINT('Ctrl Pts',(-0.00162619100530393,-0.0349172144971981,
-0.0140771445083684));
#40644=CARTESIAN_POINT('Ctrl Pts',(-0.00169871417846689,-0.0349104814565078,
-0.0140126370325997));
#40645=CARTESIAN_POINT('Ctrl Pts',(-0.0018702580661283,-0.0348936947865843,
-0.0138411828317261));
#40646=CARTESIAN_POINT('Ctrl Pts',(-0.00196404013687724,-0.0348837131726053,
-0.0137294762447948));
#40647=CARTESIAN_POINT('Ctrl Pts',(-0.00207615499489246,-0.0348707937864232,
-0.0135694320090113));
#40648=CARTESIAN_POINT('Ctrl Pts',(-0.00210351034160456,-0.0348675423799178,
-0.0135277874646796));
#40649=CARTESIAN_POINT('Ctrl Pts',(-0.0021480636276629,-0.0348620662428828,
-0.0134553315183505));
#40650=CARTESIAN_POINT('Ctrl Pts',(-0.00216588647483754,-0.0348598200184832,
-0.0134249240903401));
#40651=CARTESIAN_POINT('Ctrl Pts',(-0.00220154332330296,-0.0348552024123791,
-0.0133610306533227));
#40652=CARTESIAN_POINT('Ctrl Pts',(-0.00221927013416792,-0.0348528351504397,
-0.0133274950296997));
#40653=CARTESIAN_POINT('Ctrl Pts',(-0.00226589133500932,-0.0348463933289219,
-0.013234219293502));
#40654=CARTESIAN_POINT('Ctrl Pts',(-0.00229318207892717,-0.0348423718817109,
-0.0131737105690229));
#40655=CARTESIAN_POINT('Ctrl Pts',(-0.00235198570859494,-0.0348329897712581,
-0.0130281328476765));
#40656=CARTESIAN_POINT('Ctrl Pts',(-0.0023813413657695,-0.0348276863615184,
-0.0129422943152839));
#40657=CARTESIAN_POINT('Ctrl Pts',(-0.00245089171485022,-0.0348127771057478,
-0.0126959199882142));
#40658=CARTESIAN_POINT('Ctrl Pts',(-0.00247990987111939,-0.0348032782901581,
-0.0125327474543379));
#40659=CARTESIAN_POINT('Ctrl Pts',(-0.00249485035638801,-0.0347913016097072,
-0.012338861396878));
#40660=CARTESIAN_POINT('Ctrl Pts',(-0.00249658151021034,-0.0347894851826981,
-0.0123097582443375));
#40661=CARTESIAN_POINT('Ctrl Pts',(-0.00249863727622723,-0.0347863853039192,
-0.0122607516109443));
#40662=CARTESIAN_POINT('Ctrl Pts',(-0.00249923381653334,-0.0347851156123171,
-0.012240862990334));
#40663=CARTESIAN_POINT('Ctrl Pts',(-0.00250003567650427,-0.0347822511558717,
-0.0121964359270043));
#40664=CARTESIAN_POINT('Ctrl Pts',(-0.00250011725465795,-0.0347806506849812,
-0.0121718995581665));
#40665=CARTESIAN_POINT('Ctrl Pts',(-0.00249918491759101,-0.0347752606909682,
-0.0120900812205439));
#40666=CARTESIAN_POINT('Ctrl Pts',(-0.00249656323300301,-0.0347714031510676,
-0.0120328388236775));
#40667=CARTESIAN_POINT('Ctrl Pts',(-0.00248406381804999,-0.0347607589941701,
-0.0118771843812791));
#40668=CARTESIAN_POINT('Ctrl Pts',(-0.00247030979190908,-0.0347538912629718,
-0.0117791864073395));
#40669=CARTESIAN_POINT('Ctrl Pts',(-0.00242253787305385,-0.0347371464752765,
-0.0115419875563959));
#40670=CARTESIAN_POINT('Ctrl Pts',(-0.00238229176058288,-0.0347273403432799,
-0.0114043798598893));
#40671=CARTESIAN_POINT('Ctrl Pts',(-0.0023124426663361,-0.034714581181683,
-0.0112244890987779));
#40672=CARTESIAN_POINT('Ctrl Pts',(-0.00229301275046583,-0.0347113272335813,
-0.0111785679759999));
#40673=CARTESIAN_POINT('Ctrl Pts',(-0.00225750900482489,-0.0347058460402081,
-0.011101191635245));
#40674=CARTESIAN_POINT('Ctrl Pts',(-0.00224211888896316,-0.0347035973048026,
-0.0110694412202372));
#40675=CARTESIAN_POINT('Ctrl Pts',(-0.00220877457923461,-0.0346989736008557,
-0.0110042059535001));
#40676=CARTESIAN_POINT('Ctrl Pts',(-0.0021907187591027,-0.0346966027780981,
-0.0109707830927261));
#40677=CARTESIAN_POINT('Ctrl Pts',(-0.00213896637873289,-0.0346901468490987,
-0.0108799955127675));
#40678=CARTESIAN_POINT('Ctrl Pts',(-0.00210373030650426,-0.0346861151041094,
-0.010823542523949));
#40679=CARTESIAN_POINT('Ctrl Pts',(-0.00201504598976053,-0.0346767004594844,
-0.0106933304108255));
#40680=CARTESIAN_POINT('Ctrl Pts',(-0.00195973785539656,-0.0346713753060738,
-0.0106209535195878));
#40681=CARTESIAN_POINT('Ctrl Pts',(-0.00179391365990515,-0.0346565070988832,
-0.0104268978815339));
#40682=CARTESIAN_POINT('Ctrl Pts',(-0.00167519341524708,-0.0346470665395916,
-0.0103128757264084));
#40683=CARTESIAN_POINT('Ctrl Pts',(-0.00152315075834697,-0.0346351516612502,
-0.0101932111141045));
#40684=CARTESIAN_POINT('Ctrl Pts',(-0.00149981465869832,-0.034633326671725,
-0.0101754998091879));
#40685=CARTESIAN_POINT('Ctrl Pts',(-0.00146005539847901,-0.034630213585713,
-0.0101464107249192));
#40686=CARTESIAN_POINT('Ctrl Pts',(-0.00144379775285785,-0.0346289393583023,
-0.0101348126469914));
#40687=CARTESIAN_POINT('Ctrl Pts',(-0.00140715559342006,-0.0346260624641363,
-0.0101093293173079));
#40688=CARTESIAN_POINT('Ctrl Pts',(-0.00138670289505513,-0.0346244540307896,
-0.0100955496669878));
#40689=CARTESIAN_POINT('Ctrl Pts',(-0.00131767199853158,-0.0346190252680089,
-0.0100505116017802));
#40690=CARTESIAN_POINT('Ctrl Pts',(-0.00126821736329774,-0.0346151362338775,
-0.0100206362456736));
#40691=CARTESIAN_POINT('Ctrl Pts',(-0.00113005790033621,-0.0346043556512447,
-0.00994357699891012));
#40692=CARTESIAN_POINT('Ctrl Pts',(-0.00103947295709561,-0.0345973817149763,
-0.00989998351372832));
#40693=CARTESIAN_POINT('Ctrl Pts',(-0.000817317040240532,-0.0345807880205129,
-0.00980910915411257));
#40694=CARTESIAN_POINT('Ctrl Pts',(-0.000683906107050634,-0.0345712359493515,
-0.00976716765936511));
#40695=CARTESIAN_POINT('Ctrl Pts',(-0.000499157737457075,-0.0345587217490452,
-0.00972568710585009));
#40696=CARTESIAN_POINT('Ctrl Pts',(-0.000450322081987992,-0.0345554768339693,
-0.00971624288290118));
#40697=CARTESIAN_POINT('Ctrl Pts',(-0.000366359927380762,-0.0345500014398331,
-0.00970259050555726));
#40698=CARTESIAN_POINT('Ctrl Pts',(-0.000331367910254513,-0.0345477498223317,
-0.00969765961177541));
#40699=CARTESIAN_POINT('Ctrl Pts',(-0.00025836570147237,-0.0345431109971148,
-0.00968894652041296));
#40700=CARTESIAN_POINT('Ctrl Pts',(-0.000220349580041532,-0.0345407281429581,
-0.00968529021697187));
#40701=CARTESIAN_POINT('Ctrl Pts',(-0.000115083207838991,-0.0345342096616183,
-0.00967759527502233));
#40702=CARTESIAN_POINT('Ctrl Pts',(-4.77289176190029E-5,-0.034530129033425,
-0.00967540127058989));
#40703=CARTESIAN_POINT('Ctrl Pts',(0.000112395044014337,-0.0345205656371134,
-0.00967665899731326));
#40704=CARTESIAN_POINT('Ctrl Pts',(0.000205045019048902,-0.0345151433717406,
-0.0096825497271631));
#40705=CARTESIAN_POINT('Ctrl Pts',(0.000456794418630767,-0.0345003804972055,
-0.00971268695829775));
#40706=CARTESIAN_POINT('Ctrl Pts',(0.000614197895265314,-0.0344911282724244,
-0.00974715027266843));
#40707=CARTESIAN_POINT('Ctrl Pts',(0.000795455547349672,-0.0344794091892002,
-0.0098055931852241));
#40708=CARTESIAN_POINT('Ctrl Pts',(0.000823562568213125,-0.0344775597722573,
-0.00981521206143733));
#40709=CARTESIAN_POINT('Ctrl Pts',(0.000870229185463951,-0.0344744247707291,
-0.00983211729452332));
#40710=CARTESIAN_POINT('Ctrl Pts',(0.000888884696183502,-0.0344731538804419,
-0.00983912882522668));
#40711=CARTESIAN_POINT('Ctrl Pts',(0.000929847402013366,-0.0344703214682339,
-0.00985508589381992));
#40712=CARTESIAN_POINT('Ctrl Pts',(0.000952111331147731,-0.0344687549775865,
-0.00986413068409234));
#40713=CARTESIAN_POINT('Ctrl Pts',(0.00102435125151682,-0.0344635913345055,
-0.00989469892168406));
#40714=CARTESIAN_POINT('Ctrl Pts',(0.0010737529249031,-0.034459932618979,
-0.0099175321172254));
#40715=CARTESIAN_POINT('Ctrl Pts',(0.00120309491152283,-0.0344500783895446,
-0.00998251682775234));
#40716=CARTESIAN_POINT('Ctrl Pts',(0.00128156241638059,-0.0344438125132599,
-0.0100274215797191));
#40717=CARTESIAN_POINT('Ctrl Pts',(0.00148927752055119,-0.0344266722724442,
-0.0101617266769406));
#40718=CARTESIAN_POINT('Ctrl Pts',(0.00161282305172891,-0.034415869697555,
-0.0102592239452315));
#40719=CARTESIAN_POINT('Ctrl Pts',(0.00176215409281682,-0.0344022211451491,
-0.0104018029790606));
#40720=CARTESIAN_POINT('Ctrl Pts',(0.0017968745929216,-0.034398996343267,
-0.0104369789987399));
#40721=CARTESIAN_POINT('Ctrl Pts',(0.00185438199177565,-0.0343935609645254,
-0.01049880417321));
#40722=CARTESIAN_POINT('Ctrl Pts',(0.00187769182175053,-0.0343913291775538,
-0.0105249444700266));
#40723=CARTESIAN_POINT('Ctrl Pts',(0.00192494248141358,-0.0343867401775118,
-0.0105802286361311));
#40724=CARTESIAN_POINT('Ctrl Pts',(0.0019487886479754,-0.0343843870709691,
-0.0106094419030752));
#40725=CARTESIAN_POINT('Ctrl Pts',(0.00201246984772701,-0.0343779877183206,
-0.0106911622899306));
#40726=CARTESIAN_POINT('Ctrl Pts',(0.00205090501795098,-0.0343739940692101,
-0.0107447237002124));
#40727=CARTESIAN_POINT('Ctrl Pts',(0.0021366190938103,-0.0343646899409113,
-0.0108747285746264));
#40728=CARTESIAN_POINT('Ctrl Pts',(0.00218198220270771,-0.0343594357387127,
-0.0109523249243086));
#40729=CARTESIAN_POINT('Ctrl Pts',(0.00229942111359487,-0.0343444900436488,
-0.0111806061415237));
#40730=CARTESIAN_POINT('Ctrl Pts',(0.00236070736120421,-0.0343349134514614,
-0.0113362691455636));
#40731=CARTESIAN_POINT('Ctrl Pts',(0.00241391784569683,-0.0343228479597993,
-0.011524819440807));
#40732=CARTESIAN_POINT('Ctrl Pts',(0.00242132170961338,-0.0343210374697997,
-0.0115529203501193));
#40733=CARTESIAN_POINT('Ctrl Pts',(0.00243295361025697,-0.0343179471798899,
-0.0116004139777165));
#40734=CARTESIAN_POINT('Ctrl Pts',(0.00243744344825402,-0.034316681104037,
-0.0116197390274582));
#40735=CARTESIAN_POINT('Ctrl Pts',(0.0024469583218066,-0.0343138240267315,
-0.0116630237408342));
#40736=CARTESIAN_POINT('Ctrl Pts',(0.00245186197514166,-0.0343122273176846,
-0.0116870057467782));
#40737=CARTESIAN_POINT('Ctrl Pts',(0.00246160256896688,-0.0343087760115555,
-0.0117384837852018));
#40738=CARTESIAN_POINT('Ctrl Pts',(0.00246633264409253,-0.0343069169375645,
-0.0117659966725079));
#40739=CARTESIAN_POINT('Ctrl Pts',(0.00249006680650221,-0.034296491498923,
-0.011919389326348));
#40740=CARTESIAN_POINT('Ctrl Pts',(0.00249989323900895,-0.0342876380916422,
-0.0120464827820831));
#40741=CARTESIAN_POINT('Ctrl Pts',(0.00249999913488366,-0.0342788233790734,
-0.0121737734834593));
#40742=CARTESIAN_POINT('Ctrl Pts',(0.00249999913488366,-0.0342788233790735,
-0.0121737734834589));
#40743=CARTESIAN_POINT('Ctrl Pts',(0.00249999971163259,-0.0342787753708198,
-0.0121744667566923));
#40744=CARTESIAN_POINT('Ctrl Pts',(0.00249999999999997,-0.0342787273641556,
-0.0121751600244162));
#40745=CARTESIAN_POINT('Ctrl Pts',(0.0025,-0.0342786793591244,-0.0121758532864529));
#40746=CARTESIAN_POINT('Ctrl Pts',(0.0025,-0.0341527041915604,-0.0121758532865581));
#40747=CARTESIAN_POINT('Ctrl Pts',(0.0025,-0.0341588066255373,-0.0120871360834245));
#40748=CARTESIAN_POINT('Ctrl Pts',(0.00249527753979069,-0.0341649953633893,
-0.0119984444073263));
#40749=CARTESIAN_POINT('Ctrl Pts',(0.00247527802227061,-0.0341780560342344,
-0.0118113307178051));
#40750=CARTESIAN_POINT('Ctrl Pts',(0.0024588306282862,-0.034184905362994,
-0.0117132164488123));
#40751=CARTESIAN_POINT('Ctrl Pts',(0.00242104579703883,-0.034196288560602,
-0.0115486714482207));
#40752=CARTESIAN_POINT('Ctrl Pts',(0.002402695164542,-0.0342008942560627,
-0.0114816794736156));
#40753=CARTESIAN_POINT('Ctrl Pts',(0.00237028452718894,-0.0342078267516067,
-0.0113801585393498));
#40754=CARTESIAN_POINT('Ctrl Pts',(0.00235820408642621,-0.0342102163424318,
-0.0113450388630887));
#40755=CARTESIAN_POINT('Ctrl Pts',(0.00233392831921142,-0.0342146782956228,
-0.0112792676887648));
#40756=CARTESIAN_POINT('Ctrl Pts',(0.0023219002592204,-0.0342167557500717,
-0.0112485634233305));
#40757=CARTESIAN_POINT('Ctrl Pts',(0.00229279761930796,-0.0342214953478311,
-0.0111783928168259));
#40758=CARTESIAN_POINT('Ctrl Pts',(0.00227530506476294,-0.0342241424844795,
-0.0111391105392396));
#40759=CARTESIAN_POINT('Ctrl Pts',(0.00220319579794283,-0.0342343399942572,
-0.0109878058473953));
#40760=CARTESIAN_POINT('Ctrl Pts',(0.00214124627572804,-0.0342416334892694,
-0.0108794746021455));
#40761=CARTESIAN_POINT('Ctrl Pts',(0.00197772515517029,-0.0342585269327383,
-0.0106374644220687));
#40762=CARTESIAN_POINT('Ctrl Pts',(0.00187028961638902,-0.0342680078613533,
-0.0105085073887182));
#40763=CARTESIAN_POINT('Ctrl Pts',(0.00172324388897944,-0.0342804657353731,
-0.0103642464392609));
#40764=CARTESIAN_POINT('Ctrl Pts',(0.00169507978659403,-0.0342828329444561,
-0.0103378671573889));
#40765=CARTESIAN_POINT('Ctrl Pts',(0.0016508484689062,-0.0342865435359199,
-0.0102983203408101));
#40766=CARTESIAN_POINT('Ctrl Pts',(0.00163520732566602,-0.0342878544559937,
-0.0102846823249714));
#40767=CARTESIAN_POINT('Ctrl Pts',(0.00160554463223583,-0.0342903419211229,
-0.0102594615979602));
#40768=CARTESIAN_POINT('Ctrl Pts',(0.00159156337863107,-0.0342915146022978,
-0.0102478344500988));
#40769=CARTESIAN_POINT('Ctrl Pts',(0.00155272924514236,-0.0342947695793796,
-0.0102162492836129));
#40770=CARTESIAN_POINT('Ctrl Pts',(0.00152762036526226,-0.0342968716373137,
-0.0101966130894075));
#40771=CARTESIAN_POINT('Ctrl Pts',(0.0013900000871955,-0.0343083502253584,
-0.0100931670484586));
#40772=CARTESIAN_POINT('Ctrl Pts',(0.00127096671351649,-0.0343181124927171,
-0.0100184657936914));
#40773=CARTESIAN_POINT('Ctrl Pts',(0.00105454468871803,-0.0343349655484827,
-0.00990680122130327));
#40774=CARTESIAN_POINT('Ctrl Pts',(0.000959931804580723,-0.0343420692047618,
-0.0098651833277424));
#40775=CARTESIAN_POINT('Ctrl Pts',(0.000795326128183773,-0.0343538827462664,
-0.00980463899732866));
#40776=CARTESIAN_POINT('Ctrl Pts',(0.000726592220849624,-0.0343586643515419,
-0.0097826825447444));
#40777=CARTESIAN_POINT('Ctrl Pts',(0.000619092573203952,-0.0343659122134982,
-0.00975340247814949));
#40778=CARTESIAN_POINT('Ctrl Pts',(0.000580946012781767,-0.0343684407216593,
-0.00974397221660094));
#40779=CARTESIAN_POINT('Ctrl Pts',(0.000507803718102459,-0.0343732109216152,
-0.00972771003510177));
#40780=CARTESIAN_POINT('Ctrl Pts',(0.000472853504121802,-0.0343754568773819,
-0.00972071993818531));
#40781=CARTESIAN_POINT('Ctrl Pts',(0.00038938266601959,-0.0343807484171251,
-0.00970587434504571));
#40782=CARTESIAN_POINT('Ctrl Pts',(0.000340755663290763,-0.0343837732703598,
-0.00969869748261892));
#40783=CARTESIAN_POINT('Ctrl Pts',(0.000139091650495084,-0.0343961245379447,
-0.00967498522396319));
#40784=CARTESIAN_POINT('Ctrl Pts',(-1.50987334682496E-5,-0.0344050872759136,
-0.00967116483158575));
#40785=CARTESIAN_POINT('Ctrl Pts',(-0.000255412828585984,-0.0344191739210142,
-0.00968741544892404));
#40786=CARTESIAN_POINT('Ctrl Pts',(-0.00034178566742747,-0.0344242673917242,
-0.00969780170210138));
#40787=CARTESIAN_POINT('Ctrl Pts',(-0.000479858556137154,-0.0344326814562363,
-0.00972176149651209));
#40788=CARTESIAN_POINT('Ctrl Pts',(-0.000531972596123756,-0.0344359214382035,
-0.00973252868328095));
#40789=CARTESIAN_POINT('Ctrl Pts',(-0.000607322494260492,-0.0344407505742914,
-0.00975062142143391));
#40790=CARTESIAN_POINT('Ctrl Pts',(-0.00063086034652542,-0.0344422799766202,
-0.00975663743600475));
#40791=CARTESIAN_POINT('Ctrl Pts',(-0.00067408836425521,-0.0344451336154259,
-0.00976835977515811));
#40792=CARTESIAN_POINT('Ctrl Pts',(-0.000693802337755741,-0.0344464529108768,
-0.00977396687385435));
#40793=CARTESIAN_POINT('Ctrl Pts',(-0.000743847697447611,-0.0344498460801814,
-0.00978886838748338));
#40794=CARTESIAN_POINT('Ctrl Pts',(-0.000774074200212703,-0.0344519364745488,
-0.00979849861727811));
#40795=CARTESIAN_POINT('Ctrl Pts',(-0.000938846434620175,-0.0344635285834141,
-0.00985447076540195));
#40796=CARTESIAN_POINT('Ctrl Pts',(-0.00106942247211225,-0.0344734257907555,
-0.00991165807024596));
#40797=CARTESIAN_POINT('Ctrl Pts',(-0.00128262330724824,-0.0344901991988712,
-0.0100276076658194));
#40798=CARTESIAN_POINT('Ctrl Pts',(-0.00136786615463089,-0.0344970962365445,
-0.0100808528759677));
#40799=CARTESIAN_POINT('Ctrl Pts',(-0.00150714199903529,-0.0345085989724635,
-0.0101799831754404));
#40800=CARTESIAN_POINT('Ctrl Pts',(-0.00156285087249957,-0.0345132718793386,
-0.0102232977412049));
#40801=CARTESIAN_POINT('Ctrl Pts',(-0.00164617099831743,-0.0345203744222644,
-0.0102939345548012));
#40802=CARTESIAN_POINT('Ctrl Pts',(-0.00167510067844966,-0.0345228636463663,
-0.0103196380375233));
#40803=CARTESIAN_POINT('Ctrl Pts',(-0.00172916345075504,-0.0345275643055618,
-0.010369965562069));
#40804=CARTESIAN_POINT('Ctrl Pts',(-0.00175439601091676,-0.0345297798551923,
-0.0103944685599831));
#40805=CARTESIAN_POINT('Ctrl Pts',(-0.0018131129180065,-0.034534994059562,
-0.0104539459477249));
#40806=CARTESIAN_POINT('Ctrl Pts',(-0.00184611539207541,-0.0345379722942296,
-0.0104893771510893));
#40807=CARTESIAN_POINT('Ctrl Pts',(-0.00200734640564339,-0.034552819072591,
-0.0106728822769819));
#40808=CARTESIAN_POINT('Ctrl Pts',(-0.00211888257719614,-0.034564020584709,
-0.0108346963237527));
#40809=CARTESIAN_POINT('Ctrl Pts',(-0.00224218962433326,-0.0345794601199705,
-0.0110680544964574));
#40810=CARTESIAN_POINT('Ctrl Pts',(-0.00227151524080403,-0.0345834730057849,
-0.0111295024965632));
#40811=CARTESIAN_POINT('Ctrl Pts',(-0.00231633471788838,-0.0345903399083541,
-0.0112342085440858));
#40812=CARTESIAN_POINT('Ctrl Pts',(-0.0023332099359214,-0.0345931434377555,
-0.0112768359419936));
#40813=CARTESIAN_POINT('Ctrl Pts',(-0.00235669728837949,-0.0345974275935937,
-0.0113412898294623));
#40814=CARTESIAN_POINT('Ctrl Pts',(-0.00236419893875982,-0.0345988636594737,
-0.011362784063289));
#40815=CARTESIAN_POINT('Ctrl Pts',(-0.00237775615393995,-0.034601596563785,
-0.0114034039150018));
#40816=CARTESIAN_POINT('Ctrl Pts',(-0.00238387686492832,-0.0346028899322269,
-0.0114225051975321));
#40817=CARTESIAN_POINT('Ctrl Pts',(-0.00239926615506288,-0.0346063003020619,
-0.0114725978206038));
#40818=CARTESIAN_POINT('Ctrl Pts',(-0.00240816401635497,-0.034608435783106,
-0.0115036984121756));
#40819=CARTESIAN_POINT('Ctrl Pts',(-0.00245776525168612,-0.0346213505499705,
-0.0116907176672835));
#40820=CARTESIAN_POINT('Ctrl Pts',(-0.00248391695972193,-0.0346326314314633,
-0.0118500947594906));
#40821=CARTESIAN_POINT('Ctrl Pts',(-0.00250043972836219,-0.0346499134687464,
-0.0120999208994485));
#40822=CARTESIAN_POINT('Ctrl Pts',(-0.0025015570929233,-0.034656018967385,
-0.012189227968466));
#40823=CARTESIAN_POINT('Ctrl Pts',(-0.00249520360204096,-0.0346664103715346,
-0.0123439756892704));
#40824=CARTESIAN_POINT('Ctrl Pts',(-0.00248993102487983,-0.0346707468517693,
-0.0124094146122461));
#40825=CARTESIAN_POINT('Ctrl Pts',(-0.00247759270724932,-0.0346774501245827,
-0.0125119340443495));
#40826=CARTESIAN_POINT('Ctrl Pts',(-0.00247225347343839,-0.0346798672544537,
-0.0125491881345538));
#40827=CARTESIAN_POINT('Ctrl Pts',(-0.00246033089218614,-0.0346844824373551,
-0.0126208206288806));
#40828=CARTESIAN_POINT('Ctrl Pts',(-0.00245386274308029,-0.0346866834371846,
-0.0126552089642862));
#40829=CARTESIAN_POINT('Ctrl Pts',(-0.00243652122789473,-0.0346919419128282,
-0.0127378203036215));
#40830=CARTESIAN_POINT('Ctrl Pts',(-0.00242493529230502,-0.0346949767860079,
-0.0127858794660014));
#40831=CARTESIAN_POINT('Ctrl Pts',(-0.00237079009253734,-0.034707458746439,
-0.0129844380386911));
#40832=CARTESIAN_POINT('Ctrl Pts',(-0.00231558321647399,-0.0347165164253347,
-0.0131311200080114));
#40833=CARTESIAN_POINT('Ctrl Pts',(-0.00220725574056772,-0.0347308826707438,
-0.0133532466730315));
#40834=CARTESIAN_POINT('Ctrl Pts',(-0.00216307428721633,-0.0347361646808396,
-0.0134325716319483));
#40835=CARTESIAN_POINT('Ctrl Pts',(-0.00208559301979993,-0.034744849175532,
-0.0135554459739408));
#40836=CARTESIAN_POINT('Ctrl Pts',(-0.00205500448363599,-0.0347481590617163,
-0.0136006093793495));
#40837=CARTESIAN_POINT('Ctrl Pts',(-0.00200884604631038,-0.0347530455716281,
-0.0136641795636465));
#40838=CARTESIAN_POINT('Ctrl Pts',(-0.00199444686028728,-0.0347545560259131,
-0.0136834205863111));
#40839=CARTESIAN_POINT('Ctrl Pts',(-0.00196762282415661,-0.0347573509393794,
-0.013718207443292));
#40840=CARTESIAN_POINT('Ctrl Pts',(-0.00195528590681365,-0.0347586298962244,
-0.0137338176126994));
#40841=CARTESIAN_POINT('Ctrl Pts',(-0.00192413681585118,-0.0347618413164208,
-0.0137722785161897));
#40842=CARTESIAN_POINT('Ctrl Pts',(-0.00190510312411324,-0.0347637876592029,
-0.0137949449783718));
#40843=CARTESIAN_POINT('Ctrl Pts',(-0.00177957163424077,-0.0347764947088792,
-0.0139391568136953));
#40844=CARTESIAN_POINT('Ctrl Pts',(-0.001661909235318,-0.0347877922504112,
-0.0140504643252598));
#40845=CARTESIAN_POINT('Ctrl Pts',(-0.00146138727552628,-0.0348053310502105,
-0.0142063421343996));
#40846=CARTESIAN_POINT('Ctrl Pts',(-0.0013853439671957,-0.0348116592925567,
-0.0142589668650018));
#40847=CARTESIAN_POINT('Ctrl Pts',(-0.00124927825710126,-0.034822375789468,
-0.0143423752518866));
#40848=CARTESIAN_POINT('Ctrl Pts',(-0.00119060441940622,-0.0348268186772828,
-0.014375165912033));
#40849=CARTESIAN_POINT('Ctrl Pts',(-0.00109667301561655,-0.0348336589888785,
-0.0144227982865496));
#40850=CARTESIAN_POINT('Ctrl Pts',(-0.00106227844854788,-0.0348361091690161,
-0.0144392618418728));
#40851=CARTESIAN_POINT('Ctrl Pts',(-0.000995346579244765,-0.0348407773540105,
-0.014469437960957));
#40852=CARTESIAN_POINT('Ctrl Pts',(-0.000962869248225981,-0.0348429985456148,
-0.014483260593093));
#40853=CARTESIAN_POINT('Ctrl Pts',(-0.000883991768261539,-0.0348482948092699,
-0.0145148759477198));
#40854=CARTESIAN_POINT('Ctrl Pts',(-0.000837331887679209,-0.0348513474180882,
-0.0145319823697533));
#40855=CARTESIAN_POINT('Ctrl Pts',(-0.000658411478654128,-0.0348627929143484,
-0.0145915907667689));
#40856=CARTESIAN_POINT('Ctrl Pts',(-0.000523198611056358,-0.0348708971700031,
-0.0146244367467287));
#40857=CARTESIAN_POINT('Ctrl Pts',(-0.000286185470567523,-0.0348848647081733,
-0.0146614705853953));
#40858=CARTESIAN_POINT('Ctrl Pts',(-0.000185575366755641,-0.0348907277122509,
-0.0146709996317674));
#40859=CARTESIAN_POINT('Ctrl Pts',(-2.67850317323729E-5,-0.0349002124437143,
-0.0146763806565578));
#40860=CARTESIAN_POINT('Ctrl Pts',(3.11468071411945E-5,-0.0349037218853999,
-0.0146763299281411));
#40861=CARTESIAN_POINT('Ctrl Pts',(0.000113669102529428,-0.0349088548135483,
-0.0146733896095488));
#40862=CARTESIAN_POINT('Ctrl Pts',(0.00013830275365594,-0.0349104041086912,
-0.014672146656456));
#40863=CARTESIAN_POINT('Ctrl Pts',(0.000182810386925665,-0.0349132406345279,
-0.0146692401322728));
#40864=CARTESIAN_POINT('Ctrl Pts',(0.000202689664399399,-0.0349145215382621,
-0.0146677028817972));
#40865=CARTESIAN_POINT('Ctrl Pts',(0.000251617838013116,-0.0349177074934655,
-0.0146633299731633));
#40866=CARTESIAN_POINT('Ctrl Pts',(0.000280638455603433,-0.0349196255971715,
-0.014660223163764));
#40867=CARTESIAN_POINT('Ctrl Pts',(0.000473358686122774,-0.034932524723535,
-0.0146361718211618));
#40868=CARTESIAN_POINT('Ctrl Pts',(0.000634684462408655,-0.0349440698286065,
-0.0145995706082129));
#40869=CARTESIAN_POINT('Ctrl Pts',(0.000877230163152631,-0.0349617170482116,
-0.014518648403471));
#40870=CARTESIAN_POINT('Ctrl Pts',(0.000961623538307123,-0.0349679219629098,
-0.014485291346347));
#40871=CARTESIAN_POINT('Ctrl Pts',(0.00110430817594107,-0.0349784602585224,
-0.0144197127726436));
#40872=CARTESIAN_POINT('Ctrl Pts',(0.00116346999585728,-0.0349828457527284,
-0.0143896149681043));
#40873=CARTESIAN_POINT('Ctrl Pts',(0.00125445804353623,-0.0349896165763571,
-0.0143386693166316));
#40874=CARTESIAN_POINT('Ctrl Pts',(0.00128712287594484,-0.0349920531056776,
-0.014319390810375));
#40875=CARTESIAN_POINT('Ctrl Pts',(0.00134926931571013,-0.0349967039092671,
-0.0142807794191611));
#40876=CARTESIAN_POINT('Ctrl Pts',(0.00137880529019818,-0.0349989211753236,
-0.0142615517013248));
#40877=CARTESIAN_POINT('Ctrl Pts',(0.00144908291609466,-0.0350042202873406,
-0.0142136558653951));
#40878=CARTESIAN_POINT('Ctrl Pts',(0.00148939418751574,-0.0350072793149464,
-0.0141843816280446));
#40879=CARTESIAN_POINT('Ctrl Pts',(0.00164112625355554,-0.0350189125261958,
-0.0140671111735574));
#40880=CARTESIAN_POINT('Ctrl Pts',(0.00174585202455605,-0.0350271814890667,
-0.0139708900980514));
#40881=CARTESIAN_POINT('Ctrl Pts',(0.00190927271030721,-0.0350412409457035,
-0.0137928319113384));
#40882=CARTESIAN_POINT('Ctrl Pts',(0.00197223586600247,-0.0350470293269974,
-0.013715407077957));
#40883=CARTESIAN_POINT('Ctrl Pts',(0.00206397662559593,-0.035056414587606,
-0.0135877001800061));
#40884=CARTESIAN_POINT('Ctrl Pts',(0.00209592289932448,-0.0350599010652843,
-0.0135398244610649));
#40885=CARTESIAN_POINT('Ctrl Pts',(0.0021391025049762,-0.0350650034463417,
-0.0134700106846962));
#40886=CARTESIAN_POINT('Ctrl Pts',(0.00215170936165408,-0.0350665457260261,
-0.0134489399342518));
#40887=CARTESIAN_POINT('Ctrl Pts',(0.00217395034764177,-0.0350693703485281,
-0.0134104927094573));
#40888=CARTESIAN_POINT('Ctrl Pts',(0.00218369114775571,-0.0350706464090404,
-0.0133931813009595));
#40889=CARTESIAN_POINT('Ctrl Pts',(0.00220715464695614,-0.035073816863557,
-0.0133502938921162));
#40890=CARTESIAN_POINT('Ctrl Pts',(0.00222063971208916,-0.0350757241727262,
-0.013324592364697));
#40891=CARTESIAN_POINT('Ctrl Pts',(0.00230837111307789,-0.035088696793558,
-0.0131500629978429));
#40892=CARTESIAN_POINT('Ctrl Pts',(0.00236804885050966,-0.0351003376094888,
-0.0129943889731383));
#40893=CARTESIAN_POINT('Ctrl Pts',(0.00243557924095236,-0.0351180438994538,
-0.0127469014541685));
#40894=CARTESIAN_POINT('Ctrl Pts',(0.00245460364213349,-0.0351242181989909,
-0.0126586218181295));
#40895=CARTESIAN_POINT('Ctrl Pts',(0.00247922918477262,-0.0351347128073175,
-0.0125041793623759));
#40896=CARTESIAN_POINT('Ctrl Pts',(0.00248704867823636,-0.0351390846953079,
-0.0124384661183763));
#40897=CARTESIAN_POINT('Ctrl Pts',(0.00249523125352792,-0.0351458381559335,
-0.0123347700737067));
#40898=CARTESIAN_POINT('Ctrl Pts',(0.00249735195341803,-0.0351482706356105,
-0.0122969607783721));
#40899=CARTESIAN_POINT('Ctrl Pts',(0.00249953761635375,-0.0351524419826498,
-0.0122313718280536));
#40900=CARTESIAN_POINT('Ctrl Pts',(0.00249999999999506,-0.0351541924015739,
-0.0122036137105421));
#40901=CARTESIAN_POINT('Ctrl Pts',(0.0025,-0.0351559292844039,-0.0121758532870029));
#40902=CARTESIAN_POINT('Origin',(0.,-0.0397787743898723,-0.0121758532865581));
#40903=CARTESIAN_POINT('',(0.0025,-0.0362767501454997,-0.0121758532853817));
#40904=CARTESIAN_POINT('',(0.0025,-0.0361517921417372,-0.0121758532874351));
#40905=CARTESIAN_POINT('',(0.0025,-0.0397787743898723,-0.0121758532865581));
#40906=CARTESIAN_POINT('Ctrl Pts',(0.0025,-0.0362767501454997,-0.0121758532842053));
#40907=CARTESIAN_POINT('Ctrl Pts',(0.00250000000003539,-0.0362742798368169,
-0.012213451230406));
#40908=CARTESIAN_POINT('Ctrl Pts',(0.00249915183964461,-0.036271833829592,
-0.012251047489016));
#40909=CARTESIAN_POINT('Ctrl Pts',(0.00249586502308434,-0.0362671423022065,
-0.0123238451097689));
#40910=CARTESIAN_POINT('Ctrl Pts',(0.00249352892036452,-0.0362648943823479,
-0.0123590403969366));
#40911=CARTESIAN_POINT('Ctrl Pts',(0.00248713228653339,-0.0362602718961515,
-0.0124320080354312));
#40912=CARTESIAN_POINT('Ctrl Pts',(0.00248295402812442,-0.0362579014839455,
-0.0124697610933965));
#40913=CARTESIAN_POINT('Ctrl Pts',(0.00246909473769026,-0.0362514458748145,
-0.0125733409410715));
#40914=CARTESIAN_POINT('Ctrl Pts',(0.00245764382194434,-0.0362474140866701,
-0.0126389009802414));
#40915=CARTESIAN_POINT('Ctrl Pts',(0.00242436584690413,-0.0362380003315025,
-0.0127928893667135));
#40916=CARTESIAN_POINT('Ctrl Pts',(0.00240029697529597,-0.0362326761439758,
-0.0128807355787434));
#40917=CARTESIAN_POINT('Ctrl Pts',(0.00231943916770289,-0.0362177967447705,
-0.0131230862230201));
#40918=CARTESIAN_POINT('Ctrl Pts',(0.00225212683118324,-0.0362083448600165,
-0.0132735600266043));
#40919=CARTESIAN_POINT('Ctrl Pts',(0.00215602120519229,-0.0361964175200519,
-0.0134417241289305));
#40920=CARTESIAN_POINT('Ctrl Pts',(0.00214105616598809,-0.0361945944312331,
-0.0134668741033465));
#40921=CARTESIAN_POINT('Ctrl Pts',(0.00211516712920496,-0.0361914863336613,
-0.0135086942177314));
#40922=CARTESIAN_POINT('Ctrl Pts',(0.00210447930295857,-0.0361902152349852,
-0.0135255064880057));
#40923=CARTESIAN_POINT('Ctrl Pts',(0.00208019706886413,-0.036187351384371,
-0.0135627133196155));
#40924=CARTESIAN_POINT('Ctrl Pts',(0.00206650264918606,-0.0361857530052879,
-0.0135830374564709));
#40925=CARTESIAN_POINT('Ctrl Pts',(0.00201994219183921,-0.0361803815135176,
-0.0136499930560305));
#40926=CARTESIAN_POINT('Ctrl Pts',(0.00198578075629083,-0.0361765410478188,
-0.0136956981243938));
#40927=CARTESIAN_POINT('Ctrl Pts',(0.0018886691428119,-0.0361659647451942,
-0.0138167565458728));
#40928=CARTESIAN_POINT('Ctrl Pts',(0.00182279533272519,-0.0361591488909438,
-0.0138896358640562));
#40929=CARTESIAN_POINT('Ctrl Pts',(0.00165028818866548,-0.0361424075153059,
-0.0140592603107328));
#40930=CARTESIAN_POINT('Ctrl Pts',(0.00153924892779323,-0.036132553152112,
-0.0141510484031478));
#40931=CARTESIAN_POINT('Ctrl Pts',(0.00137993077660253,-0.0361197512957352,
-0.0142611045970387));
#40932=CARTESIAN_POINT('Ctrl Pts',(0.0013381012702414,-0.0361164994641448,
-0.0142881902689378));
#40933=CARTESIAN_POINT('Ctrl Pts',(0.00126532526474961,-0.0361110212028333,
-0.0143322845357926));
#40934=CARTESIAN_POINT('Ctrl Pts',(0.00123477829368026,-0.036108773319183,
-0.0143499201035272));
#40935=CARTESIAN_POINT('Ctrl Pts',(0.00117058220422291,-0.0361041508053646,
-0.0143851924752899));
#40936=CARTESIAN_POINT('Ctrl Pts',(0.00113688360032603,-0.0361017803314408,
-0.0144027206525344));
#40937=CARTESIAN_POINT('Ctrl Pts',(0.00104309055690354,-0.0360953242551307,
-0.0144488223243292));
#40938=CARTESIAN_POINT('Ctrl Pts',(0.000982233098250018,-0.0360912920756931,
-0.0144757761897292));
#40939=CARTESIAN_POINT('Ctrl Pts',(0.000835734274614518,-0.0360818770585062,
-0.0145337833658971));
#40940=CARTESIAN_POINT('Ctrl Pts',(0.000749329330506343,-0.0360765520245548,
-0.014562648820967));
#40941=CARTESIAN_POINT('Ctrl Pts',(0.000502973206773787,-0.0360616738905954,
-0.014630248183925));
#40942=CARTESIAN_POINT('Ctrl Pts',(0.000340520377472886,-0.0360522239677828,
-0.0146580034234385));
#40943=CARTESIAN_POINT('Ctrl Pts',(0.000147346921735369,-0.0360402986902551,
-0.0146716789118213));
#40944=CARTESIAN_POINT('Ctrl Pts',(0.000118118522926962,-0.0360384753567975,
-0.0146732328151908));
#40945=CARTESIAN_POINT('Ctrl Pts',(6.89599105717247E-5,-0.0360353669758907,
-0.0146749814319072));
#40946=CARTESIAN_POINT('Ctrl Pts',(4.90429610993991E-5,-0.0360340958447883,
-0.0146754515968087));
#40947=CARTESIAN_POINT('Ctrl Pts',(4.61775067226181E-6,-0.0360312320843629,
-0.0146759691206749));
#40948=CARTESIAN_POINT('Ctrl Pts',(-1.98876176675432E-5,-0.0360296338314264,
-0.0146758942623929));
#40949=CARTESIAN_POINT('Ctrl Pts',(-0.000101411416379767,-0.0360242634596296,
-0.0146744466026542));
#40950=CARTESIAN_POINT('Ctrl Pts',(-0.000158380604390681,-0.0360204240261645,
-0.0146714829554495));
#40951=CARTESIAN_POINT('Ctrl Pts',(-0.000312940110943239,-0.0360098519690956,
-0.0146581292788499));
#40952=CARTESIAN_POINT('Ctrl Pts',(-0.000410101335124589,-0.036003039393073,
-0.0146439378515311));
#40953=CARTESIAN_POINT('Ctrl Pts',(-0.000647037732160346,-0.0359862969155427,
-0.0145949508310812));
#40954=CARTESIAN_POINT('Ctrl Pts',(-0.000785141392585863,-0.0359764382009579,
-0.0145537207444458));
#40955=CARTESIAN_POINT('Ctrl Pts',(-0.000965278266506552,-0.035963632264159,
-0.0144825218564019));
#40956=CARTESIAN_POINT('Ctrl Pts',(-0.00101105504778219,-0.0359603804027877,
-0.0144628273296399));
#40957=CARTESIAN_POINT('Ctrl Pts',(-0.0010881806630824,-0.0359549020845861,
-0.0144268767500522));
#40958=CARTESIAN_POINT('Ctrl Pts',(-0.00111982828435481,-0.0359526541738741,
-0.014411301474992));
#40959=CARTESIAN_POINT('Ctrl Pts',(-0.00118485030569796,-0.0359480315930496,
-0.0143775735571073));
#40960=CARTESIAN_POINT('Ctrl Pts',(-0.00121816195650317,-0.0359456610794981,
-0.014359319357517));
#40961=CARTESIAN_POINT('Ctrl Pts',(-0.00130864788004727,-0.0359392048471741,
-0.0143070189622278));
#40962=CARTESIAN_POINT('Ctrl Pts',(-0.00136490058654355,-0.035935172554497,
-0.0142714376593029));
#40963=CARTESIAN_POINT('Ctrl Pts',(-0.00149460010370507,-0.0359257572057223,
-0.0141819582813932));
#40964=CARTESIAN_POINT('Ctrl Pts',(-0.00156665336028348,-0.0359204319588141,
-0.0141262084595669));
#40965=CARTESIAN_POINT('Ctrl Pts',(-0.00175986139117141,-0.0359055540571048,
-0.0139590867851481));
#40966=CARTESIAN_POINT('Ctrl Pts',(-0.00187328553768628,-0.035896104546535,
-0.0138395305970088));
#40967=CARTESIAN_POINT('Ctrl Pts',(-0.00199209951218874,-0.0358841796984165,
-0.013686613446243));
#40968=CARTESIAN_POINT('Ctrl Pts',(-0.00200964984411278,-0.0358823563041242,
-0.0136631878350116));
#40969=CARTESIAN_POINT('Ctrl Pts',(-0.00203844820398308,-0.0358792478622715,
-0.0136233082515866));
#40970=CARTESIAN_POINT('Ctrl Pts',(-0.00204991778651283,-0.0358779767328549,
-0.0136070185436724));
#40971=CARTESIAN_POINT('Ctrl Pts',(-0.00207505884702381,-0.0358751130527538,
-0.013570389492645));
#40972=CARTESIAN_POINT('Ctrl Pts',(-0.00208862718096007,-0.0358735148801182,
-0.0135499845896847));
#40973=CARTESIAN_POINT('Ctrl Pts',(-0.00213276806177369,-0.0358681450113287,
-0.0134814384070232));
#40974=CARTESIAN_POINT('Ctrl Pts',(-0.00216199154365445,-0.0358643060142999,
-0.0134324533434562));
#40975=CARTESIAN_POINT('Ctrl Pts',(-0.00223685756843397,-0.0358537357269175,
-0.0132966075180066));
#40976=CARTESIAN_POINT('Ctrl Pts',(-0.00227910406805199,-0.0358469245073912,
-0.0132079896077078));
#40977=CARTESIAN_POINT('Ctrl Pts',(-0.00237020292568441,-0.0358301812583886,
-0.0129838367762815));
#40978=CARTESIAN_POINT('Ctrl Pts',(-0.00241277157008422,-0.0358203204328534,
-0.0128461088212256));
#40979=CARTESIAN_POINT('Ctrl Pts',(-0.00245381173849764,-0.0358075125512418,
-0.0126567794304275));
#40980=CARTESIAN_POINT('Ctrl Pts',(-0.00246290864222748,-0.03580426070058,
-0.0126077833554056));
#40981=CARTESIAN_POINT('Ctrl Pts',(-0.00247593425567407,-0.0357987824382894,
-0.012523694199589));
#40982=CARTESIAN_POINT('Ctrl Pts',(-0.00248059492029272,-0.0357965345717058,
-0.0124887315081));
#40983=CARTESIAN_POINT('Ctrl Pts',(-0.00248873492754618,-0.0357919121216361,
-0.0124159381709361));
#40984=CARTESIAN_POINT('Ctrl Pts',(-0.00249209500409768,-0.035789541693736,
-0.0123781031826441));
#40985=CARTESIAN_POINT('Ctrl Pts',(-0.00249896535964855,-0.0357830858424721,
-0.0122738221572908));
#40986=CARTESIAN_POINT('Ctrl Pts',(-0.00250068764272604,-0.0357790538369016,
-0.012207288060753));
#40987=CARTESIAN_POINT('Ctrl Pts',(-0.00249847599515115,-0.0357696393713747,
-0.012049747895681));
#40988=CARTESIAN_POINT('Ctrl Pts',(-0.0024922287946029,-0.0357643147058106,
-0.0119588697962729));
#40989=CARTESIAN_POINT('Ctrl Pts',(-0.00246082382976147,-0.0357494359607489,
-0.0117053343378756));
#40990=CARTESIAN_POINT('Ctrl Pts',(-0.0024245586070309,-0.0357399851284444,
-0.0115445493743673));
#40991=CARTESIAN_POINT('Ctrl Pts',(-0.00236356409660929,-0.0357280588907157,
-0.0113607328619742));
#40992=CARTESIAN_POINT('Ctrl Pts',(-0.00235386028875028,-0.0357262356822809,
-0.0113331207579026));
#40993=CARTESIAN_POINT('Ctrl Pts',(-0.00233673996969483,-0.035723127472226,
-0.0112870095198973));
#40994=CARTESIAN_POINT('Ctrl Pts',(-0.00232958311796028,-0.0357218563846345,
-0.0112684176731279));
#40995=CARTESIAN_POINT('Ctrl Pts',(-0.00231312842250273,-0.0357189927008714,
-0.0112271502869139));
#40996=CARTESIAN_POINT('Ctrl Pts',(-0.00230371869008368,-0.0357173944807205,
-0.0112045240076565));
#40997=CARTESIAN_POINT('Ctrl Pts',(-0.00227130619100571,-0.0357120241559889,
-0.0111297075121592));
#40998=CARTESIAN_POINT('Ctrl Pts',(-0.00224685145687106,-0.03570818473348,
-0.0110781692014115));
#40999=CARTESIAN_POINT('Ctrl Pts',(-0.00217559331369965,-0.0356976127653918,
-0.010940369967551));
#41000=CARTESIAN_POINT('Ctrl Pts',(-0.0021254391976599,-0.0356908002626232,
-0.0108559546446451));
#41001=CARTESIAN_POINT('Ctrl Pts',(-0.0019898306636158,-0.0356740567926241,
-0.0106555675341315));
#41002=CARTESIAN_POINT('Ctrl Pts',(-0.00189906250214117,-0.0356641970266547,
-0.0105435952334376));
#41003=CARTESIAN_POINT('Ctrl Pts',(-0.00176456351026726,-0.0356513900662507,
-0.0104041880502071));
#41004=CARTESIAN_POINT('Ctrl Pts',(-0.00172890604034565,-0.0356481381518676,
-0.0103693742372358));
#41005=CARTESIAN_POINT('Ctrl Pts',(-0.00166627049053323,-0.0356426598097454,
-0.0103117753893409));
#41006=CARTESIAN_POINT('Ctrl Pts',(-0.00163980793770195,-0.0356404119257114,
-0.0102884545785825));
#41007=CARTESIAN_POINT('Ctrl Pts',(-0.00158384268185474,-0.0356357894651906,
-0.0102411996644271));
#41008=CARTESIAN_POINT('Ctrl Pts',(-0.00155427004074099,-0.0356334190437703,
-0.010217362245588));
#41009=CARTESIAN_POINT('Ctrl Pts',(-0.00147143279599603,-0.0356269632742615,
-0.0101536487678609));
#41010=CARTESIAN_POINT('Ctrl Pts',(-0.00141710052301308,-0.0356229313404055,
-0.0101152095135281));
#41011=CARTESIAN_POINT('Ctrl Pts',(-0.00128495398481078,-0.0356135170682256,
-0.0100294195715061));
#41012=CARTESIAN_POINT('Ctrl Pts',(-0.00120595941157477,-0.0356081925194984,
-0.00998406231443595));
#41013=CARTESIAN_POINT('Ctrl Pts',(-0.000977800071622283,-0.0355933138902623,
-0.00986913509743623));
#41014=CARTESIAN_POINT('Ctrl Pts',(-0.000824012815343339,-0.0355838630581899,
-0.00980983728253009));
#41015=CARTESIAN_POINT('Ctrl Pts',(-0.000637330312100262,-0.035571936837129,
-0.00975827875267805));
#41016=CARTESIAN_POINT('Ctrl Pts',(-0.000608986284533946,-0.035570113618245,
-0.00975098378753445));
#41017=CARTESIAN_POINT('Ctrl Pts',(-0.000561142507623278,-0.0355670053188939,
-0.00973956182958314));
#41018=CARTESIAN_POINT('Ctrl Pts',(-0.000541710140536657,-0.0355657341502486,
-0.0097351675080811));
#41019=CARTESIAN_POINT('Ctrl Pts',(-0.000498257495023248,-0.0355628700836613,
-0.00972588590340469));
#41020=CARTESIAN_POINT('Ctrl Pts',(-0.000474215893425129,-0.0355612715571717,
-0.00972111910811612));
#41021=CARTESIAN_POINT('Ctrl Pts',(-0.000393985943292631,-0.0355558994479853,
-0.00970643424078383));
#41022=CARTESIAN_POINT('Ctrl Pts',(-0.000337531478998195,-0.035552058503816,
-0.00969808677768321));
#41023=CARTESIAN_POINT('Ctrl Pts',(-0.000183288186653136,-0.0355414802182338,
-0.0096806489841735));
#41024=CARTESIAN_POINT('Ctrl Pts',(-8.51688573928007E-5,-0.0355346628439944,
-0.00967537648262942));
#41025=CARTESIAN_POINT('Ctrl Pts',(0.000156730123925787,-0.0355179238096782,
-0.009676634668049));
#41026=CARTESIAN_POINT('Ctrl Pts',(0.000300141709513632,-0.035508073266911,
-0.00968977547925869));
#41027=CARTESIAN_POINT('Ctrl Pts',(0.000490679471344255,-0.0354952749840797,
-0.00972397327593038));
#41028=CARTESIAN_POINT('Ctrl Pts',(0.000539443418733203,-0.0354920231967573,
-0.00973423839298679));
#41029=CARTESIAN_POINT('Ctrl Pts',(0.000622150905097135,-0.0354865448540481,
-0.00975424800276134));
#41030=CARTESIAN_POINT('Ctrl Pts',(0.000656252858193686,-0.0354842968498632,
-0.0097632662339819));
#41031=CARTESIAN_POINT('Ctrl Pts',(0.000726660925783979,-0.0354796739271464,
-0.00978348905775959));
#41032=CARTESIAN_POINT('Ctrl Pts',(0.000762925550661222,-0.0354773031686589,
-0.00979480571308437));
#41033=CARTESIAN_POINT('Ctrl Pts',(0.000861976948827517,-0.0354708457606185,
-0.00982821102320259));
#41034=CARTESIAN_POINT('Ctrl Pts',(0.000924163142924798,-0.0354668125653466,
-0.009851987540393));
#41035=CARTESIAN_POINT('Ctrl Pts',(0.00106902259016853,-0.035457394463237,
-0.0099141098788852));
#41036=CARTESIAN_POINT('Ctrl Pts',(0.00115069444666908,-0.0354520674139331,
-0.00995454822799694));
#41037=CARTESIAN_POINT('Ctrl Pts',(0.00137306282325345,-0.0354371918028122,
-0.0100802127853202));
#41038=CARTESIAN_POINT('Ctrl Pts',(0.00150780583625054,-0.0354277460887824,
-0.0101749736609747));
#41039=CARTESIAN_POINT('Ctrl Pts',(0.00165443749127167,-0.0354158252131631,
-0.0103013683383368));
#41040=CARTESIAN_POINT('Ctrl Pts',(0.0016762756203987,-0.0354140013013983,
-0.010320871586817));
#41041=CARTESIAN_POINT('Ctrl Pts',(0.00171239035777612,-0.0354108923045119,
-0.0103542835675033));
#41042=CARTESIAN_POINT('Ctrl Pts',(0.00172685190792062,-0.0354096211519043,
-0.0103679872971774));
#41043=CARTESIAN_POINT('Ctrl Pts',(0.00175872769575892,-0.0354067579332773,
-0.0103989241994791));
#41044=CARTESIAN_POINT('Ctrl Pts',(0.00177605393037219,-0.0354051602564452,
-0.0104162418478012));
#41045=CARTESIAN_POINT('Ctrl Pts',(0.00183282929455883,-0.035399793802733,
-0.010474681950104));
#41046=CARTESIAN_POINT('Ctrl Pts',(0.00187112462385743,-0.0353959578255314,
-0.0105168961417131));
#41047=CARTESIAN_POINT('Ctrl Pts',(0.00197124035714185,-0.0353853998316306,
-0.0106351368726826));
#41048=CARTESIAN_POINT('Ctrl Pts',(0.00203008880682895,-0.0353785980558163,
-0.0107135489551092));
#41049=CARTESIAN_POINT('Ctrl Pts',(0.002163746215651,-0.0353618501330064,
-0.0109153145172044));
#41050=CARTESIAN_POINT('Ctrl Pts',(0.00223278743846951,-0.0353519752945608,
-0.0110420870544471));
#41051=CARTESIAN_POINT('Ctrl Pts',(0.00231049099123751,-0.0353391544457537,
-0.0112197605476901));
#41052=CARTESIAN_POINT('Ctrl Pts',(0.00232908545824077,-0.035335902625978,
-0.0112659942674584));
#41053=CARTESIAN_POINT('Ctrl Pts',(0.00235846134782538,-0.0353304245824456,
-0.0113458511149229));
#41054=CARTESIAN_POINT('Ctrl Pts',(0.00236993463776702,-0.0353281768989369,
-0.0113792018272071));
#41055=CARTESIAN_POINT('Ctrl Pts',(0.00239228894420847,-0.0353235549985508,
-0.0114489451401146));
#41056=CARTESIAN_POINT('Ctrl Pts',(0.00240305403993767,-0.0353211849330625,
-0.011485365512862));
#41057=CARTESIAN_POINT('Ctrl Pts',(0.00243037926343884,-0.0353147307057141,
-0.0115862096129212));
#41058=CARTESIAN_POINT('Ctrl Pts',(0.00244520534939592,-0.0353106999261971,
-0.0116510724868956));
#41059=CARTESIAN_POINT('Ctrl Pts',(0.00247414595144908,-0.0353012892458527,
-0.0118058820223453));
#41060=CARTESIAN_POINT('Ctrl Pts',(0.00248597059139312,-0.0352959670760043,
-0.0118961597482336));
#41061=CARTESIAN_POINT('Ctrl Pts',(0.00249761723666546,-0.0352869934099935,
-0.0120498004510097));
#41062=CARTESIAN_POINT('Ctrl Pts',(0.0025,-0.0352833345293618,-0.0121128350691632));
#41063=CARTESIAN_POINT('Ctrl Pts',(0.0025,-0.0352796511099541,-0.0121758532865581));
#41064=CARTESIAN_POINT('Ctrl Pts',(0.0025,-0.0351559292844039,-0.0121758532870029));
#41065=CARTESIAN_POINT('Ctrl Pts',(0.00250000000000132,-0.0351563949541079,
-0.0121684105349698));
#41066=CARTESIAN_POINT('Ctrl Pts',(0.00249996676327267,-0.0351568596530242,
-0.0121609676173145));
#41067=CARTESIAN_POINT('Ctrl Pts',(0.00249945563224408,-0.0351604252519763,
-0.0121037414352842));
#41068=CARTESIAN_POINT('Ctrl Pts',(0.00249752398131161,-0.0351634828049984,
-0.0120539802566494));
#41069=CARTESIAN_POINT('Ctrl Pts',(0.00248417584769355,-0.0351752826153707,
-0.0118599116843188));
#41070=CARTESIAN_POINT('Ctrl Pts',(0.00246172365287784,-0.0351837048321569,
-0.0117166472795673));
#41071=CARTESIAN_POINT('Ctrl Pts',(0.00240359142092288,-0.0351978012676244,
-0.011481397620577));
#41072=CARTESIAN_POINT('Ctrl Pts',(0.00237466026504458,-0.035203470028303,
-0.0113881305486763));
#41073=CARTESIAN_POINT('Ctrl Pts',(0.00232036759136451,-0.0352126903552338,
-0.0112435843160812));
#41074=CARTESIAN_POINT('Ctrl Pts',(0.00229857248667062,-0.0352161360438733,
-0.0111910717120396));
#41075=CARTESIAN_POINT('Ctrl Pts',(0.00226487208409575,-0.0352211894268369,
-0.0111171029889639));
#41076=CARTESIAN_POINT('Ctrl Pts',(0.00225441016863284,-0.0352227253709667,
-0.01109500527027));
#41077=CARTESIAN_POINT('Ctrl Pts',(0.00223485120237666,-0.0352255454814689,
-0.0110552124706219));
#41078=CARTESIAN_POINT('Ctrl Pts',(0.0022258641541744,-0.0352268235574635,
-0.0110374665313088));
#41079=CARTESIAN_POINT('Ctrl Pts',(0.0022031559284935,-0.0352300088783028,
-0.0109939236615293));
#41080=CARTESIAN_POINT('Ctrl Pts',(0.00218919286850779,-0.03523192932776,
-0.0109682572885822));
#41081=CARTESIAN_POINT('Ctrl Pts',(0.00209352430275947,-0.0352448140888636,
-0.0107995170592295));
#41082=CARTESIAN_POINT('Ctrl Pts',(0.00199830057539474,-0.0352563406702599,
-0.0106645841139374));
#41083=CARTESIAN_POINT('Ctrl Pts',(0.00183102350259616,-0.0352739873557177,
-0.0104712665222593));
#41084=CARTESIAN_POINT('Ctrl Pts',(0.00176783438139355,-0.0352802088729795,
-0.01040581741614));
#41085=CARTESIAN_POINT('Ctrl Pts',(0.00165251240364309,-0.0352907716238003,
-0.0102987223685377));
#41086=CARTESIAN_POINT('Ctrl Pts',(0.00160202124309784,-0.0352951653377304,
-0.0102554504786439));
#41087=CARTESIAN_POINT('Ctrl Pts',(0.00152008518961002,-0.0353019458751378,
-0.0101907132115773));
#41088=CARTESIAN_POINT('Ctrl Pts',(0.00148977592009498,-0.0353043841466608,
-0.0101678672158307));
#41089=CARTESIAN_POINT('Ctrl Pts',(0.00143034112872585,-0.0353090367980789,
-0.0101251543753234));
#41090=CARTESIAN_POINT('Ctrl Pts',(0.00140129271959162,-0.0353112542025186,
-0.0101051962220878));
#41091=CARTESIAN_POINT('Ctrl Pts',(0.00133021990096038,-0.0353165516001159,
-0.0100585454518144));
#41092=CARTESIAN_POINT('Ctrl Pts',(0.00128780065812075,-0.0353196088451457,
-0.0100324803810824));
#41093=CARTESIAN_POINT('Ctrl Pts',(0.00112127729252926,-0.0353312577349212,
-0.00993688767448848));
#41094=CARTESIAN_POINT('Ctrl Pts',(0.000992104147321659,-0.0353395429594198,
-0.0098767308884868));
#41095=CARTESIAN_POINT('Ctrl Pts',(0.000765359196507202,-0.0353535905513078,
-0.00979382437928423));
#41096=CARTESIAN_POINT('Ctrl Pts',(0.000670272116732628,-0.035359350249661,
-0.00976534094291586));
#41097=CARTESIAN_POINT('Ctrl Pts',(0.000517919142949801,-0.0353686952236813,
-0.00972941706779019));
#41098=CARTESIAN_POINT('Ctrl Pts',(0.000461655641987034,-0.0353721714424997,
-0.00971817887930309));
#41099=CARTESIAN_POINT('Ctrl Pts',(0.000380842526593096,-0.0353772623090306,
-0.00970490989068861));
#41100=CARTESIAN_POINT('Ctrl Pts',(0.000356568932833508,-0.0353788039382319,
-0.00970129054060954));
#41101=CARTESIAN_POINT('Ctrl Pts',(0.000312527065379535,-0.0353816299620092,
-0.00969538504345239));
#41102=CARTESIAN_POINT('Ctrl Pts',(0.000292778126937727,-0.0353829081395409,
-0.00969297657919998));
#41103=CARTESIAN_POINT('Ctrl Pts',(0.000244031635842235,-0.0353860887645381,
-0.00968762137815184));
#41104=CARTESIAN_POINT('Ctrl Pts',(0.000215008280882003,-0.0353880042806885,
-0.00968494567372648));
#41105=CARTESIAN_POINT('Ctrl Pts',(2.10568285708737E-5,-0.0354009219605038,
-0.00967047978151122));
#41106=CARTESIAN_POINT('Ctrl Pts',(-0.000144635598741956,-0.0354124912163048,
-0.00967457069291537));
#41107=CARTESIAN_POINT('Ctrl Pts',(-0.000398625926296231,-0.0354301576349027,
-0.00970617534028667));
#41108=CARTESIAN_POINT('Ctrl Pts',(-0.000487882207660514,-0.0354363590074527,
-0.00972224675691553));
#41109=CARTESIAN_POINT('Ctrl Pts',(-0.000640618188577008,-0.0354468925933814,
-0.00975841501196895));
#41110=CARTESIAN_POINT('Ctrl Pts',(-0.000704532122699878,-0.0354512768861299,
-0.00977626264724338));
#41111=CARTESIAN_POINT('Ctrl Pts',(-0.000803747658189741,-0.0354580459161638,
-0.00980827495116807));
#41112=CARTESIAN_POINT('Ctrl Pts',(-0.00083956193405003,-0.0354604818534231,
-0.00982073683892129));
#41113=CARTESIAN_POINT('Ctrl Pts',(-0.000908079630434014,-0.0354651314129944,
-0.00984633995201143));
#41114=CARTESIAN_POINT('Ctrl Pts',(-0.000940815643358329,-0.0354673480290801,
-0.0098593673462336));
#41115=CARTESIAN_POINT('Ctrl Pts',(-0.00101912801234922,-0.0354726454485083,
-0.00989246609554668));
#41116=CARTESIAN_POINT('Ctrl Pts',(-0.00106440209258983,-0.0354757034503298,
-0.0099132159646103));
#41117=CARTESIAN_POINT('Ctrl Pts',(-0.00123708373798894,-0.0354873919919925,
-0.00999869009301758));
#41118=CARTESIAN_POINT('Ctrl Pts',(-0.00135947302964417,-0.0354957125265262,
-0.0100729378051985));
#41119=CARTESIAN_POINT('Ctrl Pts',(-0.00155467588182124,-0.0355097771927162,
-0.0102155586805669));
#41120=CARTESIAN_POINT('Ctrl Pts',(-0.00163096160039099,-0.0355155180835879,
-0.0102785566945272));
#41121=CARTESIAN_POINT('Ctrl Pts',(-0.0017452270509599,-0.035524837603733,
-0.0103849146161293));
#41122=CARTESIAN_POINT('Ctrl Pts',(-0.00178578494218066,-0.0355283077406332,
-0.0104253533759202));
#41123=CARTESIAN_POINT('Ctrl Pts',(-0.00184167326752474,-0.0355333908288594,
-0.0104850426232389));
#41124=CARTESIAN_POINT('Ctrl Pts',(-0.0018581658477028,-0.0355349309641914,
-0.0105031845512746));
#41125=CARTESIAN_POINT('Ctrl Pts',(-0.00188754741012638,-0.0355377548397322,
-0.0105364752802042));
#41126=CARTESIAN_POINT('Ctrl Pts',(-0.00190052694648923,-0.0355390323817366,
-0.0105515402925441));
#41127=CARTESIAN_POINT('Ctrl Pts',(-0.00193207562071363,-0.035542211483126,
-0.0105890538428911));
#41128=CARTESIAN_POINT('Ctrl Pts',(-0.00195043406240697,-0.0355441261073228,
-0.0106116744367565));
#41129=CARTESIAN_POINT('Ctrl Pts',(-0.00207039464085095,-0.0355570500151963,
-0.0107648815084589));
#41130=CARTESIAN_POINT('Ctrl Pts',(-0.00215920659424629,-0.0355686273779125,
-0.0109049494785052));
#41131=CARTESIAN_POINT('Ctrl Pts',(-0.00227422460617676,-0.0355862994637495,
-0.0111336877263112));
#41132=CARTESIAN_POINT('Ctrl Pts',(-0.00231049485649044,-0.0355924988893119,
-0.0112167795692172));
#41133=CARTESIAN_POINT('Ctrl Pts',(-0.00236536582511525,-0.0356030297507572,
-0.0113637927026489));
#41134=CARTESIAN_POINT('Ctrl Pts',(-0.00238607533183011,-0.0356074132363114,
-0.0114268248076432));
#41135=CARTESIAN_POINT('Ctrl Pts',(-0.0024146460863224,-0.0356141811957685,
-0.0115270687056863));
#41136=CARTESIAN_POINT('Ctrl Pts',(-0.00242420686796078,-0.0356166168562833,
-0.0115637597752124));
#41137=CARTESIAN_POINT('Ctrl Pts',(-0.00244103429876844,-0.0356212659311039,
-0.0116349352548848));
#41138=CARTESIAN_POINT('Ctrl Pts',(-0.00244841362374765,-0.0356234823380514,
-0.0116693834580102));
#41139=CARTESIAN_POINT('Ctrl Pts',(-0.00246445984132205,-0.0356287793193002,
-0.0117528682945953));
#41140=CARTESIAN_POINT('Ctrl Pts',(-0.00247239480275534,-0.0356318370935566,
-0.011802031072305));
#41141=CARTESIAN_POINT('Ctrl Pts',(-0.00249743895460319,-0.0356435434805143,
-0.01199337135211));
#41142=CARTESIAN_POINT('Ctrl Pts',(-0.00250379135426237,-0.0356518805237512,
-0.0121366800145431));
#41143=CARTESIAN_POINT('Ctrl Pts',(-0.00249374192974491,-0.0356659482009488,
-0.0123782737762828));
#41144=CARTESIAN_POINT('Ctrl Pts',(-0.00248381899150705,-0.0356716752257176,
-0.0124764595943251));
#41145=CARTESIAN_POINT('Ctrl Pts',(-0.00245902330571661,-0.0356809755889593,
-0.0126302471783816));
#41146=CARTESIAN_POINT('Ctrl Pts',(-0.00244798839926214,-0.0356844409758035,
-0.0126863640542578));
#41147=CARTESIAN_POINT('Ctrl Pts',(-0.00242949036189544,-0.0356895184138586,
-0.0127659186665383));
#41148=CARTESIAN_POINT('Ctrl Pts',(-0.00242358972925878,-0.0356910578760154,
-0.0127897044799358));
#41149=CARTESIAN_POINT('Ctrl Pts',(-0.00241226803343798,-0.0356938813899903,
-0.012832632243649));
#41150=CARTESIAN_POINT('Ctrl Pts',(-0.00240696653778475,-0.035695159266899,
-0.0128518027321222));
#41151=CARTESIAN_POINT('Ctrl Pts',(-0.00239333009357419,-0.0356983405009161,
-0.0128989171330397));
#41152=CARTESIAN_POINT('Ctrl Pts',(-0.00238473416433873,-0.035700256961596,
-0.0129267814158173));
#41153=CARTESIAN_POINT('Ctrl Pts',(-0.00232419002330921,-0.0357131684996653,
-0.0131115047219413));
#41154=CARTESIAN_POINT('Ctrl Pts',(-0.00225729013692594,-0.0357247297952758,
-0.0132630231864623));
#41155=CARTESIAN_POINT('Ctrl Pts',(-0.00213128747458824,-0.0357423933445719,
-0.0134857528895373));
#41156=CARTESIAN_POINT('Ctrl Pts',(-0.00208237238712282,-0.0357485992660666,
-0.0135621976802002));
#41157=CARTESIAN_POINT('Ctrl Pts',(-0.00199065437542108,-0.0357591394836901,
-0.0136896890876594));
#41158=CARTESIAN_POINT('Ctrl Pts',(-0.0019497689239674,-0.0357635259532333,
-0.0137419969878766));
#41159=CARTESIAN_POINT('Ctrl Pts',(-0.0018823230063378,-0.0357702976110055,
-0.0138215440671646));
#41160=CARTESIAN_POINT('Ctrl Pts',(-0.00185714294379729,-0.03577273405962,
-0.0138499077608157));
#41161=CARTESIAN_POINT('Ctrl Pts',(-0.00180734432003623,-0.0357773842517837,
-0.0139034955005437));
#41162=CARTESIAN_POINT('Ctrl Pts',(-0.00178281876809443,-0.0357796009967991,
-0.0139287932588103));
#41163=CARTESIAN_POINT('Ctrl Pts',(-0.00172236512650647,-0.03578489824693,
-0.0139885686002121));
#41164=CARTESIAN_POINT('Ctrl Pts',(-0.00168592529284494,-0.0357879559651933,
-0.014022508327387));
#41165=CARTESIAN_POINT('Ctrl Pts',(-0.00154111465971355,-0.0357996412149966,
-0.0141495215312965));
#41166=CARTESIAN_POINT('Ctrl Pts',(-0.00142585847314525,-0.0358079590661767,
-0.0142343316172787));
#41167=CARTESIAN_POINT('Ctrl Pts',(-0.00121965447240412,-0.0358220203089604,
-0.0143603925353188));
#41168=CARTESIAN_POINT('Ctrl Pts',(-0.00113234839836963,-0.0358277604684135,
-0.014406896524174));
#41169=CARTESIAN_POINT('Ctrl Pts',(-0.00099048595430555,-0.0358370788396377,
-0.0144719838534337));
#41170=CARTESIAN_POINT('Ctrl Pts',(-0.00093764677714252,-0.0358405486336832,
-0.0144940628422152));
#41171=CARTESIAN_POINT('Ctrl Pts',(-0.000861165423813789,-0.0358456314624628,
-0.0145229781923017));
#41172=CARTESIAN_POINT('Ctrl Pts',(-0.000838104951708319,-0.035847171721613,
-0.0145313110323709));
#41173=CARTESIAN_POINT('Ctrl Pts',(-0.000796121931715857,-0.0358499960293268,
-0.0145457869419733));
#41174=CARTESIAN_POINT('Ctrl Pts',(-0.000777242311018188,-0.0358512738843371,
-0.0145520456093274));
#41175=CARTESIAN_POINT('Ctrl Pts',(-0.000730516408837936,-0.0358544542942129,
-0.0145669190184823));
#41176=CARTESIAN_POINT('Ctrl Pts',(-0.000702591252722598,-0.035856369931203,
-0.0145752729907218));
#41177=CARTESIAN_POINT('Ctrl Pts',(-0.000515325747385473,-0.0358692869605858,
-0.0146277453429846));
#41178=CARTESIAN_POINT('Ctrl Pts',(-0.000352101138185912,-0.035880855383117,
-0.0146564488502266));
#41179=CARTESIAN_POINT('Ctrl Pts',(-9.68669164623152E-5,-0.0358985223478047,
-0.0146756196352032));
#41180=CARTESIAN_POINT('Ctrl Pts',(-6.17677745407344E-6,-0.0359047250243374,
-0.0146774885736422));
#41181=CARTESIAN_POINT('Ctrl Pts',(0.00015072089068347,-0.0359152605467985,
-0.0146721873896958));
#41182=CARTESIAN_POINT('Ctrl Pts',(0.000216910013586982,-0.0359196455022932,
-0.01466730909817));
#41183=CARTESIAN_POINT('Ctrl Pts',(0.000320504201698942,-0.0359264153028654,
-0.0146555134792521));
#41184=CARTESIAN_POINT('Ctrl Pts',(0.000358075737165516,-0.0359288513690887,
-0.0146503673058786));
#41185=CARTESIAN_POINT('Ctrl Pts',(0.00043030114824313,-0.0359335010444259,
-0.0146387950019428));
#41186=CARTESIAN_POINT('Ctrl Pts',(0.000464964516071402,-0.0359357176501853,
-0.0146324869926315));
#41187=CARTESIAN_POINT('Ctrl Pts',(0.000548266533117582,-0.0359410148640837,
-0.014615501303359));
#41188=CARTESIAN_POINT('Ctrl Pts',(0.000596742851522922,-0.0359440726772972,
-0.0146040989705843));
#41189=CARTESIAN_POINT('Ctrl Pts',(0.000782961132498546,-0.0359557650983978,
-0.0145543835955347));
#41190=CARTESIAN_POINT('Ctrl Pts',(0.000917660488111485,-0.0359640893766176,
-0.0145057327874343));
#41191=CARTESIAN_POINT('Ctrl Pts',(0.00113715701687981,-0.0359781534616333,
-0.0144044470026523));
#41192=CARTESIAN_POINT('Ctrl Pts',(0.00122430588180622,-0.0359838899235319,
-0.0143577857336156));
#41193=CARTESIAN_POINT('Ctrl Pts',(0.00135722981399037,-0.0359932032659589,
-0.0142761396728781));
#41194=CARTESIAN_POINT('Ctrl Pts',(0.00140495166513847,-0.0359966718463788,
-0.0142445208550007));
#41195=CARTESIAN_POINT('Ctrl Pts',(0.00147150257022165,-0.0360017531454617,
-0.0141970611387035));
#41196=CARTESIAN_POINT('Ctrl Pts',(0.00149125094538757,-0.0360032931326325,
-0.0141825350016581));
#41197=CARTESIAN_POINT('Ctrl Pts',(0.00152662888027616,-0.0360061170838302,
-0.0141557017332193));
#41198=CARTESIAN_POINT('Ctrl Pts',(0.00154233056835375,-0.0360073948585694,
-0.014143494496561));
#41199=CARTESIAN_POINT('Ctrl Pts',(0.00158068010730316,-0.0360105751504573,
-0.0141129387059224));
#41200=CARTESIAN_POINT('Ctrl Pts',(0.00160315512244763,-0.0360124907513033,
-0.0140943795449346));
#41201=CARTESIAN_POINT('Ctrl Pts',(0.00175092877958355,-0.0360254080664405,
-0.0139679429082744));
#41202=CARTESIAN_POINT('Ctrl Pts',(0.00186557731151984,-0.0360369768609485,
-0.0138482624403817));
#41203=CARTESIAN_POINT('Ctrl Pts',(0.00202348288254117,-0.0360546442363876,
-0.0136468162847873));
#41204=CARTESIAN_POINT('Ctrl Pts',(0.00207548166271109,-0.0360608469707916,
-0.0135724896926553));
#41205=CARTESIAN_POINT('Ctrl Pts',(0.00215834924311046,-0.0360713825906825,
-0.013439154265334));
#41206=CARTESIAN_POINT('Ctrl Pts',(0.00219111239163233,-0.036075767587884,
-0.0133814355439498));
#41207=CARTESIAN_POINT('Ctrl Pts',(0.00223893312397356,-0.0360825374315269,
-0.0132887845890405));
#41208=CARTESIAN_POINT('Ctrl Pts',(0.00225555521490443,-0.0360849735010654,
-0.0132546992167139));
#41209=CARTESIAN_POINT('Ctrl Pts',(0.0022861127219348,-0.0360896231694473,
-0.0131882413457559));
#41210=CARTESIAN_POINT('Ctrl Pts',(0.00230015158766458,-0.0360918397652216,
-0.0131559266659638));
#41211=CARTESIAN_POINT('Ctrl Pts',(0.00233237146583091,-0.0360971369383572,
-0.0130772532706332));
#41212=CARTESIAN_POINT('Ctrl Pts',(0.00234986000222167,-0.0361001947216171,
-0.0130306263859647));
#41213=CARTESIAN_POINT('Ctrl Pts',(0.0024121387699056,-0.0361118893788775,
-0.0128481863567145));
#41214=CARTESIAN_POINT('Ctrl Pts',(0.00244663952748377,-0.0361202157318824,
-0.012709149564717));
#41215=CARTESIAN_POINT('Ctrl Pts',(0.00248455077588863,-0.0361342800876291,
-0.0124703984729227));
#41216=CARTESIAN_POINT('Ctrl Pts',(0.00249424391780315,-0.0361400146975396,
-0.0123720541215961));
#41217=CARTESIAN_POINT('Ctrl Pts',(0.00249936542594825,-0.0361478511771709,
-0.0122408961514366));
#41218=CARTESIAN_POINT('Ctrl Pts',(0.00249999999997718,-0.0361498099347429,
-0.0122083743989067));
#41219=CARTESIAN_POINT('Ctrl Pts',(0.0025,-0.0361517921417372,-0.0121758532883121));
#41220=CARTESIAN_POINT('Origin',(0.,-0.0397787743898723,-0.0121758532865581));
#41221=CARTESIAN_POINT('',(0.0025,-0.0372809459012698,-0.0121758532870403));
#41222=CARTESIAN_POINT('',(0.0025,-0.0371551761478877,-0.0121758532865581));
#41223=CARTESIAN_POINT('',(0.0025,-0.0397787743898723,-0.0121758532865581));
#41224=CARTESIAN_POINT('Ctrl Pts',(0.0025,-0.0372809459012698,-0.0121758532875225));
#41225=CARTESIAN_POINT('Ctrl Pts',(0.00249999999999826,-0.0372806546811033,
-0.0121803528786627));
#41226=CARTESIAN_POINT('Ctrl Pts',(0.00249998785222117,-0.0372803628467704,
-0.0121848524327188));
#41227=CARTESIAN_POINT('Ctrl Pts',(0.00249979491297204,-0.0372780405125425,
-0.012220585046315));
#41228=CARTESIAN_POINT('Ctrl Pts',(0.00249904097763098,-0.0372759821757314,
-0.0122518106556588));
#41229=CARTESIAN_POINT('Ctrl Pts',(0.00249141738934109,-0.037264133550365,
-0.0124295042276286));
#41230=CARTESIAN_POINT('Ctrl Pts',(0.00247225739487052,-0.0372539157741499,
-0.0125751496023748));
#41231=CARTESIAN_POINT('Ctrl Pts',(0.00241897661960846,-0.0372369329524492,
-0.0128148728429871));
#41232=CARTESIAN_POINT('Ctrl Pts',(0.00239178608095105,-0.0372301350622787,
-0.0129101256705615));
#41233=CARTESIAN_POINT('Ctrl Pts',(0.0023358517734136,-0.0372187671655393,
-0.0130695494378505));
#41234=CARTESIAN_POINT('Ctrl Pts',(0.00230992232089387,-0.037214131712778,
-0.0131345798746825));
#41235=CARTESIAN_POINT('Ctrl Pts',(0.00226553425745776,-0.0372070763977103,
-0.0132336053574228));
#41236=CARTESIAN_POINT('Ctrl Pts',(0.0022489606948044,-0.0372045976597058,
-0.0132684012130409));
#41237=CARTESIAN_POINT('Ctrl Pts',(0.0022157801777306,-0.037199913974546,
-0.0133341054345397));
#41238=CARTESIAN_POINT('Ctrl Pts',(0.00219931429537779,-0.037197704980789,
-0.0133650743164107));
#41239=CARTESIAN_POINT('Ctrl Pts',(0.00215861569823421,-0.0371925021572555,
-0.0134378813613273));
#41240=CARTESIAN_POINT('Ctrl Pts',(0.00213380997413948,-0.0371895288001224,
-0.0134793838947029));
#41241=CARTESIAN_POINT('Ctrl Pts',(0.00200365535702628,-0.0371748198049943,
-0.0136834632903798));
#41242=CARTESIAN_POINT('Ctrl Pts',(0.00188087033881847,-0.0371637343348594,
-0.0138341214708739));
#41243=CARTESIAN_POINT('Ctrl Pts',(0.00169308628104789,-0.0371484181459929,
-0.0140165306544881));
#41244=CARTESIAN_POINT('Ctrl Pts',(0.00164234107884988,-0.037144404425019,
-0.014061946896773));
#41245=CARTESIAN_POINT('Ctrl Pts',(0.00155445320821453,-0.0371375386082975,
-0.0141343664989117));
#41246=CARTESIAN_POINT('Ctrl Pts',(0.00151830554132067,-0.0371347369840929,
-0.0141625204727291));
#41247=CARTESIAN_POINT('Ctrl Pts',(0.00146306701981392,-0.0371304547336446,
-0.0142031552592165));
#41248=CARTESIAN_POINT('Ctrl Pts',(0.00144454398665757,-0.0371290186029304,
-0.0142163951200463));
#41249=CARTESIAN_POINT('Ctrl Pts',(0.00140924341705303,-0.0371262760850975,
-0.0142409056844498));
#41250=CARTESIAN_POINT('Ctrl Pts',(0.0013925054517009,-0.037124973005608,
-0.0142522291851827));
#41251=CARTESIAN_POINT('Ctrl Pts',(0.00134826588070653,-0.0371215250172291,
-0.0142813825125378));
#41252=CARTESIAN_POINT('Ctrl Pts',(0.00132054821017414,-0.0371193611075894,
-0.0142988762246454));
#41253=CARTESIAN_POINT('Ctrl Pts',(0.00119218362771139,-0.0371093504729853,
-0.0143764058496733));
#41254=CARTESIAN_POINT('Ctrl Pts',(0.00108774217604955,-0.0371012422149654,
-0.014429860032106));
#41255=CARTESIAN_POINT('Ctrl Pts',(0.000873866457429997,-0.0370851441176888,
-0.0145209872269158));
#41256=CARTESIAN_POINT('Ctrl Pts',(0.000764779457276776,-0.0370771741690067,
-0.0145587951108632));
#41257=CARTESIAN_POINT('Ctrl Pts',(0.000579813914917926,-0.0370642273627232,
-0.0146088839571667));
#41258=CARTESIAN_POINT('Ctrl Pts',(0.000505282094828397,-0.0370591545566314,
-0.0146254480109019));
#41259=CARTESIAN_POINT('Ctrl Pts',(0.000391182189236705,-0.0370516090473155,
-0.0146453750044895));
#41260=CARTESIAN_POINT('Ctrl Pts',(0.00035210422655215,-0.0370490630008536,
-0.0146512489959077));
#41261=CARTESIAN_POINT('Ctrl Pts',(0.000278343736747567,-0.0370443250435151,
-0.0146605540765496));
#41262=CARTESIAN_POINT('Ctrl Pts',(0.000243697272084421,-0.0370421274216141,
-0.0146641911015208));
#41263=CARTESIAN_POINT('Ctrl Pts',(0.000163686157660349,-0.0370371107344305,
-0.0146709030335588));
#41264=CARTESIAN_POINT('Ctrl Pts',(0.000118290461412279,-0.0370343075948691,
-0.0146734669779745));
#41265=CARTESIAN_POINT('Ctrl Pts',(-0.000116565283842468,-0.0370199869260898,
-0.0146803133806776));
#41266=CARTESIAN_POINT('Ctrl Pts',(-0.000305990309238362,-0.0370091029457028,
-0.0146642831645918));
#41267=CARTESIAN_POINT('Ctrl Pts',(-0.000564558233591509,-0.0369937077781957,
-0.0146124044464048));
#41268=CARTESIAN_POINT('Ctrl Pts',(-0.000636631090722892,-0.0369893480618895,
-0.0145945734484314));
#41269=CARTESIAN_POINT('Ctrl Pts',(-0.000754204479724711,-0.0369819752793467,
-0.0145598660050422));
#41270=CARTESIAN_POINT('Ctrl Pts',(-0.000800198539011744,-0.0369790228788128,
-0.0145448240966522));
#41271=CARTESIAN_POINT('Ctrl Pts',(-0.000867554337385341,-0.0369745584985715,
-0.0145206107627216));
#41272=CARTESIAN_POINT('Ctrl Pts',(-0.000889273459909068,-0.0369730968291128,
-0.0145124599651095));
#41273=CARTESIAN_POINT('Ctrl Pts',(-0.000929534223632692,-0.0369703404143629,
-0.014496708212092));
#41274=CARTESIAN_POINT('Ctrl Pts',(-0.00094810336952257,-0.0369690497778317,
-0.0144891845102255));
#41275=CARTESIAN_POINT('Ctrl Pts',(-0.00099577709507874,-0.0369656888467966,
-0.0144691980782198));
#41276=CARTESIAN_POINT('Ctrl Pts',(-0.00102473835286799,-0.0369636013152733,
-0.0144564044150624));
#41277=CARTESIAN_POINT('Ctrl Pts',(-0.00118234216581179,-0.0369520171889592,
-0.0143831746833694));
#41278=CARTESIAN_POINT('Ctrl Pts',(-0.00130588642945272,-0.0369421227216923,
-0.0143124057243385));
#41279=CARTESIAN_POINT('Ctrl Pts',(-0.00150590312048323,-0.0369252946900534,
-0.0141739735551446));
#41280=CARTESIAN_POINT('Ctrl Pts',(-0.0015855018253225,-0.0369183412091915,
-0.0141114192519402));
#41281=CARTESIAN_POINT('Ctrl Pts',(-0.00171406350900674,-0.0369067593774612,
-0.0139971191472443));
#41282=CARTESIAN_POINT('Ctrl Pts',(-0.0017650074598079,-0.0369020618501485,
-0.0139477938189828));
#41283=CARTESIAN_POINT('Ctrl Pts',(-0.00184040823604885,-0.0368949365726642,
-0.013868305191199));
#41284=CARTESIAN_POINT('Ctrl Pts',(-0.0018663724053138,-0.0368924479739349,
-0.0138396291836528));
#41285=CARTESIAN_POINT('Ctrl Pts',(-0.00191456237588379,-0.03688775679489,
-0.0137838575673963));
#41286=CARTESIAN_POINT('Ctrl Pts',(-0.00193690415489454,-0.0368855499164958,
-0.0137568749011753));
#41287=CARTESIAN_POINT('Ctrl Pts',(-0.00198850037393263,-0.0368803695701905,
-0.0136918249708031));
#41288=CARTESIAN_POINT('Ctrl Pts',(-0.00201724043616705,-0.036877416045971,
-0.013653366520541));
#41289=CARTESIAN_POINT('Ctrl Pts',(-0.00215749318834099,-0.0368625952633362,
-0.0134539596241547));
#41290=CARTESIAN_POINT('Ctrl Pts',(-0.00225092607795201,-0.0368513970927537,
-0.013281144317455));
#41291=CARTESIAN_POINT('Ctrl Pts',(-0.00234810262601651,-0.0368359988845671,
-0.0130366351344967));
#41292=CARTESIAN_POINT('Ctrl Pts',(-0.00237042646227637,-0.0368320281218455,
-0.0129731040245538));
#41293=CARTESIAN_POINT('Ctrl Pts',(-0.00240349211014895,-0.0368252258398617,
-0.0128652692260529));
#41294=CARTESIAN_POINT('Ctrl Pts',(-0.00241563576422337,-0.0368224435814232,
-0.0128214320749274));
#41295=CARTESIAN_POINT('Ctrl Pts',(-0.00243204017488845,-0.0368181847744732,
-0.0127552464268947));
#41296=CARTESIAN_POINT('Ctrl Pts',(-0.00243720316374131,-0.036816751998145,
-0.012733129226598));
#41297=CARTESIAN_POINT('Ctrl Pts',(-0.00244639496721373,-0.036814011094812,
-0.0126911795184535));
#41298=CARTESIAN_POINT('Ctrl Pts',(-0.0024504855641188,-0.0368127061679313,
-0.0126713629756497));
#41299=CARTESIAN_POINT('Ctrl Pts',(-0.00246060112265457,-0.0368092456332954,
-0.0126191667481233));
#41300=CARTESIAN_POINT('Ctrl Pts',(-0.00246622739419459,-0.0368070707704291,
-0.01258671446946));
#41301=CARTESIAN_POINT('Ctrl Pts',(-0.00248985220071243,-0.036796646803082,
-0.012432391259228));
#41302=CARTESIAN_POINT('Ctrl Pts',(-0.00249946638041196,-0.0367881088263436,
-0.0123094172689833));
#41303=CARTESIAN_POINT('Ctrl Pts',(-0.00250063509976623,-0.0367686412633752,
-0.0120282695279969));
#41304=CARTESIAN_POINT('Ctrl Pts',(-0.00248631645326805,-0.0367577763474871,
-0.0118705663002083));
#41305=CARTESIAN_POINT('Ctrl Pts',(-0.00244810252673388,-0.0367440701375694,
-0.0116667030251335));
#41306=CARTESIAN_POINT('Ctrl Pts',(-0.00243756442219698,-0.0367408472555988,
-0.0116184304627458));
#41307=CARTESIAN_POINT('Ctrl Pts',(-0.00241707678493895,-0.0367354016567608,
-0.0115363382703059));
#41308=CARTESIAN_POINT('Ctrl Pts',(-0.00240783031484883,-0.0367331581484131,
-0.0115023601425407));
#41309=CARTESIAN_POINT('Ctrl Pts',(-0.00238708232382073,-0.0367285311772032,
-0.0114320175024609));
#41310=CARTESIAN_POINT('Ctrl Pts',(-0.00237546026863942,-0.0367261521508053,
-0.0113956978868597));
#41311=CARTESIAN_POINT('Ctrl Pts',(-0.00234099282563577,-0.0367196326852915,
-0.0112959094654426));
#41312=CARTESIAN_POINT('Ctrl Pts',(-0.00231640249687684,-0.0367155476019408,
-0.011233075947207));
#41313=CARTESIAN_POINT('Ctrl Pts',(-0.00225189965040911,-0.0367059619142053,
-0.0110860775100659));
#41314=CARTESIAN_POINT('Ctrl Pts',(-0.0022097676897272,-0.0367005224583516,
-0.0110029972017964));
#41315=CARTESIAN_POINT('Ctrl Pts',(-0.00208302931870926,-0.0366858048066992,
-0.0107842733090032));
#41316=CARTESIAN_POINT('Ctrl Pts',(-0.00198991179638418,-0.0366766112439648,
-0.0106540960393782));
#41317=CARTESIAN_POINT('Ctrl Pts',(-0.00186546062510466,-0.0366649546425962,
-0.0105112378927437));
#41318=CARTESIAN_POINT('Ctrl Pts',(-0.00184549028730537,-0.0366630999754086,
-0.0104891247450294));
#41319=CARTESIAN_POINT('Ctrl Pts',(-0.00181147493556331,-0.0366599564426063,
-0.0104527868789954));
#41320=CARTESIAN_POINT('Ctrl Pts',(-0.00179764622375264,-0.0366586823407605,
-0.0104383644913556));
#41321=CARTESIAN_POINT('Ctrl Pts',(-0.00176668900135214,-0.0366558360342001,
-0.0104068435160508));
#41322=CARTESIAN_POINT('Ctrl Pts',(-0.00174948372368646,-0.0366542587256429,
-0.0103898263577796));
#41323=CARTESIAN_POINT('Ctrl Pts',(-0.00169246110904554,-0.0366490539337528,
-0.0103350417665158));
#41324=CARTESIAN_POINT('Ctrl Pts',(-0.00165164888087414,-0.0366453643926251,
-0.0102983371757591));
#41325=CARTESIAN_POINT('Ctrl Pts',(-0.00153957170239187,-0.0366353949112652,
-0.0102040238792165));
#41326=CARTESIAN_POINT('Ctrl Pts',(-0.0014662913717555,-0.0366290437720225,
-0.0101489392003892));
#41327=CARTESIAN_POINT('Ctrl Pts',(-0.00126233992970625,-0.0366120542218922,
-0.0100124884119692));
#41328=CARTESIAN_POINT('Ctrl Pts',(-0.00112688958707917,-0.0366014876390732,
-0.00993893992301181));
#41329=CARTESIAN_POINT('Ctrl Pts',(-0.000939911680799899,-0.036588039556691,
-0.0098587367156452));
#41330=CARTESIAN_POINT('Ctrl Pts',(-0.000893725531981653,-0.0365848006553184,
-0.00984053352286213));
#41331=CARTESIAN_POINT('Ctrl Pts',(-0.000813868931503444,-0.0365793369893011,
-0.00981177645386332));
#41332=CARTESIAN_POINT('Ctrl Pts',(-0.00078046252223885,-0.0365770910671529,
-0.00980053849471339));
#41333=CARTESIAN_POINT('Ctrl Pts',(-0.000710521477533227,-0.0365724666210445,
-0.00977864520734291));
#41334=CARTESIAN_POINT('Ctrl Pts',(-0.000673958596474642,-0.0365700923773996,
-0.00976811007037555));
#41335=CARTESIAN_POINT('Ctrl Pts',(-0.000572447072846225,-0.0365636084103815,
-0.00974135454314261));
#41336=CARTESIAN_POINT('Ctrl Pts',(-0.000507063920339304,-0.0365595529565469,
-0.0097269010527598));
#41337=CARTESIAN_POINT('Ctrl Pts',(-0.000350693671306399,-0.0365500631393257,
-0.00969886640561742));
#41338=CARTESIAN_POINT('Ctrl Pts',(-0.000259382816589645,-0.0365446880321659,
-0.00968764671185863));
#41339=CARTESIAN_POINT('Ctrl Pts',(-5.67775373194534E-6,-0.0365298811520002,
-0.00967059402151928));
#41340=CARTESIAN_POINT('Ctrl Pts',(0.000156958885541035,-0.0365205441272375,
-0.00967551177728026));
#41341=CARTESIAN_POINT('Ctrl Pts',(0.000347211629370229,-0.0365087373076922,
-0.00969990609530903));
#41342=CARTESIAN_POINT('Ctrl Pts',(0.000376404586822594,-0.0365069000521739,
-0.00970417575474959));
#41343=CARTESIAN_POINT('Ctrl Pts',(0.000425198309956907,-0.036503776112433,
-0.00971219658293011));
#41344=CARTESIAN_POINT('Ctrl Pts',(0.000444841605217921,-0.0365025037208431,
-0.00971566754709915));
#41345=CARTESIAN_POINT('Ctrl Pts',(0.000488384087035448,-0.0364996480020015,
-0.00972390004960938));
#41346=CARTESIAN_POINT('Ctrl Pts',(0.000512257208666858,-0.0364980592869458,
-0.00972877622667336));
#41347=CARTESIAN_POINT('Ctrl Pts',(0.000590792072181815,-0.0364927650463557,
-0.00974601679721187));
#41348=CARTESIAN_POINT('Ctrl Pts',(0.000645106573247217,-0.0364889946491507,
-0.00975986959177396));
#41349=CARTESIAN_POINT('Ctrl Pts',(0.000790180433086395,-0.0364787036275535,
-0.00980211102496447));
#41350=CARTESIAN_POINT('Ctrl Pts',(0.000879862224628475,-0.0364721071590439,
-0.00983387147933904));
#41351=CARTESIAN_POINT('Ctrl Pts',(0.0011042663627245,-0.0364552614039727,
-0.00992805631955577));
#41352=CARTESIAN_POINT('Ctrl Pts',(0.00123565606089343,-0.0364450846335122,
-0.0099975144137393));
#41353=CARTESIAN_POINT('Ctrl Pts',(0.00140191148913842,-0.0364319847883632,
-0.0101053160605805));
#41354=CARTESIAN_POINT('Ctrl Pts',(0.0014428811107623,-0.0364287341578732,
-0.0101336547438982));
#41355=CARTESIAN_POINT('Ctrl Pts',(0.00151136937717297,-0.0364232572464437,
-0.0101841188166146));
#41356=CARTESIAN_POINT('Ctrl Pts',(0.00153931483466529,-0.0364210095393525,
-0.0102056366401827));
#41357=CARTESIAN_POINT('Ctrl Pts',(0.00159639611881538,-0.0364163868303005,
-0.0102515450326858));
#41358=CARTESIAN_POINT('Ctrl Pts',(0.00162545013808221,-0.0364140159962058,
-0.0102760230542913));
#41359=CARTESIAN_POINT('Ctrl Pts',(0.00170385358245753,-0.0364075572963168,
-0.0103451938031733));
#41360=CARTESIAN_POINT('Ctrl Pts',(0.0017519946202944,-0.0364035229324523,
-0.0103912112804881));
#41361=CARTESIAN_POINT('Ctrl Pts',(0.00186153963496296,-0.0363941009246183,
-0.0105046347322418));
#41362=CARTESIAN_POINT('Ctrl Pts',(0.00192120729947134,-0.0363887712190662,
-0.0105735845468272));
#41363=CARTESIAN_POINT('Ctrl Pts',(0.00207750402219195,-0.0363738997735992,
-0.0107755142547893));
#41364=CARTESIAN_POINT('Ctrl Pts',(0.00216497405934135,-0.0363644604052467,
-0.0109149620133418));
#41365=CARTESIAN_POINT('Ctrl Pts',(0.00225118270482701,-0.0363525462068422,
-0.0110881794429497));
#41366=CARTESIAN_POINT('Ctrl Pts',(0.00226377103503794,-0.0363507215581471,
-0.0111146282917565));
#41367=CARTESIAN_POINT('Ctrl Pts',(0.00228413701928706,-0.0363476117173661,
-0.0111594305784336));
#41368=CARTESIAN_POINT('Ctrl Pts',(0.00229216492712964,-0.036346340477327,
-0.0111776664503463));
#41369=CARTESIAN_POINT('Ctrl Pts',(0.00230957368568218,-0.0363434775285437,
-0.0112185292969175));
#41370=CARTESIAN_POINT('Ctrl Pts',(0.00231884086723502,-0.0363418802192158,
-0.0112412000065099));
#41371=CARTESIAN_POINT('Ctrl Pts',(0.00234853982716357,-0.0363365173614458,
-0.011317015493793));
#41372=CARTESIAN_POINT('Ctrl Pts',(0.00236748801046929,-0.0363326847400693,
-0.0113707189971832));
#41373=CARTESIAN_POINT('Ctrl Pts',(0.00241395958707821,-0.0363221406850836,
-0.0115183085507397));
#41374=CARTESIAN_POINT('Ctrl Pts',(0.00243783319235319,-0.0363153497085916,
-0.0116132395647649));
#41375=CARTESIAN_POINT('Ctrl Pts',(0.00248300807545953,-0.0362985975935805,
-0.011851065506205));
#41376=CARTESIAN_POINT('Ctrl Pts',(0.00249761459014234,-0.0362887078554256,
-0.0119948904697711));
#41377=CARTESIAN_POINT('Ctrl Pts',(0.00249991037372639,-0.036278358753258,
-0.0121514091157483));
#41378=CARTESIAN_POINT('Ctrl Pts',(0.0024999999999885,-0.0362775531707368,
-0.0121636312894922));
#41379=CARTESIAN_POINT('Ctrl Pts',(0.0025,-0.0362767501454997,-0.0121758532842053));
#41380=CARTESIAN_POINT('Ctrl Pts',(0.0025,-0.0361517921417372,-0.0121758532883121));
#41381=CARTESIAN_POINT('Ctrl Pts',(0.00250000000001732,-0.0361532969286916,
-0.0121511649771985));
#41382=CARTESIAN_POINT('Ctrl Pts',(0.0024996342921978,-0.0361548152361512,
-0.0121264770364312));
#41383=CARTESIAN_POINT('Ctrl Pts',(0.00249817675417057,-0.036157873977649,
-0.0120772944971944));
#41384=CARTESIAN_POINT('Ctrl Pts',(0.00249709026948674,-0.0361594138859829,
-0.0120528044824867));
#41385=CARTESIAN_POINT('Ctrl Pts',(0.00249447021013777,-0.0361622378119806,
-0.0120084794140612));
#41386=CARTESIAN_POINT('Ctrl Pts',(0.00249305971196675,-0.0361635156435239,
-0.0119886399896802));
#41387=CARTESIAN_POINT('Ctrl Pts',(0.00248899862140974,-0.036166696268289,
-0.0119397693412445));
#41388=CARTESIAN_POINT('Ctrl Pts',(0.00248607674588793,-0.0361686121509704,
-0.0119107646084144));
#41389=CARTESIAN_POINT('Ctrl Pts',(0.0024632065078464,-0.0361815275415674,
-0.0117176620029709));
#41390=CARTESIAN_POINT('Ctrl Pts',(0.0024275324011118,-0.0361930938416531,
-0.0115558482267804));
#41391=CARTESIAN_POINT('Ctrl Pts',(0.00234797607685132,-0.036210759873643,
-0.0113125885522278));
#41392=CARTESIAN_POINT('Ctrl Pts',(0.0023151306115756,-0.0362169635994065,
-0.0112280188199955));
#41393=CARTESIAN_POINT('Ctrl Pts',(0.00225041533685465,-0.0362275006411803,
-0.0110849671775967));
#41394=CARTESIAN_POINT('Ctrl Pts',(0.00222067230207197,-0.0362318860880483,
-0.0110256283119983));
#41395=CARTESIAN_POINT('Ctrl Pts',(0.00217027473221903,-0.0362386564823279,
-0.0109343439909819));
#41396=CARTESIAN_POINT('Ctrl Pts',(0.00215119460944113,-0.0362410926642295,
-0.0109015692728963));
#41397=CARTESIAN_POINT('Ctrl Pts',(0.00211296375747703,-0.0362457424840735,
-0.0108392063025702));
#41398=CARTESIAN_POINT('Ctrl Pts',(0.00209391866524951,-0.0362479591203712,
-0.0108095642179501));
#41399=CARTESIAN_POINT('Ctrl Pts',(0.00204646243198919,-0.0362532562979283,
-0.0107390269112703));
#41400=CARTESIAN_POINT('Ctrl Pts',(0.00201744330125472,-0.0362563140474926,
-0.0106985579403063));
#41401=CARTESIAN_POINT('Ctrl Pts',(0.00190053039245494,-0.0362680032982854,
-0.0105453920086602));
#41402=CARTESIAN_POINT('Ctrl Pts',(0.00180424597537692,-0.0362763247494811,
-0.010439442936532));
#41403=CARTESIAN_POINT('Ctrl Pts',(0.00162696619575666,-0.0362903875899586,
-0.0102751316646094));
#41404=CARTESIAN_POINT('Ctrl Pts',(0.00155058886803671,-0.0362961256843174,
-0.0102123273989611));
#41405=CARTESIAN_POINT('Ctrl Pts',(0.00142441094666287,-0.0363054412430823,
-0.010120535755744));
#41406=CARTESIAN_POINT('Ctrl Pts',(0.00137698190117222,-0.0363089103531119,
-0.0100884633952098));
#41407=CARTESIAN_POINT('Ctrl Pts',(0.00130772902535701,-0.036313992309463,
-0.0100450210835914));
#41408=CARTESIAN_POINT('Ctrl Pts',(0.00128677059063228,-0.0363155324036604,
-0.0100322995969759));
#41409=CARTESIAN_POINT('Ctrl Pts',(0.00124847617560075,-0.0363183564947223,
-0.0100098193835235));
#41410=CARTESIAN_POINT('Ctrl Pts',(0.00123120507554796,-0.0363196343005626,
-0.00999995586350741));
#41411=CARTESIAN_POINT('Ctrl Pts',(0.00118833787072059,-0.0363228146290413,
-0.00997614816207177));
#41412=CARTESIAN_POINT('Ctrl Pts',(0.00116261294324202,-0.0363247302345519,
-0.00996244403812264));
#41413=CARTESIAN_POINT('Ctrl Pts',(0.000989394468147815,-0.0363376475562736,
-0.00987402021924515));
#41414=CARTESIAN_POINT('Ctrl Pts',(0.000835048476674809,-0.0363492163461727,
-0.00981364558938359));
#41415=CARTESIAN_POINT('Ctrl Pts',(0.00058862236812525,-0.0363668836383153,
-0.00974444656543307));
#41416=CARTESIAN_POINT('Ctrl Pts',(0.00050008768365968,-0.0363730862942786,
-0.00972470467635234));
#41417=CARTESIAN_POINT('Ctrl Pts',(0.00034523322347434,-0.0363836218073554,
-0.00969891671423938));
#41418=CARTESIAN_POINT('Ctrl Pts',(0.000279384082836112,-0.036388006773449,
-0.00969062762879891));
#41419=CARTESIAN_POINT('Ctrl Pts',(0.000175500231029585,-0.0363947765997946,
-0.00968173273989668));
#41420=CARTESIAN_POINT('Ctrl Pts',(0.000137652102716281,-0.0363972126811644,
-0.00967935778649933));
#41421=CARTESIAN_POINT('Ctrl Pts',(6.45631858851483E-5,-0.0364018623922129,
-0.00967643883724852));
#41422=CARTESIAN_POINT('Ctrl Pts',(2.93364191766409E-5,-0.0364040790184051,
-0.00967577717484428));
#41423=CARTESIAN_POINT('Ctrl Pts',(-5.56805786665413E-5,-0.0364093763025371,
-0.00967597761172541));
#41424=CARTESIAN_POINT('Ctrl Pts',(-0.000105454781875508,-0.0364124341648461,
-0.00967758218416136));
#41425=CARTESIAN_POINT('Ctrl Pts',(-0.000297933856858051,-0.0364241332866678,
-0.00968955054345357));
#41426=CARTESIAN_POINT('Ctrl Pts',(-0.000439695786970914,-0.0364324636511113,
-0.00971066805494442));
#41427=CARTESIAN_POINT('Ctrl Pts',(-0.000674889545747243,-0.0364465292891003,
-0.00976664935470826));
#41428=CARTESIAN_POINT('Ctrl Pts',(-0.000769454155484879,-0.0364522610894565,
-0.00979516476164522));
#41429=CARTESIAN_POINT('Ctrl Pts',(-0.000915778419033223,-0.0364615680289228,
-0.00984891914892726));
#41430=CARTESIAN_POINT('Ctrl Pts',(-0.000968779356184011,-0.0364650350507535,
-0.00987048169580886));
#41431=CARTESIAN_POINT('Ctrl Pts',(-0.00104336442719228,-0.0364701145110101,
-0.00990385163642731));
#41432=CARTESIAN_POINT('Ctrl Pts',(-0.00106558944021804,-0.0364716542938449,
-0.00991419021192531));
#41433=CARTESIAN_POINT('Ctrl Pts',(-0.00110556773651197,-0.036474478114334,
-0.00993350727543451));
#41434=CARTESIAN_POINT('Ctrl Pts',(-0.0011233719444242,-0.0364757559694346,
-0.00994237370716314));
#41435=CARTESIAN_POINT('Ctrl Pts',(-0.00116700820236698,-0.0364789368402748,
-0.00996475812456358));
#41436=CARTESIAN_POINT('Ctrl Pts',(-0.00119271230461342,-0.0364808529507348,
-0.00997851691147382));
#41437=CARTESIAN_POINT('Ctrl Pts',(-0.00136249481386875,-0.0364937666334979,
-0.0100732540690368));
#41438=CARTESIAN_POINT('Ctrl Pts',(-0.00149847041161189,-0.036505330758113,
-0.0101678950466629));
#41439=CARTESIAN_POINT('Ctrl Pts',(-0.00169303184232238,-0.0365229956639271,
-0.0103341521300499));
#41440=CARTESIAN_POINT('Ctrl Pts',(-0.00175870768402333,-0.0365292003026396,
-0.0103967609568813));
#41441=CARTESIAN_POINT('Ctrl Pts',(-0.00186630593728238,-0.0365397386233811,
-0.0105111297115197));
#41442=CARTESIAN_POINT('Ctrl Pts',(-0.00190983191449707,-0.036544124456584,
-0.0105612493828944));
#41443=CARTESIAN_POINT('Ctrl Pts',(-0.00197501891260304,-0.0365508952693436,
-0.0106426415966734));
#41444=CARTESIAN_POINT('Ctrl Pts',(-0.00199804702552586,-0.0365533314959028,
-0.0106727744044653));
#41445=CARTESIAN_POINT('Ctrl Pts',(-0.00204112950067508,-0.0365579813068854,
-0.0107318895407052));
#41446=CARTESIAN_POINT('Ctrl Pts',(-0.00206127394947851,-0.036560197891696,
-0.010760794687589));
#41447=CARTESIAN_POINT('Ctrl Pts',(-0.00210839480464267,-0.0365654947794551,
-0.0108315506887275));
#41448=CARTESIAN_POINT('Ctrl Pts',(-0.0021347455600349,-0.0365685522962797,
-0.0108738010540575));
#41449=CARTESIAN_POINT('Ctrl Pts',(-0.0022316391465855,-0.0365802238850457,
-0.0110400169025678));
#41450=CARTESIAN_POINT('Ctrl Pts',(-0.00229278851383359,-0.0365885293957336,
-0.0111691442498614));
#41451=CARTESIAN_POINT('Ctrl Pts',(-0.00237717351599074,-0.0366025875573592,
-0.0113955656445488));
#41452=CARTESIAN_POINT('Ctrl Pts',(-0.00240620629511256,-0.036608337229675,
-0.011490308210455));
#41453=CARTESIAN_POINT('Ctrl Pts',(-0.0024430533413161,-0.0366176686467207,
-0.0116422104894747));
#41454=CARTESIAN_POINT('Ctrl Pts',(-0.00245464291861119,-0.0366211415914102,
-0.0116983478731764));
#41455=CARTESIAN_POINT('Ctrl Pts',(-0.00246842316546757,-0.036626228096677,
-0.0117790049578425));
#41456=CARTESIAN_POINT('Ctrl Pts',(-0.00247219739638716,-0.0366277687225857,
-0.0118032389482794));
#41457=CARTESIAN_POINT('Ctrl Pts',(-0.00247838547372813,-0.0366305932312941,
-0.0118472182194491));
#41458=CARTESIAN_POINT('Ctrl Pts',(-0.00248092123203021,-0.0366318709074048,
-0.0118669434164088));
#41459=CARTESIAN_POINT('Ctrl Pts',(-0.00248659076542711,-0.0366350500853271,
-0.0119156322172972));
#41460=CARTESIAN_POINT('Ctrl Pts',(-0.00248945399433441,-0.0366369646464156,
-0.0119446233639717));
#41461=CARTESIAN_POINT('Ctrl Pts',(-0.00250519307016456,-0.0366498895321647,
-0.0121385867037762));
#41462=CARTESIAN_POINT('Ctrl Pts',(-0.00250216785424727,-0.0366614680161941,
-0.0123044278731853));
#41463=CARTESIAN_POINT('Ctrl Pts',(-0.00247217179840446,-0.0366791403559196,
-0.0125586995973125));
#41464=CARTESIAN_POINT('Ctrl Pts',(-0.00245667809783091,-0.0366853389791898,
-0.0126480181772522));
#41465=CARTESIAN_POINT('Ctrl Pts',(-0.00242150302932559,-0.0366958687944396,
-0.0128009296560709));
#41466=CARTESIAN_POINT('Ctrl Pts',(-0.00240407065510009,-0.0367002520094542,
-0.0128649417761621));
#41467=CARTESIAN_POINT('Ctrl Pts',(-0.00237270290059417,-0.0367070198541235,
-0.0129643444210921));
#41468=CARTESIAN_POINT('Ctrl Pts',(-0.00236047245004971,-0.0367094556523334,
-0.0130002363207279));
#41469=CARTESIAN_POINT('Ctrl Pts',(-0.00233531102820602,-0.0367141051878846,
-0.0130689174097979));
#41470=CARTESIAN_POINT('Ctrl Pts',(-0.00232249393527816,-0.0367163219137734,
-0.0131017383997141));
#41471=CARTESIAN_POINT('Ctrl Pts',(-0.0022898952971021,-0.0367216200561394,
-0.0131802732696674));
#41472=CARTESIAN_POINT('Ctrl Pts',(-0.00226943282765788,-0.0367246786571308,
-0.0132256890407943));
#41473=CARTESIAN_POINT('Ctrl Pts',(-0.00218425900271001,-0.0367364794608299,
-0.0134005810244449));
#41474=CARTESIAN_POINT('Ctrl Pts',(-0.00210971157630988,-0.0367449020013716,
-0.0135249519644654));
#41475=CARTESIAN_POINT('Ctrl Pts',(-0.00196762097177015,-0.0367589962287997,
-0.0137211612422479));
#41476=CARTESIAN_POINT('Ctrl Pts',(-0.00190585685069581,-0.03676466239984,
-0.0137967224149057));
#41477=CARTESIAN_POINT('Ctrl Pts',(-0.00180136522244201,-0.0367738792902254,
-0.0139103021666383));
#41478=CARTESIAN_POINT('Ctrl Pts',(-0.00176147677090706,-0.0367773243908369,
-0.0139507978499153));
#41479=CARTESIAN_POINT('Ctrl Pts',(-0.00170249836123113,-0.03678237778154,
-0.014006726737373));
#41480=CARTESIAN_POINT('Ctrl Pts',(-0.00168450494104781,-0.0367839144467999,
-0.0140232951013958));
#41481=CARTESIAN_POINT('Ctrl Pts',(-0.00165143667225138,-0.0367867357696183,
-0.0140528596616974));
#41482=CARTESIAN_POINT('Ctrl Pts',(-0.00163644482265526,-0.0367880143348335,
-0.0140659443583956));
#41483=CARTESIAN_POINT('Ctrl Pts',(-0.00160265868890948,-0.0367908934064162,
-0.0140947292020543));
#41484=CARTESIAN_POINT('Ctrl Pts',(-0.00158378709633748,-0.0367924995960476,
-0.0141103346075932));
#41485=CARTESIAN_POINT('Ctrl Pts',(-0.00150439359046006,-0.0367992384943448,
-0.0141740466991031));
#41486=CARTESIAN_POINT('Ctrl Pts',(-0.00144188970856939,-0.0368044990645285,
-0.0142196069584674));
#41487=CARTESIAN_POINT('Ctrl Pts',(-0.00125115314914072,-0.0368202172315811,
-0.0143455293211941));
#41488=CARTESIAN_POINT('Ctrl Pts',(-0.00111761228202061,-0.0368307807472205,
-0.0144172425660154));
#41489=CARTESIAN_POINT('Ctrl Pts',(-0.00089827136869339,-0.0368469809664464,
-0.0145105249262246));
#41490=CARTESIAN_POINT('Ctrl Pts',(-0.000816403892349176,-0.0368528012427316,
-0.0145403977517451));
#41491=CARTESIAN_POINT('Ctrl Pts',(-0.000693967532365007,-0.036861166894107,
-0.0145779539541803));
#41492=CARTESIAN_POINT('Ctrl Pts',(-0.00065450752144139,-0.0368638134889614,
-0.0145890044989252));
#41493=CARTESIAN_POINT('Ctrl Pts',(-0.000581250311792042,-0.0368686399286667,
-0.0146075904271785));
#41494=CARTESIAN_POINT('Ctrl Pts',(-0.000547534542512971,-0.0368708278713999,
-0.0146154031545027));
#41495=CARTESIAN_POINT('Ctrl Pts',(-0.000470743990796697,-0.0368757410587395,
-0.014631525008002));
#41496=CARTESIAN_POINT('Ctrl Pts',(-0.000427590417983763,-0.0368784526320793,
-0.0146394056596525));
#41497=CARTESIAN_POINT('Ctrl Pts',(-0.000269596982441658,-0.036888226000936,
-0.0146639812537609));
#41498=CARTESIAN_POINT('Ctrl Pts',(-0.000153835917919869,-0.0368950843502155,
-0.0146738127984216));
#41499=CARTESIAN_POINT('Ctrl Pts',(0.000126232869975961,-0.0369114508375757,
-0.0146780480195134));
#41500=CARTESIAN_POINT('Ctrl Pts',(0.000290097198179099,-0.0369208319654994,
-0.0146643764553365));
#41501=CARTESIAN_POINT('Ctrl Pts',(0.000492094376711041,-0.0369332714562593,
-0.014627292221559));
#41502=CARTESIAN_POINT('Ctrl Pts',(0.000532569559533968,-0.0369358105335989,
-0.0146188184863748));
#41503=CARTESIAN_POINT('Ctrl Pts',(0.000594191105201978,-0.036939772999877,
-0.0146043135513696));
#41504=CARTESIAN_POINT('Ctrl Pts',(0.00061550066413709,-0.0369411612306676,
-0.0145990002442089));
#41505=CARTESIAN_POINT('Ctrl Pts',(0.000656931831980199,-0.0369439003268179,
-0.0145880880822758));
#41506=CARTESIAN_POINT('Ctrl Pts',(0.000677058449612257,-0.0369452497874767,
-0.0145825165150732));
#41507=CARTESIAN_POINT('Ctrl Pts',(0.000731286758599727,-0.0369489326942958,
-0.0145667706992798));
#41508=CARTESIAN_POINT('Ctrl Pts',(0.00076524405256289,-0.0369512894517418,
-0.0145561195837569));
#41509=CARTESIAN_POINT('Ctrl Pts',(0.000843357924680048,-0.0369568112282263,
-0.0145297740096758));
#41510=CARTESIAN_POINT('Ctrl Pts',(0.000887323544886222,-0.0369599946877288,
-0.0145135555439412));
#41511=CARTESIAN_POINT('Ctrl Pts',(0.00105743149094895,-0.0369725494534005,
-0.0144453143032938));
#41512=CARTESIAN_POINT('Ctrl Pts',(0.00117968727277185,-0.0369820782492673,
-0.0143842359263524));
#41513=CARTESIAN_POINT('Ctrl Pts',(0.00138750242481359,-0.0369987432919234,
-0.014258208031137));
#41514=CARTESIAN_POINT('Ctrl Pts',(0.00147503332822346,-0.0370059338421185,
-0.0141971512952803));
#41515=CARTESIAN_POINT('Ctrl Pts',(0.00159269736944193,-0.037015807946753,
-0.0141033486013389));
#41516=CARTESIAN_POINT('Ctrl Pts',(0.00162626396876562,-0.0370186519954304,
-0.0140751134028164));
#41517=CARTESIAN_POINT('Ctrl Pts',(0.00168495799956095,-0.0370236786460554,
-0.0140230441184259));
#41518=CARTESIAN_POINT('Ctrl Pts',(0.00171036523524432,-0.0370258736920758,
-0.0139995441540643));
#41519=CARTESIAN_POINT('Ctrl Pts',(0.00176477311080598,-0.037030621518774,
-0.0139470830045284));
#41520=CARTESIAN_POINT('Ctrl Pts',(0.00179356633607497,-0.0370331650295079,
-0.0139179207185068));
#41521=CARTESIAN_POINT('Ctrl Pts',(0.00188129117384234,-0.0370410299940846,
-0.0138245896676529));
#41522=CARTESIAN_POINT('Ctrl Pts',(0.00193759644071001,-0.0370462472017684,
-0.0137580385614667));
#41523=CARTESIAN_POINT('Ctrl Pts',(0.002081919231378,-0.0370603246273959,
-0.0135681633444368));
#41524=CARTESIAN_POINT('Ctrl Pts',(0.00216238379915213,-0.0370689902042344,
-0.0134395817250453));
#41525=CARTESIAN_POINT('Ctrl Pts',(0.00226556750569695,-0.0370824683125001,
-0.0132356461609043));
#41526=CARTESIAN_POINT('Ctrl Pts',(0.00229720156907751,-0.0370870846129693,
-0.013165206580885));
#41527=CARTESIAN_POINT('Ctrl Pts',(0.00233450993633415,-0.0370933687283898,
-0.0130706508566329));
#41528=CARTESIAN_POINT('Ctrl Pts',(0.00234315989326879,-0.0370948974266925,
-0.0130477483184021));
#41529=CARTESIAN_POINT('Ctrl Pts',(0.00235822829673303,-0.0370977017584978,
-0.0130060070404093));
#41530=CARTESIAN_POINT('Ctrl Pts',(0.00236476048704052,-0.0370989712793348,
-0.0129872124931785));
#41531=CARTESIAN_POINT('Ctrl Pts',(0.00237882319653925,-0.0371018307596736,
-0.0129451378391678));
#41532=CARTESIAN_POINT('Ctrl Pts',(0.00238623703721665,-0.0371034263155972,
-0.0129218232702511));
#41533=CARTESIAN_POINT('Ctrl Pts',(0.00240974314132829,-0.0371087828488224,
-0.0128439640018595));
#41534=CARTESIAN_POINT('Ctrl Pts',(0.00242431555260982,-0.037112610749602,
-0.0127889822036274));
#41535=CARTESIAN_POINT('Ctrl Pts',(0.00245877930717899,-0.0371231378500889,
-0.0126383855162499));
#41536=CARTESIAN_POINT('Ctrl Pts',(0.0024749645776264,-0.0371299163886139,
-0.0125420239951231));
#41537=CARTESIAN_POINT('Ctrl Pts',(0.00249515434765317,-0.037142895916894,
-0.0123555552999207));
#41538=CARTESIAN_POINT('Ctrl Pts',(0.0025,-0.0371490887583808,-0.0122657206983139));
#41539=CARTESIAN_POINT('Ctrl Pts',(0.0025,-0.0371551761478877,-0.0121758532865581));
#41540=CARTESIAN_POINT('Origin',(0.,-0.0397787743898723,-0.0121758532865581));
#41541=CARTESIAN_POINT('',(0.0025,-0.0382770671668707,-0.0121758532865581));
#41542=CARTESIAN_POINT('',(0.0025,-0.0381539840246788,-0.0121758532868784));
#41543=CARTESIAN_POINT('',(0.0025,-0.0397787743898723,-0.0121758532865581));
#41544=CARTESIAN_POINT('Ctrl Pts',(0.0025,-0.0382770671668707,-0.0121758532865581));
#41545=CARTESIAN_POINT('Ctrl Pts',(0.0025,-0.038266648351978,-0.0123484233248802));
#41546=CARTESIAN_POINT('Ctrl Pts',(0.00248213258965094,-0.0382567310896037,
-0.0125205849801563));
#41547=CARTESIAN_POINT('Ctrl Pts',(0.00243165258255063,-0.0382423854219848,
-0.0127609933562431));
#41548=CARTESIAN_POINT('Ctrl Pts',(0.00241354186202213,-0.0382380963272977,
-0.0128317021372035));
#41549=CARTESIAN_POINT('Ctrl Pts',(0.00237847075891303,-0.0382308262909001,
-0.0129473250147727));
#41550=CARTESIAN_POINT('Ctrl Pts',(0.00236326300636025,-0.0382279038854537,
-0.0129927248310423));
#41551=CARTESIAN_POINT('Ctrl Pts',(0.00233879518817045,-0.038223475770528,
-0.0130593527232582));
#41552=CARTESIAN_POINT('Ctrl Pts',(0.00233052768115301,-0.0382220191983679,
-0.0130809360570954));
#41553=CARTESIAN_POINT('Ctrl Pts',(0.00231452670270875,-0.0382192660654279,
-0.0131210351070867));
#41554=CARTESIAN_POINT('Ctrl Pts',(0.00230686748142584,-0.0382179734620846,
-0.0131395777521876));
#41555=CARTESIAN_POINT('Ctrl Pts',(0.00228647242581149,-0.038214597660604,
-0.0131873168000068));
#41556=CARTESIAN_POINT('Ctrl Pts',(0.0022734004952124,-0.0382124969175176,
-0.0132163649697932));
#41557=CARTESIAN_POINT('Ctrl Pts',(0.00220025267773399,-0.0382010942503547,
-0.0133709499643583));
#41558=CARTESIAN_POINT('Ctrl Pts',(0.00213033134399354,-0.0381914124996758,
-0.0134915475237513));
#41559=CARTESIAN_POINT('Ctrl Pts',(0.00199201142202049,-0.0381746777935562,
-0.013689932750067));
#41560=CARTESIAN_POINT('Ctrl Pts',(0.00192813818566363,-0.0381676127607061,
-0.0137704793170425));
#41561=CARTESIAN_POINT('Ctrl Pts',(0.00181169201214085,-0.0381558784733875,
-0.0139000589343368));
#41562=CARTESIAN_POINT('Ctrl Pts',(0.00176163394186917,-0.0381511372952276,
-0.0139511731146526));
#41563=CARTESIAN_POINT('Ctrl Pts',(0.00168115620616752,-0.03814396308667,
-0.0140265875247387));
#41564=CARTESIAN_POINT('Ctrl Pts',(0.00165224924064926,-0.0381414677931332,
-0.0140524395821871));
#41565=CARTESIAN_POINT('Ctrl Pts',(0.00159613119701894,-0.0381367717600846,
-0.0141003245865437));
#41566=CARTESIAN_POINT('Ctrl Pts',(0.00156903617274202,-0.0381345665462568,
-0.0141224786392016));
#41567=CARTESIAN_POINT('Ctrl Pts',(0.00150388348262836,-0.0381294022216525,
-0.0141735057746038));
#41568=CARTESIAN_POINT('Ctrl Pts',(0.00146544531958654,-0.0381264626895305,
-0.0142018719071543));
#41569=CARTESIAN_POINT('Ctrl Pts',(0.00126422037268961,-0.0381115638696141,
-0.014341644368517));
#41570=CARTESIAN_POINT('Ctrl Pts',(0.00108948233514589,-0.03810028716686,
-0.0144345998725599));
#41571=CARTESIAN_POINT('Ctrl Pts',(0.000843375268429188,-0.0380848313346593,
-0.014530248968462));
#41572=CARTESIAN_POINT('Ctrl Pts',(0.000780180522547825,-0.0380808902953429,
-0.0145519379353241));
#41573=CARTESIAN_POINT('Ctrl Pts',(0.000672841287146767,-0.0380741320873495,
-0.0145840335931913));
#41574=CARTESIAN_POINT('Ctrl Pts',(0.00062914429002299,-0.038071363357087,
-0.0145958170698696));
#41575=CARTESIAN_POINT('Ctrl Pts',(0.00056311357261925,-0.038067121015749,
-0.0146117139289849));
#41576=CARTESIAN_POINT('Ctrl Pts',(0.000541002316568172,-0.0380656906816978,
-0.0146167200117643));
#41577=CARTESIAN_POINT('Ctrl Pts',(0.000499014490772209,-0.0380629509935083,
-0.0146256277130373));
#41578=CARTESIAN_POINT('Ctrl Pts',(0.000479153134571793,-0.0380616447631206,
-0.0146295896961051));
#41579=CARTESIAN_POINT('Ctrl Pts',(0.00042676264808953,-0.0380581754496267,
-0.0146393803772029));
#41580=CARTESIAN_POINT('Ctrl Pts',(0.000394162893044924,-0.0380559929334715,
-0.0146448059910956));
#41581=CARTESIAN_POINT('Ctrl Pts',(0.000237681942354664,-0.0380454325208168,
-0.0146676713405692));
#41582=CARTESIAN_POINT('Ctrl Pts',(0.0001127222718948,-0.0380367573077866,
-0.0146764410897942));
#41583=CARTESIAN_POINT('Ctrl Pts',(-0.00012229675935095,-0.0380204846613085,
-0.0146752792485404));
#41584=CARTESIAN_POINT('Ctrl Pts',(-0.000232086539329571,-0.038012900235242,
-0.0146674844334593));
#41585=CARTESIAN_POINT('Ctrl Pts',(-0.000414653142569712,-0.0380004645323029,
-0.0146423464343174));
#41586=CARTESIAN_POINT('Ctrl Pts',(-0.000487809575432174,-0.0379955279587467,
-0.0146289267159705));
#41587=CARTESIAN_POINT('Ctrl Pts',(-0.000598483184159789,-0.0379881343249413,
-0.0146034767591937));
#41588=CARTESIAN_POINT('Ctrl Pts',(-0.00063649064759546,-0.0379856085767315,
-0.0145937899647144));
#41589=CARTESIAN_POINT('Ctrl Pts',(-0.000707857580316338,-0.0379808875062097,
-0.0145738014226241));
#41590=CARTESIAN_POINT('Ctrl Pts',(-0.000741259410710683,-0.0379786869673909,
-0.0145636875132853));
#41591=CARTESIAN_POINT('Ctrl Pts',(-0.000818981756903161,-0.037973582053773,
-0.014538365392493));
#41592=CARTESIAN_POINT('Ctrl Pts',(-0.000863108846696353,-0.0379706958386521,
-0.0145226038289881));
#41593=CARTESIAN_POINT('Ctrl Pts',(-0.00107697192358637,-0.037956724362385,
-0.014439365787931));
#41594=CARTESIAN_POINT('Ctrl Pts',(-0.00123940278310876,-0.0379462140620093,
-0.0143546703154158));
#41595=CARTESIAN_POINT('Ctrl Pts',(-0.00145520677732491,-0.0379310638560855,
-0.0142101379644974));
#41596=CARTESIAN_POINT('Ctrl Pts',(-0.00151722691609498,-0.0379265429119622,
-0.0141643105092558));
#41597=CARTESIAN_POINT('Ctrl Pts',(-0.00161546144222776,-0.0379189366981224,
-0.0140844490439993));
#41598=CARTESIAN_POINT('Ctrl Pts',(-0.00165295557991421,-0.0379159170948097,
-0.0140520703874035));
#41599=CARTESIAN_POINT('Ctrl Pts',(-0.001706697726981,-0.0379113716998078,
-0.0140027987497902));
#41600=CARTESIAN_POINT('Ctrl Pts',(-0.00172371144335557,-0.0379098989077076,
-0.0139867551672282));
#41601=CARTESIAN_POINT('Ctrl Pts',(-0.00175483575075298,-0.0379071355314612,
-0.0139565695695701));
#41602=CARTESIAN_POINT('Ctrl Pts',(-0.00176900621429655,-0.0379058493936831,
-0.0139424930062018));
#41603=CARTESIAN_POINT('Ctrl Pts',(-0.00180489770710741,-0.0379025216360983,
-0.0139059745726439));
#41604=CARTESIAN_POINT('Ctrl Pts',(-0.00182636912948285,-0.0379004634545333,
-0.0138832931810054));
#41605=CARTESIAN_POINT('Ctrl Pts',(-0.00194621227548652,-0.037888613615882,
-0.0137518492914627));
#41606=CARTESIAN_POINT('Ctrl Pts',(-0.00203528250209412,-0.0378783943318016,
-0.0136350056196532));
#41607=CARTESIAN_POINT('Ctrl Pts',(-0.00216644150800256,-0.037861410949501,
-0.0134273814148368));
#41608=CARTESIAN_POINT('Ctrl Pts',(-0.00221427918536977,-0.037854613938942,
-0.013340654498436));
#41609=CARTESIAN_POINT('Ctrl Pts',(-0.00228695182231855,-0.0378432472822442,
-0.0131881511219335));
#41610=CARTESIAN_POINT('Ctrl Pts',(-0.00231438818850902,-0.0378386122107011,
-0.0131237479741729));
#41611=CARTESIAN_POINT('Ctrl Pts',(-0.00235268953567896,-0.0378315573417044,
-0.0130222200966319));
#41612=CARTESIAN_POINT('Ctrl Pts',(-0.00236545581178896,-0.0378290786802289,
-0.0129858556904086));
#41613=CARTESIAN_POINT('Ctrl Pts',(-0.00238822519367106,-0.037824395079808,
-0.0129158602134208));
#41614=CARTESIAN_POINT('Ctrl Pts',(-0.00239837098322131,-0.0378221860956407,
-0.0128822856242248));
#41615=CARTESIAN_POINT('Ctrl Pts',(-0.00242081373804952,-0.0378169832103377,
-0.0128019503705473));
#41616=CARTESIAN_POINT('Ctrl Pts',(-0.0024324675822765,-0.037814009784381,
-0.0127550239281337));
#41617=CARTESIAN_POINT('Ctrl Pts',(-0.00248397054685601,-0.0377993005476244,
-0.0125185110836304));
#41618=CARTESIAN_POINT('Ctrl Pts',(-0.00250304935813366,-0.0377882149399982,
-0.0123250908286065));
#41619=CARTESIAN_POINT('Ctrl Pts',(-0.00249839422320036,-0.0377728984480414,
-0.0120633319114935));
#41620=CARTESIAN_POINT('Ctrl Pts',(-0.0024944038416649,-0.0377688845626646,
-0.0119953450407695));
#41621=CARTESIAN_POINT('Ctrl Pts',(-0.00248309530968993,-0.0377620184978214,
-0.011882022402238));
#41622=CARTESIAN_POINT('Ctrl Pts',(-0.0024772941505594,-0.0377592167969208,
-0.0118365716291559));
#41623=CARTESIAN_POINT('Ctrl Pts',(-0.00246674595997307,-0.0377549344726481,
-0.0117688118173486));
#41624=CARTESIAN_POINT('Ctrl Pts',(-0.00246293679715169,-0.0377534983494909,
-0.0117463644825976));
#41625=CARTESIAN_POINT('Ctrl Pts',(-0.00245516903720368,-0.0377507558901246,
-0.0117040976486968));
#41626=CARTESIAN_POINT('Ctrl Pts',(-0.00245127573949789,-0.0377494528624718,
-0.0116842685808227));
#41627=CARTESIAN_POINT('Ctrl Pts',(-0.00244043933679202,-0.0377460051162837,
-0.0116324106847229));
#41628=CARTESIAN_POINT('Ctrl Pts',(-0.00243310615354872,-0.0377438414008662,
-0.0116004679998408));
#41629=CARTESIAN_POINT('Ctrl Pts',(-0.00239825207901131,-0.0377342614452151,
-0.0114612551109804));
#41630=CARTESIAN_POINT('Ctrl Pts',(-0.00236425029004917,-0.0377266129669288,
-0.0113557431978358));
#41631=CARTESIAN_POINT('Ctrl Pts',(-0.00227924626902856,-0.0377106726335527,
-0.0111417743626027));
#41632=CARTESIAN_POINT('Ctrl Pts',(-0.00222721189728784,-0.0377024004858524,
-0.0110340066596268));
#41633=CARTESIAN_POINT('Ctrl Pts',(-0.00212891630433674,-0.0376890583085457,
-0.0108629310756423));
#41634=CARTESIAN_POINT('Ctrl Pts',(-0.00208703917488962,-0.0376838835626023,
-0.0107973327615932));
#41635=CARTESIAN_POINT('Ctrl Pts',(-0.00201925249087216,-0.0376762247688677,
-0.0107013372466339));
#41636=CARTESIAN_POINT('Ctrl Pts',(-0.00199556615574467,-0.0376736638126523,
-0.0106694356219295));
#41637=CARTESIAN_POINT('Ctrl Pts',(-0.00194972728444761,-0.0376689130109799,
-0.0106106778723023));
#41638=CARTESIAN_POINT('Ctrl Pts',(-0.00192775500652634,-0.0376667170987196,
-0.0105836939397391));
#41639=CARTESIAN_POINT('Ctrl Pts',(-0.00187603710986693,-0.0376617246778843,
-0.0105228206022559));
#41640=CARTESIAN_POINT('Ctrl Pts',(-0.00184592333688678,-0.0376589435342649,
-0.0104892591725747));
#41641=CARTESIAN_POINT('Ctrl Pts',(-0.0016826449216898,-0.0376444655533574,
-0.0103169026617696));
#41642=CARTESIAN_POINT('Ctrl Pts',(-0.00153470487112565,-0.0376334272681061,
-0.0101930074092318));
#41643=CARTESIAN_POINT('Ctrl Pts',(-0.00131297605128778,-0.0376179279783162,
-0.0100471372151987));
#41644=CARTESIAN_POINT('Ctrl Pts',(-0.00125020949291117,-0.0376136330159059,
-0.0100096784792033));
#41645=CARTESIAN_POINT('Ctrl Pts',(-0.00114371618836145,-0.0376063544853546,
-0.00995229553907206));
#41646=CARTESIAN_POINT('Ctrl Pts',(-0.00110089385966737,-0.0376034296172707,
-0.00993078583470947));
#41647=CARTESIAN_POINT('Ctrl Pts',(-0.00103653257121679,-0.0375989984507089,
-0.00990074124558544));
#41648=CARTESIAN_POINT('Ctrl Pts',(-0.00101544832222549,-0.0375975413772552,
-0.00989125284397109));
#41649=CARTESIAN_POINT('Ctrl Pts',(-0.000975826893932983,-0.0375947876648727,
-0.00987407908875711));
#41650=CARTESIAN_POINT('Ctrl Pts',(-0.000957323491036033,-0.0375934949928333,
-0.00986632212002606));
#41651=CARTESIAN_POINT('Ctrl Pts',(-0.000909212325078636,-0.0375901194626916,
-0.00984683048040391));
#41652=CARTESIAN_POINT('Ctrl Pts',(-0.000879470681621455,-0.0375880190717043,
-0.00983543764281324));
#41653=CARTESIAN_POINT('Ctrl Pts',(-0.000718505933719115,-0.0375766078509464,
-0.00977727975102571));
#41654=CARTESIAN_POINT('Ctrl Pts',(-0.000583772210240915,-0.0375669164424697,
-0.00974097940270314));
#41655=CARTESIAN_POINT('Ctrl Pts',(-0.000345762855775532,-0.0375501781106134,
-0.00969775359825071));
#41656=CARTESIAN_POINT('Ctrl Pts',(-0.000243758648160511,-0.0375431187611106,
-0.00968564955050368));
#41657=CARTESIAN_POINT('Ctrl Pts',(-6.99317160158425E-5,-0.0375313921284449,
-0.0096758096358315));
#41658=CARTESIAN_POINT('Ctrl Pts',(1.57452670687609E-6,-0.0375266530757697,
-0.00967483193645387));
#41659=CARTESIAN_POINT('Ctrl Pts',(0.000111785748213136,-0.0375194810481381,
-0.00967805280963605));
#41660=CARTESIAN_POINT('Ctrl Pts',(0.000150511321571955,-0.0375169858909543,
-0.00968008689398806));
#41661=CARTESIAN_POINT('Ctrl Pts',(0.000224075758914965,-0.0375122896015905,
-0.0096856695418937));
#41662=CARTESIAN_POINT('Ctrl Pts',(0.000258917622393482,-0.0375100840063717,
-0.0096890507441003));
#41663=CARTESIAN_POINT('Ctrl Pts',(0.000341129780876372,-0.0375049179300782,
-0.00969877565138785));
#41664=CARTESIAN_POINT('Ctrl Pts',(0.000388412563168479,-0.0375019770558065,
-0.00970574817488102));
#41665=CARTESIAN_POINT('Ctrl Pts',(0.000629568223582207,-0.0374870849273301,
-0.00974840662841968));
#41666=CARTESIAN_POINT('Ctrl Pts',(0.000818921324996043,-0.037475814987661,
-0.0098055737602736));
#41667=CARTESIAN_POINT('Ctrl Pts',(0.00106085895570087,-0.0374603642066134,
-0.00991111379467665));
#41668=CARTESIAN_POINT('Ctrl Pts',(0.00112101794069365,-0.0374564206572916,
-0.00994028076458841));
#41669=CARTESIAN_POINT('Ctrl Pts',(0.00121984533105607,-0.0374496586916192,
-0.00999318818389156));
#41670=CARTESIAN_POINT('Ctrl Pts',(0.00125916764197979,-0.0374468887744168,
-0.0100156343406633));
#41671=CARTESIAN_POINT('Ctrl Pts',(0.00131723694949441,-0.0374426449026767,
-0.0100509059909875));
#41672=CARTESIAN_POINT('Ctrl Pts',(0.00133645575220129,-0.0374412142612031,
-0.0100629405755851));
#41673=CARTESIAN_POINT('Ctrl Pts',(0.0013725243257484,-0.0374384743380744,
-0.0100862152481735));
#41674=CARTESIAN_POINT('Ctrl Pts',(0.00138940593267399,-0.0374371681873588,
-0.0100974016509193));
#41675=CARTESIAN_POINT('Ctrl Pts',(0.00143346693514852,-0.0374336994114188,
-0.0101273747846713));
#41676=CARTESIAN_POINT('Ctrl Pts',(0.00146041249060754,-0.0374315173641894,
-0.010146497047843));
#41677=CARTESIAN_POINT('Ctrl Pts',(0.00158743526547992,-0.0374209657718817,
-0.0102404804182953));
#41678=CARTESIAN_POINT('Ctrl Pts',(0.00168217860577192,-0.0374122994590536,
-0.0103222379662543));
#41679=CARTESIAN_POINT('Ctrl Pts',(0.00184808696327729,-0.0373960295382161,
-0.0104886427016876));
#41680=CARTESIAN_POINT('Ctrl Pts',(0.00192054560524107,-0.0373884391069072,
-0.0105716049076001));
#41681=CARTESIAN_POINT('Ctrl Pts',(0.00203242463859123,-0.0373759954816367,
-0.0107181906946309));
#41682=CARTESIAN_POINT('Ctrl Pts',(0.00207488578225504,-0.0373710568226065,
-0.0107792929077976));
#41683=CARTESIAN_POINT('Ctrl Pts',(0.00213548411650259,-0.0373636609840927,
-0.010875374279836));
#41684=CARTESIAN_POINT('Ctrl Pts',(0.00215562283752787,-0.0373611350396869,
-0.0109090350207436));
#41685=CARTESIAN_POINT('Ctrl Pts',(0.00219216590290643,-0.0373564140130751,
-0.0109735114061478));
#41686=CARTESIAN_POINT('Ctrl Pts',(0.00220873293498352,-0.0373542137050769,
-0.0110042235002551));
#41687=CARTESIAN_POINT('Ctrl Pts',(0.00224601787164922,-0.0373491099814727,
-0.0110769461870895));
#41688=CARTESIAN_POINT('Ctrl Pts',(0.00226620921720971,-0.0373462247054723,
-0.0111192127150631));
#41689=CARTESIAN_POINT('Ctrl Pts',(0.00235932290368399,-0.0373322458693659,
-0.0113290937475608));
#41690=CARTESIAN_POINT('Ctrl Pts',(0.0024148994130645,-0.0373217284070465,
-0.0115037873353278));
#41691=CARTESIAN_POINT('Ctrl Pts',(0.00246612169864635,-0.0373065731665948,
-0.0117585075669225));
#41692=CARTESIAN_POINT('Ctrl Pts',(0.00247780866819228,-0.0373020549170756,
-0.0118346838080897));
#41693=CARTESIAN_POINT('Ctrl Pts',(0.00249120017015691,-0.0372944525908288,
-0.0119605087079745));
#41694=CARTESIAN_POINT('Ctrl Pts',(0.00249497607041573,-0.0372914341066806,
-0.0120098855005812));
#41695=CARTESIAN_POINT('Ctrl Pts',(0.00249837305303083,-0.0372868901336898,
-0.0120826935118889));
#41696=CARTESIAN_POINT('Ctrl Pts',(0.00249913499473276,-0.0372854176070781,
-0.0121060618950372));
#41697=CARTESIAN_POINT('Ctrl Pts',(0.00249985636577821,-0.0372829413351572,
-0.0121449081098642));
#41698=CARTESIAN_POINT('Ctrl Pts',(0.00250000000000597,-0.0372819472956257,
-0.0121603809209419));
#41699=CARTESIAN_POINT('Ctrl Pts',(0.0025,-0.0372809459012698,-0.0121758532875225));
#41700=CARTESIAN_POINT('Ctrl Pts',(0.0025,-0.0371551761478877,-0.0121758532865581));
#41701=CARTESIAN_POINT('Ctrl Pts',(0.0025,-0.0371588732405284,-0.012121273544903));
#41702=CARTESIAN_POINT('Ctrl Pts',(0.00249821262887724,-0.0371625322456442,
-0.0120666817557802));
#41703=CARTESIAN_POINT('Ctrl Pts',(0.00249137523274373,-0.037169436287764,
-0.0119624781081467));
#41704=CARTESIAN_POINT('Ctrl Pts',(0.00248663097685343,-0.0371726865236799,
-0.0119128961385677));
#41705=CARTESIAN_POINT('Ctrl Pts',(0.00247600682716946,-0.0371781608138532,
-0.0118285331595566));
#41706=CARTESIAN_POINT('Ctrl Pts',(0.00247086659556786,-0.0371804063271866,
-0.0117936759115406));
#41707=CARTESIAN_POINT('Ctrl Pts',(0.00245866842605222,-0.0371850225114768,
-0.0117215549224501));
#41708=CARTESIAN_POINT('Ctrl Pts',(0.00245149592927497,-0.0371873890689005,
-0.0116843195856719));
#41709=CARTESIAN_POINT('Ctrl Pts',(0.00242945596982218,-0.0371938287839682,
-0.0115824374803436));
#41710=CARTESIAN_POINT('Ctrl Pts',(0.00241285834255083,-0.0371978489164038,
-0.0115181950912784));
#41711=CARTESIAN_POINT('Ctrl Pts',(0.00236758877508944,-0.0372072274110915,
-0.0113679349943336));
#41712=CARTESIAN_POINT('Ctrl Pts',(0.00233675583325947,-0.0372125286275146,
-0.0112826668131943));
#41713=CARTESIAN_POINT('Ctrl Pts',(0.00223673439751916,-0.0372274419122276,
-0.0110469649549369));
#41714=CARTESIAN_POINT('Ctrl Pts',(0.00215715865973339,-0.0372369465789953,
-0.0109014816815006));
#41715=CARTESIAN_POINT('Ctrl Pts',(0.00204737012559697,-0.0372489283153428,
-0.0107408882967017));
#41716=CARTESIAN_POINT('Ctrl Pts',(0.00203050791415675,-0.0372507437279206,
-0.0107171256237146));
#41717=CARTESIAN_POINT('Ctrl Pts',(0.00200144354890014,-0.0372538419051825,
-0.0106776479317048));
#41718=CARTESIAN_POINT('Ctrl Pts',(0.00198946244084735,-0.0372551109401504,
-0.0106617744480759));
#41719=CARTESIAN_POINT('Ctrl Pts',(0.00196228652425008,-0.0372579737976691,
-0.0106266493113335));
#41720=CARTESIAN_POINT('Ctrl Pts',(0.00194699665243246,-0.0372595733141312,
-0.0106074766462316));
#41721=CARTESIAN_POINT('Ctrl Pts',(0.00189505636386408,-0.0372649617863302,
-0.0105442764724628));
#41722=CARTESIAN_POINT('Ctrl Pts',(0.00185717700575608,-0.0372688187012443,
-0.010501286445035));
#41723=CARTESIAN_POINT('Ctrl Pts',(0.001749942780224,-0.0372794653861836,
-0.0103877012494666));
#41724=CARTESIAN_POINT('Ctrl Pts',(0.00167781950046844,-0.0372863362539561,
-0.0103198608063866));
#41725=CARTESIAN_POINT('Ctrl Pts',(0.00149230024038699,-0.0373030559236669,
-0.0101650307748533));
#41726=CARTESIAN_POINT('Ctrl Pts',(0.00137509013877611,-0.0373128341623391,
-0.0100831268389333));
#41727=CARTESIAN_POINT('Ctrl Pts',(0.00120842556643995,-0.0373255623895726,
-0.00998674718971798));
#41728=CARTESIAN_POINT('Ctrl Pts',(0.00116459711126692,-0.0373288114824042,
-0.00996311923557821));
#41729=CARTESIAN_POINT('Ctrl Pts',(0.00108859657512858,-0.0373342844840245,
-0.00992503156688167));
#41730=CARTESIAN_POINT('Ctrl Pts',(0.00105677214308859,-0.0373365298255882,
-0.009909915565667));
#41731=CARTESIAN_POINT('Ctrl Pts',(0.000990049413701822,-0.037341146182647,
-0.00987993516253935));
#41732=CARTESIAN_POINT('Ctrl Pts',(0.00095511085249052,-0.037343513073693,
-0.00986518209169217));
#41733=CARTESIAN_POINT('Ctrl Pts',(0.000858146316598404,-0.0373499552354603,
-0.00982681344070009));
#41734=CARTESIAN_POINT('Ctrl Pts',(0.000795493137252516,-0.0373539774073863,
-0.00980486298231614));
#41735=CARTESIAN_POINT('Ctrl Pts',(0.000645332135951805,-0.0373633624180702,
-0.00975887808433417));
#41736=CARTESIAN_POINT('Ctrl Pts',(0.000557243831091014,-0.0373686679862518,
-0.00973706191922827));
#41737=CARTESIAN_POINT('Ctrl Pts',(0.0003058305787371,-0.0373835749319994,
-0.00968913321034425));
#41738=CARTESIAN_POINT('Ctrl Pts',(0.000140850642591267,-0.0373930696817843,
-0.00967436231927322));
#41739=CARTESIAN_POINT('Ctrl Pts',(-5.35128056789639E-5,-0.0374050410017591,
-0.0096762560079129));
#41740=CARTESIAN_POINT('Ctrl Pts',(-8.26605479173067E-5,-0.0374068576632098,
-0.00967705012508711));
#41741=CARTESIAN_POINT('Ctrl Pts',(-0.000131657307400051,-0.0374099572288557,
-0.0096792431841545));
#41742=CARTESIAN_POINT('Ctrl Pts',(-0.000151515075138346,-0.0374112263696641,
-0.00968036960596051));
#41743=CARTESIAN_POINT('Ctrl Pts',(-0.000195810511243041,-0.0374140884700735,
-0.009683412922291));
#41744=CARTESIAN_POINT('Ctrl Pts',(-0.000220235451106661,-0.0374156871018454,
-0.00968545232238211));
#41745=CARTESIAN_POINT('Ctrl Pts',(-0.00030154221504298,-0.0374210684326458,
-0.00969344656263809));
#41746=CARTESIAN_POINT('Ctrl Pts',(-0.000358246224784456,-0.0374249188587891,
-0.00970099379323162));
#41747=CARTESIAN_POINT('Ctrl Pts',(-0.000511910111394329,-0.0374355387061347,
-0.00972683762022137));
#41748=CARTESIAN_POINT('Ctrl Pts',(-0.000608126794533348,-0.0374423888299507,
-0.00974893952325825));
#41749=CARTESIAN_POINT('Ctrl Pts',(-0.000840134536559872,-0.0374591171587561,
-0.00981690052360707));
#41750=CARTESIAN_POINT('Ctrl Pts',(-0.000973793184968563,-0.0374689245539323,
-0.0098688594032971));
#41751=CARTESIAN_POINT('Ctrl Pts',(-0.00114696659032597,-0.0374816802645159,
-0.00995392934498782));
#41752=CARTESIAN_POINT('Ctrl Pts',(-0.00119098612857973,-0.0374849297068421,
-0.00997721030457246));
#41753=CARTESIAN_POINT('Ctrl Pts',(-0.00126491818064556,-0.0374904030981148,
-0.0100191838732753));
#41754=CARTESIAN_POINT('Ctrl Pts',(-0.00129518282739628,-0.0374926484880039,
-0.0100372222744937));
#41755=CARTESIAN_POINT('Ctrl Pts',(-0.00135721070225358,-0.037497264779268,
-0.0100759921392308));
#41756=CARTESIAN_POINT('Ctrl Pts',(-0.00138890387081183,-0.0374996315596356,
-0.0100968188944574));
#41757=CARTESIAN_POINT('Ctrl Pts',(-0.00147471503162175,-0.0375060729337506,
-0.0101560470139788));
#41758=CARTESIAN_POINT('Ctrl Pts',(-0.0015277986500562,-0.0375100944520712,
-0.0101958951698862));
#41759=CARTESIAN_POINT('Ctrl Pts',(-0.00164951409426047,-0.0375194773767364,
-0.010295076470449));
#41760=CARTESIAN_POINT('Ctrl Pts',(-0.00171662663218259,-0.037524781552225,
-0.0103561245948884));
#41761=CARTESIAN_POINT('Ctrl Pts',(-0.00189633812871021,-0.0375396905317433,
-0.0105384070426369));
#41762=CARTESIAN_POINT('Ctrl Pts',(-0.00200042249383268,-0.037549188460147,
-0.0106673357310069));
#41763=CARTESIAN_POINT('Ctrl Pts',(-0.00210698912535109,-0.0375611631192572,
-0.0108299533617198));
#41764=CARTESIAN_POINT('Ctrl Pts',(-0.00212253870069934,-0.0375629793783563,
-0.0108546117960118));
#41765=CARTESIAN_POINT('Ctrl Pts',(-0.00214796639526064,-0.0375660784922145,
-0.0108965425406685));
#41766=CARTESIAN_POINT('Ctrl Pts',(-0.00215807566547284,-0.0375673475942844,
-0.0109136706492718));
#41767=CARTESIAN_POINT('Ctrl Pts',(-0.00218018720661165,-0.0375702099177524,
-0.0109521765882714));
#41768=CARTESIAN_POINT('Ctrl Pts',(-0.00219208047716474,-0.0375718088180809,
-0.0109736120503907));
#41769=CARTESIAN_POINT('Ctrl Pts',(-0.00223067845967603,-0.0375771923407254,
-0.0110456551904282));
#41770=CARTESIAN_POINT('Ctrl Pts',(-0.00225595930751256,-0.0375810447619402,
-0.0110970016992436));
#41771=CARTESIAN_POINT('Ctrl Pts',(-0.00232000004147967,-0.0375916728465572,
-0.0112391851563366));
#41772=CARTESIAN_POINT('Ctrl Pts',(-0.00235517620199612,-0.0375985293346023,
-0.011331524349454));
#41773=CARTESIAN_POINT('Ctrl Pts',(-0.00242770784773348,-0.0376152551268038,
-0.011562107981696));
#41774=CARTESIAN_POINT('Ctrl Pts',(-0.00245883847305205,-0.0376250536931657,
-0.0117019632134072));
#41775=CARTESIAN_POINT('Ctrl Pts',(-0.0024844539093545,-0.0376378010957612,
-0.0118930689186244));
#41776=CARTESIAN_POINT('Ctrl Pts',(-0.00248959253759177,-0.0376410504460935,
-0.0119425985279008));
#41777=CARTESIAN_POINT('Ctrl Pts',(-0.00249583606199858,-0.0376465237319185,
-0.0120273834302457));
#41778=CARTESIAN_POINT('Ctrl Pts',(-0.00249768041747382,-0.0376487691063079,
-0.0120625674577943));
#41779=CARTESIAN_POINT('Ctrl Pts',(-0.00249996476438387,-0.0376533854055685,
-0.0121356794760301));
#41780=CARTESIAN_POINT('Ctrl Pts',(-0.00250028656929416,-0.0376557522086132,
-0.0121736022524783));
#41781=CARTESIAN_POINT('Ctrl Pts',(-0.00249879901690386,-0.0376621937606823,
-0.0122778612191967));
#41782=CARTESIAN_POINT('Ctrl Pts',(-0.00249521179670208,-0.0376662154288805,
-0.0123441425926648));
#41783=CARTESIAN_POINT('Ctrl Pts',(-0.00248049282331027,-0.0376755988406322,
-0.01250046781423));
#41784=CARTESIAN_POINT('Ctrl Pts',(-0.00246709036810547,-0.0376809033440191,
-0.0125902029941435));
#41785=CARTESIAN_POINT('Ctrl Pts',(-0.00241557344638587,-0.0376958118014755,
-0.0128409311664561));
#41786=CARTESIAN_POINT('Ctrl Pts',(-0.00236633209262211,-0.037705308941086,
-0.0129991290369363));
#41787=CARTESIAN_POINT('Ctrl Pts',(-0.00229047759703111,-0.0377172827691985,
-0.0131781318190623));
#41788=CARTESIAN_POINT('Ctrl Pts',(-0.00227863488235069,-0.037719099127798,
-0.0132047715449294));
#41789=CARTESIAN_POINT('Ctrl Pts',(-0.00225793313474505,-0.0377221983630126,
-0.013249228147586));
#41790=CARTESIAN_POINT('Ctrl Pts',(-0.00224932255905463,-0.0377234674845901,
-0.0132671569228806));
#41791=CARTESIAN_POINT('Ctrl Pts',(-0.00222962310064065,-0.037726329802467,
-0.0133069508639312));
#41792=CARTESIAN_POINT('Ctrl Pts',(-0.00221842571023967,-0.0377279286766415,
-0.013328757514631));
#41793=CARTESIAN_POINT('Ctrl Pts',(-0.00218002910643096,-0.0377333118849348,
-0.0134009029738061));
#41794=CARTESIAN_POINT('Ctrl Pts',(-0.00215142413475836,-0.037737164005625,
-0.0134504696411301));
#41795=CARTESIAN_POINT('Ctrl Pts',(-0.00206890023058864,-0.0377477908518304,
-0.0135827635858914));
#41796=CARTESIAN_POINT('Ctrl Pts',(-0.00201174051928373,-0.0377546463812288,
-0.0136633490866566));
#41797=CARTESIAN_POINT('Ctrl Pts',(-0.00186047090774206,-0.037771372260567,
-0.0138518905558524));
#41798=CARTESIAN_POINT('Ctrl Pts',(-0.00176155656163934,-0.0377811718663155,
-0.0139555670708428));
#41799=CARTESIAN_POINT('Ctrl Pts',(-0.0016169827052835,-0.037793920248975,
-0.0140831668877494));
#41800=CARTESIAN_POINT('Ctrl Pts',(-0.00157868121342839,-0.0377971696079862,
-0.0141149882555724));
#41801=CARTESIAN_POINT('Ctrl Pts',(-0.00151169640836178,-0.0378026429266149,
-0.0141673388985111));
#41802=CARTESIAN_POINT('Ctrl Pts',(-0.0014834836402625,-0.0378048883246053,
-0.0141884430269106));
#41803=CARTESIAN_POINT('Ctrl Pts',(-0.00142399634368329,-0.0378095046931221,
-0.0142310107568261));
#41804=CARTESIAN_POINT('Ctrl Pts',(-0.00139266039688508,-0.0378118715413125,
-0.014252373228893));
#41805=CARTESIAN_POINT('Ctrl Pts',(-0.00130518957296975,-0.0378183132913902,
-0.0143091330755973));
#41806=CARTESIAN_POINT('Ctrl Pts',(-0.00124811122153282,-0.0378223351080318,
-0.0143430223879998));
#41807=CARTESIAN_POINT('Ctrl Pts',(-0.00111000843383108,-0.0378317189635866,
-0.0144177501259986));
#41808=CARTESIAN_POINT('Ctrl Pts',(-0.00102797727352534,-0.0378370237548111,
-0.0144565295488911));
#41809=CARTESIAN_POINT('Ctrl Pts',(-0.000790966835365474,-0.0378519318671046,
-0.014553181938555));
#41810=CARTESIAN_POINT('Ctrl Pts',(-0.000632122048189224,-0.0378614284208444,
-0.0146002560265273));
#41811=CARTESIAN_POINT('Ctrl Pts',(-0.000441183559959953,-0.0378734016368977,
-0.0146367894959463));
#41812=CARTESIAN_POINT('Ctrl Pts',(-0.000412456695076201,-0.0378752180785833,
-0.0146417667613537));
#41813=CARTESIAN_POINT('Ctrl Pts',(-0.000363995871075622,-0.0378783173992866,
-0.0146492927219344));
#41814=CARTESIAN_POINT('Ctrl Pts',(-0.000344307135439707,-0.0378795865208704,
-0.0146521101793716));
#41815=CARTESIAN_POINT('Ctrl Pts',(-0.000300281363758517,-0.0378824487445634,
-0.0146578750295461));
#41816=CARTESIAN_POINT('Ctrl Pts',(-0.000275932602387833,-0.0378840475224937,
-0.014660699744501));
#41817=CARTESIAN_POINT('Ctrl Pts',(-0.000194630029985185,-0.0378894300960542,
-0.0146689220522243));
#41818=CARTESIAN_POINT('Ctrl Pts',(-0.000137535960343696,-0.0378932816601816,
-0.0146727224454632));
#41819=CARTESIAN_POINT('Ctrl Pts',(1.82732687588285E-5,-0.0379039062317722,
-0.0146777337676203));
#41820=CARTESIAN_POINT('Ctrl Pts',(0.000117011318379751,-0.0379107600123903,
-0.0146750625860317));
#41821=CARTESIAN_POINT('Ctrl Pts',(0.000357848769779478,-0.037927486805768,
-0.0146542414179252));
#41822=CARTESIAN_POINT('Ctrl Pts',(0.000499063720456591,-0.0379372890505839,
-0.0146297091561706));
#41823=CARTESIAN_POINT('Ctrl Pts',(0.000685556045182069,-0.0379500398856968,
-0.0145805343784468));
#41824=CARTESIAN_POINT('Ctrl Pts',(0.00073330532711476,-0.037953289248627,
-0.0145664059634975));
#41825=CARTESIAN_POINT('Ctrl Pts',(0.000814069223045794,-0.0379587625282782,
-0.0145398609487416));
#41826=CARTESIAN_POINT('Ctrl Pts',(0.000847299816321274,-0.0379610078847682,
-0.01452815516945));
#41827=CARTESIAN_POINT('Ctrl Pts',(0.000915762129038186,-0.0379656241217229,
-0.0145023995310569));
#41828=CARTESIAN_POINT('Ctrl Pts',(0.000950943986517909,-0.0379679908809522,
-0.0144882424140195));
#41829=CARTESIAN_POINT('Ctrl Pts',(0.00104676196183467,-0.037974432223804,
-0.0144471285193998));
#41830=CARTESIAN_POINT('Ctrl Pts',(0.00110666981507643,-0.0379784537312753,
-0.0144185491562909));
#41831=CARTESIAN_POINT('Ctrl Pts',(0.00124557577588733,-0.0379878366347455,
-0.0143453599483277));
#41832=CARTESIAN_POINT('Ctrl Pts',(0.00132342322323941,-0.0379931407991109,
-0.0142987688448356));
#41833=CARTESIAN_POINT('Ctrl Pts',(0.00153559641294985,-0.0380080498299906,
-0.0141555685708384));
#41834=CARTESIAN_POINT('Ctrl Pts',(0.0016630947242035,-0.0380175478155954,
-0.0140497347548168));
#41835=CARTESIAN_POINT('Ctrl Pts',(0.00179967944347598,-0.0380295225377554,
-0.0139113657945893));
#41836=CARTESIAN_POINT('Ctrl Pts',(0.0018197924881693,-0.0380313387782911,
-0.0138902642335271));
#41837=CARTESIAN_POINT('Ctrl Pts',(0.00185300006796865,-0.0380344378507581,
-0.0138541817268452));
#41838=CARTESIAN_POINT('Ctrl Pts',(0.00186629272081414,-0.0380357069297858,
-0.0138393877928635));
#41839=CARTESIAN_POINT('Ctrl Pts',(0.00189557267062487,-0.0380385691689307,
-0.0138060082244455));
#41840=CARTESIAN_POINT('Ctrl Pts',(0.00191146451086293,-0.0380401680071973,
-0.0137873445789218));
#41841=CARTESIAN_POINT('Ctrl Pts',(0.00196352683298741,-0.0380455511408569,
-0.0137243480187127));
#41842=CARTESIAN_POINT('Ctrl Pts',(0.00199844765754735,-0.038049403225228,
-0.0136790098110857));
#41843=CARTESIAN_POINT('Ctrl Pts',(0.00208929641697335,-0.0380600298762508,
-0.0135522924201939));
#41844=CARTESIAN_POINT('Ctrl Pts',(0.00214200921302042,-0.038066885250019,
-0.0134687336581958));
#41845=CARTESIAN_POINT('Ctrl Pts',(0.00225866424320271,-0.0380836121429279,
-0.0132570069458657));
#41846=CARTESIAN_POINT('Ctrl Pts',(0.00231681612679142,-0.0380934129021212,
-0.0131260270516478));
#41847=CARTESIAN_POINT('Ctrl Pts',(0.00237967813600566,-0.038106162407578,
-0.0129437141366519));
#41848=CARTESIAN_POINT('Ctrl Pts',(0.00239449724357181,-0.0381094118230363,
-0.012896173927572));
#41849=CARTESIAN_POINT('Ctrl Pts',(0.00241736182664375,-0.0381148851699031,
-0.0128142910200956));
#41850=CARTESIAN_POINT('Ctrl Pts',(0.00242611817960691,-0.0381171305421612,
-0.0127801642324504));
#41851=CARTESIAN_POINT('Ctrl Pts',(0.00244279591400892,-0.0381217467913269,
-0.0127089441033296));
#41852=CARTESIAN_POINT('Ctrl Pts',(0.00245060043938598,-0.0381241135474091,
-0.0126718325405866));
#41853=CARTESIAN_POINT('Ctrl Pts',(0.00246973111666688,-0.0381305548329474,
-0.0125693375517378));
#41854=CARTESIAN_POINT('Ctrl Pts',(0.00247930384723672,-0.0381345762890585,
-0.0125036568012529));
#41855=CARTESIAN_POINT('Ctrl Pts',(0.00249541115062034,-0.0381437677413351,
-0.0123506985764858));
#41856=CARTESIAN_POINT('Ctrl Pts',(0.00249999999997759,-0.0381488885800515,
-0.0122633067332957));
#41857=CARTESIAN_POINT('Ctrl Pts',(0.0025,-0.0381539840246788,-0.0121758532871986));
#41858=CARTESIAN_POINT('Origin',(0.,-0.0397787743898723,-0.0121758532865581));
#41859=CARTESIAN_POINT('',(0.0025,-0.0410787743898723,-0.0121758532865581));
#41860=CARTESIAN_POINT('Ctrl Pts',(0.0025,-0.0410787743898723,-0.0121758532865581));
#41861=CARTESIAN_POINT('Ctrl Pts',(0.0025,-0.0410787743898723,-0.0128288629739675));
#41862=CARTESIAN_POINT('Ctrl Pts',(0.00222759672557515,-0.0410787754263847,
-0.0134795746236003));
#41863=CARTESIAN_POINT('Ctrl Pts',(0.00170270298531027,-0.0410787748338191,
-0.01401101416509));
#41864=CARTESIAN_POINT('Ctrl Pts',(0.00163307252212577,-0.0410787748546467,
-0.0140737931571262));
#41865=CARTESIAN_POINT('Ctrl Pts',(0.00112277204735936,-0.0410787754415589,
-0.0144808811151188));
#41866=CARTESIAN_POINT('Ctrl Pts',(0.000559471036736449,-0.0410787782045595,
-0.0146719896977074));
#41867=CARTESIAN_POINT('Ctrl Pts',(-0.000187047541110501,-0.0410787758560658,
-0.0146778823060338));
#41868=CARTESIAN_POINT('Ctrl Pts',(-0.000374485721687926,-0.0410787757252281,
-0.014658497162392));
#41869=CARTESIAN_POINT('Ctrl Pts',(-0.00101199045659152,-0.041078775974969,
-0.014513111446229));
#41870=CARTESIAN_POINT('Ctrl Pts',(-0.00143610269325865,-0.0410787774094811,
-0.0142704576596842));
#41871=CARTESIAN_POINT('Ctrl Pts',(-0.00196496964495242,-0.0410787753961375,
-0.0137449744512443));
#41872=CARTESIAN_POINT('Ctrl Pts',(-0.00213246263452953,-0.0410787751295836,
-0.0135142982090746));
#41873=CARTESIAN_POINT('Ctrl Pts',(-0.00241637084585988,-0.0410787750762288,
-0.0129245209925911));
#41874=CARTESIAN_POINT('Ctrl Pts',(-0.00249713293482234,-0.0410787754775941,
-0.0125483842109252));
#41875=CARTESIAN_POINT('Ctrl Pts',(-0.00249776121147513,-0.0410787759848237,
-0.0118033367512004));
#41876=CARTESIAN_POINT('Ctrl Pts',(-0.00241756107791694,-0.0410787755114441,
-0.0114267889635422));
#41877=CARTESIAN_POINT('Ctrl Pts',(-0.00213348624334714,-0.0410787752677254,
-0.0108367968316592));
#41878=CARTESIAN_POINT('Ctrl Pts',(-0.00196556467943907,-0.0410787753518017,
-0.0106062063041865));
#41879=CARTESIAN_POINT('Ctrl Pts',(-0.00143571657760741,-0.0410787772765541,
-0.0100815865218018));
#41880=CARTESIAN_POINT('Ctrl Pts',(-0.00101147589656772,-0.0410787759052714,
-0.00984010203688117));
#41881=CARTESIAN_POINT('Ctrl Pts',(-0.00037429365328496,-0.041078774977993,
-0.00969482154357104));
#41882=CARTESIAN_POINT('Ctrl Pts',(-0.000186977209885448,-0.0410787748267238,
-0.00967530739438422));
#41883=CARTESIAN_POINT('Ctrl Pts',(0.000559246821395463,-0.0410787755265359,
-0.00968032969550766));
#41884=CARTESIAN_POINT('Ctrl Pts',(0.00112319433023955,-0.0410787747030648,
-0.00987028964463931));
#41885=CARTESIAN_POINT('Ctrl Pts',(0.00163370320205056,-0.0410787748872101,
-0.010277362013647));
#41886=CARTESIAN_POINT('Ctrl Pts',(0.00170331323667582,-0.0410787749410509,
-0.0103401241140352));
#41887=CARTESIAN_POINT('Ctrl Pts',(0.00222825340530501,-0.0410787756766175,
-0.0108717944914544));
#41888=CARTESIAN_POINT('Ctrl Pts',(0.0025,-0.0410787743898723,-0.0115228435991487));
#41889=CARTESIAN_POINT('Ctrl Pts',(0.0025,-0.0410787743898723,-0.0121758532865581));
#41890=CARTESIAN_POINT('',(0.00250000000001,-0.0397787743898823,-0.0121758532865581));
#41891=CARTESIAN_POINT('',(0.0025,-0.0397787743898723,-0.0121758532865581));
#41892=CARTESIAN_POINT('',(-0.0025,-0.0397787743898723,-0.0121758532865581));
#41893=CARTESIAN_POINT('Origin',(0.,-0.0397787743898823,-0.0121758532865581));
#41894=CARTESIAN_POINT('',(0.00249999934544701,-0.0392787743898823,-0.0121740442081995));
#41895=CARTESIAN_POINT('Ctrl Pts',(-0.0025,-0.0397787743898823,-0.0121758532865575));
#41896=CARTESIAN_POINT('Ctrl Pts',(-0.00249999999999988,-0.0397478427471941,
-0.0116900920949362));
#41897=CARTESIAN_POINT('Ctrl Pts',(-0.00235413749876254,-0.0397169111045061,
-0.0112043658373873));
#41898=CARTESIAN_POINT('Ctrl Pts',(-0.00208674577744029,-0.039685979461818,
-0.010799084584003));
#41899=CARTESIAN_POINT('Ctrl Pts',(-0.00199394577425234,-0.0396752444378394,
-0.0106584291388004));
#41900=CARTESIAN_POINT('Ctrl Pts',(-0.0018869550846095,-0.0396645094138609,
-0.0105273175393106));
#41901=CARTESIAN_POINT('Ctrl Pts',(-0.00176808672695887,-0.0396537743898823,
-0.0104084061654391));
#41902=CARTESIAN_POINT('Ctrl Pts',(-0.00143189695686255,-0.0396234130278288,
-0.010072094734594));
#41903=CARTESIAN_POINT('Ctrl Pts',(-0.000995398673130767,-0.0395930516657754,
-0.00983346644714466));
#41904=CARTESIAN_POINT('Ctrl Pts',(-0.000529138176708866,-0.0395626903037219,
-0.00973249232469651));
#41905=CARTESIAN_POINT('Ctrl Pts',(-0.000355522219299805,-0.0395513849991087,
-0.00969489377393592));
#41906=CARTESIAN_POINT('Ctrl Pts',(-0.000178043485081894,-0.0395400796944955,
-0.00967591754185142));
#41907=CARTESIAN_POINT('Ctrl Pts',(-9.04539238496386E-7,-0.0395287743898823,
-0.00967585345019635));
#41908=CARTESIAN_POINT('Ctrl Pts',(0.000474817243811614,-0.0394984130278289,
-0.00967568132657733));
#41909=CARTESIAN_POINT('Ctrl Pts',(0.000952258454684218,-0.0394680516657754,
-0.00981561710386961));
#41910=CARTESIAN_POINT('Ctrl Pts',(0.00135331081152122,-0.0394376903037219,
-0.0100738185943088));
#41911=CARTESIAN_POINT('Ctrl Pts',(0.00150264597810249,-0.0394263849991087,
-0.0101699620576968));
#41912=CARTESIAN_POINT('Ctrl Pts',(0.00164153365230363,-0.0394150796944955,
-0.010281989457779));
#41913=CARTESIAN_POINT('Ctrl Pts',(0.00176680728390159,-0.0394037743898823,
-0.0104071271852207));
#41914=CARTESIAN_POINT('Ctrl Pts',(0.00210955958854106,-0.0393728427471942,
-0.0107495076521303));
#41915=CARTESIAN_POINT('Ctrl Pts',(0.00235052058641601,-0.0393419111045061,
-0.0111953350141756));
#41916=CARTESIAN_POINT('Ctrl Pts',(0.00244859938587972,-0.039310979461818,
-0.0116715110937272));
#41917=CARTESIAN_POINT('Ctrl Pts',(0.00248263825910249,-0.0393002444378395,
-0.0118367710407515));
#41918=CARTESIAN_POINT('Ctrl Pts',(0.00249987735095609,-0.0392895094138609,
-0.0120054577310056));
#41919=CARTESIAN_POINT('Ctrl Pts',(0.00249999934544701,-0.0392787743898823,
-0.0121740442081995));
#41920=CARTESIAN_POINT('',(0.0025,-0.0391527785395309,-0.0121758533085357));
#41921=CARTESIAN_POINT('',(0.0025,-0.0397787743898723,-0.0121758532865581));
#41922=CARTESIAN_POINT('',(-0.00175719004339858,-0.0397787743898823,-0.0139541342405783));
#41923=CARTESIAN_POINT('Ctrl Pts',(0.0025,-0.0391527785410365,-0.0121758533086393));
#41924=CARTESIAN_POINT('Ctrl Pts',(0.00250000000061648,-0.039157582660636,
-0.0121060562114304));
#41925=CARTESIAN_POINT('Ctrl Pts',(0.00249707701919054,-0.0391624234467435,
-0.0120362772125198));
#41926=CARTESIAN_POINT('Ctrl Pts',(0.00247960951818523,-0.0391768568469155,
-0.011828220973911));
#41927=CARTESIAN_POINT('Ctrl Pts',(0.002456456148426,-0.0391863646039281,
-0.0116909370520127));
#41928=CARTESIAN_POINT('Ctrl Pts',(0.002409695504752,-0.0391988343180563,
-0.0115081439464148));
#41929=CARTESIAN_POINT('Ctrl Pts',(0.00239595042780696,-0.0392020761857502,
-0.011460388200149));
#41930=CARTESIAN_POINT('Ctrl Pts',(0.00237002275056489,-0.0392075459337757,
-0.0113794629250897));
#41931=CARTESIAN_POINT('Ctrl Pts',(0.00235854421671177,-0.039209794925704,
-0.0113460853524034));
#41932=CARTESIAN_POINT('Ctrl Pts',(0.00233320281379181,-0.0392144275131173,
-0.0112771774626844));
#41933=CARTESIAN_POINT('Ctrl Pts',(0.0023192259424744,-0.039216806785421,
-0.0112416986552508));
#41934=CARTESIAN_POINT('Ctrl Pts',(0.00227839175432255,-0.0392233114884375,
-0.011144618391072));
#41935=CARTESIAN_POINT('Ctrl Pts',(0.00224985360101651,-0.0392273822427032,
-0.0110837570181563));
#41936=CARTESIAN_POINT('Ctrl Pts',(0.00217632142479415,-0.0392369158138843,
-0.0109420926119364));
#41937=CARTESIAN_POINT('Ctrl Pts',(0.00212922984753439,-0.0392423186708913,
-0.0108624904440866));
#41938=CARTESIAN_POINT('Ctrl Pts',(0.00198798533245351,-0.0392571089857904,
-0.0106513784799449));
#41939=CARTESIAN_POINT('Ctrl Pts',(0.00188533583113448,-0.0392664049750631,
-0.0105261243297593));
#41940=CARTESIAN_POINT('Ctrl Pts',(0.00175044921612559,-0.0392781688516613,
-0.0103906911892844));
#41941=CARTESIAN_POINT('Ctrl Pts',(0.00172919128789605,-0.0392800118854489,
-0.0103700920938546));
#41942=CARTESIAN_POINT('Ctrl Pts',(0.00169304079938588,-0.0392831383282574,
-0.0103362857389185));
#41943=CARTESIAN_POINT('Ctrl Pts',(0.00167834749159793,-0.0392844071890178,
-0.0103228703984346));
#41944=CARTESIAN_POINT('Ctrl Pts',(0.00164555616250351,-0.0392872375810382,
-0.010293641188445));
#41945=CARTESIAN_POINT('Ctrl Pts',(0.00162738882544127,-0.0392888041220506,
-0.0102779115138656));
#41946=CARTESIAN_POINT('Ctrl Pts',(0.00156726690162972,-0.0392939753712362,
-0.0102273545174884));
#41947=CARTESIAN_POINT('Ctrl Pts',(0.00152440145952903,-0.0392976419304811,
-0.0101936392959742));
#41948=CARTESIAN_POINT('Ctrl Pts',(0.00140738385367027,-0.0393075288652982,
-0.0101076420849578));
#41949=CARTESIAN_POINT('Ctrl Pts',(0.00133142975461876,-0.0393138201152119,
-0.0100579485359475));
#41950=CARTESIAN_POINT('Ctrl Pts',(0.00111758497766121,-0.0393309440465368,
-0.00993409667149849));
#41951=CARTESIAN_POINT('Ctrl Pts',(0.000975146505137239,-0.0393417046139173,
-0.00986856683695444));
#41952=CARTESIAN_POINT('Ctrl Pts',(0.000780868114425284,-0.0393553150878084,
-0.00980041918618019));
#41953=CARTESIAN_POINT('Ctrl Pts',(0.000733758235032195,-0.0393585404214021,
-0.0097854471325298));
#41954=CARTESIAN_POINT('Ctrl Pts',(0.000652590928776104,-0.0393639742761535,
-0.00976227729419006));
#41955=CARTESIAN_POINT('Ctrl Pts',(0.000618750022325753,-0.039366204060264,
-0.00975338087215502));
#41956=CARTESIAN_POINT('Ctrl Pts',(0.000548145929854338,-0.0393707865604291,
-0.00973639595912972));
#41957=CARTESIAN_POINT('Ctrl Pts',(0.000511364294928023,-0.0393731352315771,
-0.009728421407159));
#41958=CARTESIAN_POINT('Ctrl Pts',(0.000409976828297761,-0.0393795142486738,
-0.00970882543898236));
#41959=CARTESIAN_POINT('Ctrl Pts',(0.000345069813037825,-0.0393834925148775,
-0.00969891258161475));
#41960=CARTESIAN_POINT('Ctrl Pts',(0.000191138965591627,-0.0393927497783937,
-0.00968157297597101));
#41961=CARTESIAN_POINT('Ctrl Pts',(0.000101959255066238,-0.0393979733445863,
-0.00967633853530567));
#41962=CARTESIAN_POINT('Ctrl Pts',(-0.00014852370566438,-0.039412557863015,
-0.00967506733469505));
#41963=CARTESIAN_POINT('Ctrl Pts',(-0.000309417849968945,-0.0394218125435577,
-0.00968984467637572));
#41964=CARTESIAN_POINT('Ctrl Pts',(-0.000499477094730154,-0.0394336652202432,
-0.00972604394515474));
#41965=CARTESIAN_POINT('Ctrl Pts',(-0.000531083223092435,-0.0394356683107231,
-0.00973270090407705));
#41966=CARTESIAN_POINT('Ctrl Pts',(-0.000582085813717356,-0.0394389657075573,
-0.00974447957669038));
#41967=CARTESIAN_POINT('Ctrl Pts',(-0.000601566286691135,-0.0394402407870793,
-0.00974922599894935));
#41968=CARTESIAN_POINT('Ctrl Pts',(-0.000643057067412867,-0.0394429934231556,
-0.00975986555950009));
#41969=CARTESIAN_POINT('Ctrl Pts',(-0.000665047190610122,-0.0394444741367174,
-0.00976582605996293));
#41970=CARTESIAN_POINT('Ctrl Pts',(-0.000731128519181098,-0.039448983630436,
-0.00978471086953718));
#41971=CARTESIAN_POINT('Ctrl Pts',(-0.000774945934629837,-0.0394520547474661,
-0.00979855036092699));
#41972=CARTESIAN_POINT('Ctrl Pts',(-0.000882895035253787,-0.0394597845898461,
-0.00983594691946712));
#41973=CARTESIAN_POINT('Ctrl Pts',(-0.000946489559851482,-0.03946448478577,
-0.00986094031605689));
#41974=CARTESIAN_POINT('Ctrl Pts',(-0.00118754901785606,-0.0394827049763967,
-0.0099672746063182));
#41975=CARTESIAN_POINT('Ctrl Pts',(-0.00135631330578544,-0.0394962618798542,
-0.0100666995735911));
#41976=CARTESIAN_POINT('Ctrl Pts',(-0.00155044208003037,-0.0395123546487842,
-0.0102140981798258));
#41977=CARTESIAN_POINT('Ctrl Pts',(-0.0015882212972613,-0.0395155177431289,
-0.0102445564757565));
#41978=CARTESIAN_POINT('Ctrl Pts',(-0.00165182610085897,-0.03952090229862,
-0.0102989653830152));
#41979=CARTESIAN_POINT('Ctrl Pts',(-0.00167807518874211,-0.0395231430151491,
-0.0103223966430386));
#41980=CARTESIAN_POINT('Ctrl Pts',(-0.00173210405914562,-0.0395277992113981,
-0.0103727145876207));
#41981=CARTESIAN_POINT('Ctrl Pts',(-0.00175977257632255,-0.0395302095095703,
-0.0103997073555977));
#41982=CARTESIAN_POINT('Ctrl Pts',(-0.00183593877314693,-0.0395369308692806,
-0.0104775412168436));
#41983=CARTESIAN_POINT('Ctrl Pts',(-0.00188293669064766,-0.0395411808870754,
-0.0105298017389423));
#41984=CARTESIAN_POINT('Ctrl Pts',(-0.0019911769682663,-0.0395513192102645,
-0.0106608746375088));
#41985=CARTESIAN_POINT('Ctrl Pts',(-0.00205002389018882,-0.0395571354131304,
-0.0107415069289753));
#41986=CARTESIAN_POINT('Ctrl Pts',(-0.00218152261675665,-0.0395713160882073,
-0.0109463776956109));
#41987=CARTESIAN_POINT('Ctrl Pts',(-0.00224856694586445,-0.0395796423988666,
-0.0110737692938842));
#41988=CARTESIAN_POINT('Ctrl Pts',(-0.00231654710161025,-0.0395903992507804,
-0.0112353174285732));
#41989=CARTESIAN_POINT('Ctrl Pts',(-0.00232824743724487,-0.0395923615412376,
-0.0112646662379435));
#41990=CARTESIAN_POINT('Ctrl Pts',(-0.00234661026791289,-0.0395956447079986,
-0.0113133918707819));
#41991=CARTESIAN_POINT('Ctrl Pts',(-0.00235359620816925,-0.0395969484893898,
-0.0113326425769288));
#41992=CARTESIAN_POINT('Ctrl Pts',(-0.00236837108914986,-0.0395998323509752,
-0.0113749715857738));
#41993=CARTESIAN_POINT('Ctrl Pts',(-0.00237606016619275,-0.0396014169637098,
-0.011398080121452));
#41994=CARTESIAN_POINT('Ctrl Pts',(-0.00239958952059697,-0.0396065380962115,
-0.0114724020050694));
#41995=CARTESIAN_POINT('Ctrl Pts',(-0.00241411993927983,-0.0396101312131657,
-0.0115240115177225));
#41996=CARTESIAN_POINT('Ctrl Pts',(-0.00244811160213753,-0.039619739318698,
-0.011661550405884));
#41997=CARTESIAN_POINT('Ctrl Pts',(-0.00246470954775051,-0.0396258172288196,
-0.0117481107294897));
#41998=CARTESIAN_POINT('Ctrl Pts',(-0.00249739404152034,-0.0396423625611843,
-0.011985855689533));
#41999=CARTESIAN_POINT('Ctrl Pts',(-0.00250432617195534,-0.0396527653776538,
-0.012137938927484));
#42000=CARTESIAN_POINT('Ctrl Pts',(-0.0024951616966148,-0.0396660382162044,
-0.0123389309042198));
#42001=CARTESIAN_POINT('Ctrl Pts',(-0.00249146429441867,-0.039669247594065,
-0.0123880616758106));
#42002=CARTESIAN_POINT('Ctrl Pts',(-0.0024825925406336,-0.0396747068144292,
-0.0124725101522114));
#42003=CARTESIAN_POINT('Ctrl Pts',(-0.0024781095303846,-0.0396769762231178,
-0.0125078839745554));
#42004=CARTESIAN_POINT('Ctrl Pts',(-0.00246710611757726,-0.0396816966597413,
-0.0125819655751408));
#42005=CARTESIAN_POINT('Ctrl Pts',(-0.0024604277244359,-0.0396841423026736,
-0.0126206402665768));
#42006=CARTESIAN_POINT('Ctrl Pts',(-0.00243895887099843,-0.0396909914559501,
-0.0127296010944704));
#42007=CARTESIAN_POINT('Ctrl Pts',(-0.00242204630631484,-0.0396953310741771,
-0.0127994316595031));
#42008=CARTESIAN_POINT('Ctrl Pts',(-0.00237375112622782,-0.0397057137609527,
-0.0129669369278575));
#42009=CARTESIAN_POINT('Ctrl Pts',(-0.00233932099393189,-0.039711679882097,
-0.0130635956338083));
#42010=CARTESIAN_POINT('Ctrl Pts',(-0.00224325251832436,-0.0397259061316189,
-0.0132885067680261));
#42011=CARTESIAN_POINT('Ctrl Pts',(-0.00217642517413692,-0.0397341336360773,
-0.0134141361583159));
#42012=CARTESIAN_POINT('Ctrl Pts',(-0.00208213379415691,-0.0397447853638204,
-0.0135599481538735));
#42013=CARTESIAN_POINT('Ctrl Pts',(-0.00206446305273776,-0.0397467484546398,
-0.0135861695037583));
#42014=CARTESIAN_POINT('Ctrl Pts',(-0.00203588021800161,-0.0397498848631493,
-0.013626894556479));
#42015=CARTESIAN_POINT('Ctrl Pts',(-0.0020252987736522,-0.0397510380483964,
-0.0136416274365659));
#42016=CARTESIAN_POINT('Ctrl Pts',(-0.00200222590653047,-0.0397535388409107,
-0.0136730256730993));
#42017=CARTESIAN_POINT('Ctrl Pts',(-0.00198968521731073,-0.0397548901755503,
-0.0136896519358763));
#42018=CARTESIAN_POINT('Ctrl Pts',(-0.00196306243452417,-0.0397577396944162,
-0.0137240457234404));
#42019=CARTESIAN_POINT('Ctrl Pts',(-0.00194894313828253,-0.0397592401013026,
-0.0137417825646316));
#42020=CARTESIAN_POINT('Ctrl Pts',(-0.00187891197293792,-0.0397666201559316,
-0.0138273422379145));
#42021=CARTESIAN_POINT('Ctrl Pts',(-0.00181970175645458,-0.0397726701680068,
-0.0138923639339491));
#42022=CARTESIAN_POINT('Ctrl Pts',(-0.00175719004339085,-0.0397787743898682,
-0.0139541342405719));
#42023=CARTESIAN_POINT('Origin',(0.,-0.0397787743898823,-0.0121758532865581));
#42024=CARTESIAN_POINT('Ctrl Pts',(0.00190999122146646,-0.0443987860946598,
-0.0121758532865581));
#42025=CARTESIAN_POINT('Ctrl Pts',(0.00190999122146646,-0.0443987860946598,
-0.0116043852298449));
#42026=CARTESIAN_POINT('Ctrl Pts',(0.00136395817994342,-0.0443987860946598,
-0.0104664540336249));
#42027=CARTESIAN_POINT('Ctrl Pts',(-0.000486152278277537,-0.0443987860946598,
-0.0100448265867138));
#42028=CARTESIAN_POINT('Ctrl Pts',(-0.00197136065961974,-0.0443987860946598,
-0.011227004012724));
#42029=CARTESIAN_POINT('Ctrl Pts',(-0.00196862385650474,-0.0443987860946598,
-0.0131236069817994));
#42030=CARTESIAN_POINT('Ctrl Pts',(-0.000487368329395306,-0.0443987860946598,
-0.0143095653443973));
#42031=CARTESIAN_POINT('Ctrl Pts',(0.00136371609385951,-0.0443987860946598,
-0.0138834237073105));
#42032=CARTESIAN_POINT('Ctrl Pts',(0.00190999122146646,-0.0443987860946598,
-0.0127473213432713));
#42033=CARTESIAN_POINT('Ctrl Pts',(0.00190999122146646,-0.0443987860946598,
-0.0121758532865581));
#42034=CARTESIAN_POINT('Ctrl Pts',(0.00192589049556924,-0.0443775867868491,
-0.0121758532865581));
#42035=CARTESIAN_POINT('Ctrl Pts',(0.00192589049556924,-0.0443775867868491,
-0.0115996636724157));
#42036=CARTESIAN_POINT('Ctrl Pts',(0.00137529606726147,-0.0443775867868491,
-0.0104522153996155));
#42037=CARTESIAN_POINT('Ctrl Pts',(-0.00049019777087024,-0.0443775867868491,
-0.0100270982797518));
#42038=CARTESIAN_POINT('Ctrl Pts',(-0.00198775342676737,-0.0443775867868491,
-0.0112191060568122));
#42039=CARTESIAN_POINT('Ctrl Pts',(-0.00198501288010718,-0.0443775867868491,
-0.0131315025932785));
#42040=CARTESIAN_POINT('Ctrl Pts',(-0.000491416389901987,-0.0443775867868491,
-0.0143272981564294));
#42041=CARTESIAN_POINT('Ctrl Pts',(0.00137505627975056,-0.0443775867868491,
-0.0138976586778796));
#42042=CARTESIAN_POINT('Ctrl Pts',(0.00192589049556924,-0.0443775867868491,
-0.0127520429007005));
#42043=CARTESIAN_POINT('Ctrl Pts',(0.00192589049556924,-0.0443775867868491,
-0.0121758532865581));
#42044=CARTESIAN_POINT('Ctrl Pts',(0.00195438435881241,-0.0443409038628781,
-0.0121758532865581));
#42045=CARTESIAN_POINT('Ctrl Pts',(0.00195438435881241,-0.0443409038628781,
-0.0115910933812226));
#42046=CARTESIAN_POINT('Ctrl Pts',(0.00139566437443473,-0.0443409038628781,
-0.0104267256068493));
#42047=CARTESIAN_POINT('Ctrl Pts',(-0.000497452079284101,-0.0443409038628781,
-0.00999529310352459));
#42048=CARTESIAN_POINT('Ctrl Pts',(-0.00201718480527981,-0.0443409038628781,
-0.0112049501630331));
#42049=CARTESIAN_POINT('Ctrl Pts',(-0.00201437932167482,-0.044340903862878,
-0.0131456335630356));
#42050=CARTESIAN_POINT('Ctrl Pts',(-0.000498698406502515,-0.0443409038628781,
-0.0143591659955113));
#42051=CARTESIAN_POINT('Ctrl Pts',(0.00139541551284433,-0.044340903862878,
-0.0139231065486815));
#42052=CARTESIAN_POINT('Ctrl Pts',(0.00195438435881241,-0.0443409038628781,
-0.0127606131918936));
#42053=CARTESIAN_POINT('Ctrl Pts',(0.00195438435881241,-0.0443409038628781,
-0.0121758532865581));
#42054=CARTESIAN_POINT('Ctrl Pts',(0.00201714899795489,-0.0442974094567112,
-0.0121758532865581));
#42055=CARTESIAN_POINT('Ctrl Pts',(0.00201714899795489,-0.0442974094567112,
-0.0115723431648622));
#42056=CARTESIAN_POINT('Ctrl Pts',(0.00144047261468403,-0.0442974094567112,
-0.0103705452165039));
#42057=CARTESIAN_POINT('Ctrl Pts',(-0.000513426520915583,-0.0442974094567112,
-0.00992527387087597));
#42058=CARTESIAN_POINT('Ctrl Pts',(-0.00208195197224179,-0.0442974094567112,
-0.0111737702411527));
#42059=CARTESIAN_POINT('Ctrl Pts',(-0.00207907206613982,-0.0442974094567112,
-0.0131767830034219));
#42060=CARTESIAN_POINT('Ctrl Pts',(-0.000514706653486131,-0.0442974094567112,
-0.0144292589295152));
#42061=CARTESIAN_POINT('Ctrl Pts',(0.00144021931264795,-0.0442974094567112,
-0.0139792362605124));
#42062=CARTESIAN_POINT('Ctrl Pts',(0.00201714899795489,-0.0442974094567112,
-0.0127793634082539));
#42063=CARTESIAN_POINT('Ctrl Pts',(0.00201714899795489,-0.0442974094567112,
-0.0121758532865581));
#42064=CARTESIAN_POINT('Ctrl Pts',(0.00208710243564359,-0.0442779618954001,
-0.0121758532865581));
#42065=CARTESIAN_POINT('Ctrl Pts',(0.00208710243564359,-0.0442779618954001,
-0.0115513767164868));
#42066=CARTESIAN_POINT('Ctrl Pts',(0.00149044407485555,-0.0442779618954001,
-0.0103079478417784));
#42067=CARTESIAN_POINT('Ctrl Pts',(-0.000531233254498119,-0.0442779618954001,
-0.00984721379520205));
#42068=CARTESIAN_POINT('Ctrl Pts',(-0.00215417088504416,-0.0442779618954001,
-0.0111390181009185));
#42069=CARTESIAN_POINT('Ctrl Pts',(-0.00215117120441165,-0.0442779618954001,
-0.0132114880644132));
#42070=CARTESIAN_POINT('Ctrl Pts',(-0.00053256567848247,-0.0442779618954001,
-0.0145074356744791));
#42071=CARTESIAN_POINT('Ctrl Pts',(0.00149017747918706,-0.0442779618954001,
-0.0140417547899323));
#42072=CARTESIAN_POINT('Ctrl Pts',(0.00208710243564359,-0.0442779618954001,
-0.0128003298566294));
#42073=CARTESIAN_POINT('Ctrl Pts',(0.00208710243564359,-0.0442779618954001,
-0.0121758532865581));
#42074=CARTESIAN_POINT('Ctrl Pts',(0.00213645587150032,-0.0442788243925216,
-0.0121758532865581));
#42075=CARTESIAN_POINT('Ctrl Pts',(0.00213645587150032,-0.0442788243925216,
-0.0115366816146531));
#42076=CARTESIAN_POINT('Ctrl Pts',(0.00152565591062824,-0.0442788243925216,
-0.0102637592345077));
#42077=CARTESIAN_POINT('Ctrl Pts',(-0.00054379248925872,-0.0442788243925216,
-0.00979217086851526));
#42078=CARTESIAN_POINT('Ctrl Pts',(-0.002205075151519,-0.0442788243925216,
-0.0111145012429317));
#42079=CARTESIAN_POINT('Ctrl Pts',(-0.00220204305666343,-0.0442788243925216,
-0.013235990244785));
#42080=CARTESIAN_POINT('Ctrl Pts',(-0.000545141135798698,-0.0442788243925216,
-0.0145625120797918));
#42081=CARTESIAN_POINT('Ctrl Pts',(0.00152539173851854,-0.0442788243925216,
-0.0140859193992423));
#42082=CARTESIAN_POINT('Ctrl Pts',(0.00213645587150032,-0.0442788243925216,
-0.0128150249584631));
#42083=CARTESIAN_POINT('Ctrl Pts',(0.00213645587150032,-0.0442788243925216,
-0.0121758532865581));
#42084=CARTESIAN_POINT('Ctrl Pts',(0.00215952697976718,-0.0442787673768399,
-0.0121758532865581));
#42085=CARTESIAN_POINT('Ctrl Pts',(0.00215952697976718,-0.0442787673768399,
-0.0115296965823474));
#42086=CARTESIAN_POINT('Ctrl Pts',(0.00154216857972284,-0.0442787673768399,
-0.0102431322722294));
#42087=CARTESIAN_POINT('Ctrl Pts',(-0.000549667972357268,-0.0442787673768399,
-0.00976640454250539));
#42088=CARTESIAN_POINT('Ctrl Pts',(-0.00222892774721398,-0.0442787673768399,
-0.0111030387336221));
#42089=CARTESIAN_POINT('Ctrl Pts',(-0.00222581851868729,-0.0442787673768399,
-0.0132474238346592));
#42090=CARTESIAN_POINT('Ctrl Pts',(-0.000551048797835124,-0.0442787673768399,
-0.0145883521636443));
#42091=CARTESIAN_POINT('Ctrl Pts',(0.00154189149668708,-0.0442787673768399,
-0.0141064975077928));
#42092=CARTESIAN_POINT('Ctrl Pts',(0.00215952697976718,-0.0442787673768399,
-0.0128220099907686));
#42093=CARTESIAN_POINT('Ctrl Pts',(0.00215952697976718,-0.0442787673768399,
-0.0121758532865581));
#42094=CARTESIAN_POINT('',(0.00215000000001,-0.0442787743898723,-0.0121758532865581));
#42095=CARTESIAN_POINT('',(0.00191,-0.0443987743898723,-0.0121758532865581));
#42096=CARTESIAN_POINT('Ctrl Pts',(0.00215000000001,-0.0442787743898723,
-0.0121758532865581));
#42097=CARTESIAN_POINT('Ctrl Pts',(0.00213012938819229,-0.0442787743898723,
-0.0121758532865581));
#42098=CARTESIAN_POINT('Ctrl Pts',(0.00208390361990812,-0.0442788511892961,
-0.0121758532865581));
#42099=CARTESIAN_POINT('Ctrl Pts',(0.00201714899795489,-0.0442974094567112,
-0.0121758532865581));
#42100=CARTESIAN_POINT('Ctrl Pts',(0.00195438855983192,-0.0443409009516712,
-0.0121758532865581));
#42101=CARTESIAN_POINT('Ctrl Pts',(0.00192589648945146,-0.0443775790706037,
-0.0121758532865581));
#42102=CARTESIAN_POINT('Ctrl Pts',(0.00191,-0.0443987743898723,-0.0121758532865581));
#42103=CARTESIAN_POINT('',(-0.00215000000001046,-0.0442787744046664,-0.0121758532865581));
#42104=CARTESIAN_POINT('Origin',(0.,-0.0442787743898823,-0.0121758532865581));
#42105=CARTESIAN_POINT('',(-0.00190884695691278,-0.0443979099384254,-0.0121758531596464));
#42106=CARTESIAN_POINT('Ctrl Pts',(-0.00215000000001053,-0.0442787744120635,
-0.0121758532865581));
#42107=CARTESIAN_POINT('Ctrl Pts',(-0.00212945708742072,-0.0442787748951294,
-0.0121758575253048));
#42108=CARTESIAN_POINT('Ctrl Pts',(-0.00210900073339659,-0.0442787255022982,
-0.012175855287986));
#42109=CARTESIAN_POINT('Ctrl Pts',(-0.00208844214891447,-0.0442812121748871,
-0.0121758544076401));
#42110=CARTESIAN_POINT('Ctrl Pts',(-0.00206193243021586,-0.0442844186695213,
-0.0121758532724587));
#42111=CARTESIAN_POINT('Ctrl Pts',(-0.00203525272905052,-0.044291841976487,
-0.0121758543935678));
#42112=CARTESIAN_POINT('Ctrl Pts',(-0.00201079104512614,-0.0443040605875159,
-0.0121758543850288));
#42113=CARTESIAN_POINT('Ctrl Pts',(-0.00199244478218284,-0.0443132245457876,
-0.0121758543786247));
#42114=CARTESIAN_POINT('Ctrl Pts',(-0.00197534615393758,-0.0443250858625948,
-0.0121758537367935));
#42115=CARTESIAN_POINT('Ctrl Pts',(-0.0019603454088488,-0.0443386005552682,
-0.0121758540374385));
#42116=CARTESIAN_POINT('Ctrl Pts',(-0.00194061637249586,-0.0443563751298959,
-0.012175854432848));
#42117=CARTESIAN_POINT('Ctrl Pts',(-0.00192451617246681,-0.0443770096495027,
-0.0121758564585159));
#42118=CARTESIAN_POINT('Ctrl Pts',(-0.00190884695647826,-0.0443979099380992,
-0.0121758537542897));
#42119=CARTESIAN_POINT('Ctrl Pts',(0.00191,-0.0443987743898723,-0.0121758532865581));
#42120=CARTESIAN_POINT('Ctrl Pts',(0.00191,-0.0443987743898723,-0.0116769538853774));
#42121=CARTESIAN_POINT('Ctrl Pts',(0.00170286569430852,-0.0443979141034954,
-0.0111791984316711));
#42122=CARTESIAN_POINT('Ctrl Pts',(0.00130148688929984,-0.0443984059277294,
-0.0107730760513384));
#42123=CARTESIAN_POINT('Ctrl Pts',(0.00124824039806454,-0.0443984214812156,
-0.0107250730699049));
#42124=CARTESIAN_POINT('Ctrl Pts',(0.00085820319796886,-0.0443983102877573,
-0.0104139306476503));
#42125=CARTESIAN_POINT('Ctrl Pts',(0.000427365466200854,-0.0443970919325886,
-0.0102678966017304));
#42126=CARTESIAN_POINT('Ctrl Pts',(-0.000142889419619194,-0.0443981275956193,
-0.0102649171393808));
#42127=CARTESIAN_POINT('Ctrl Pts',(-0.000285989619838265,-0.0443981683922595,
-0.0102798769391036));
#42128=CARTESIAN_POINT('Ctrl Pts',(-0.000772950241023675,-0.0443979823563326,
-0.0103907749516927));
#42129=CARTESIAN_POINT('Ctrl Pts',(-0.00109761918967261,-0.0443972656261806,
-0.0105748535622802));
#42130=CARTESIAN_POINT('Ctrl Pts',(-0.00150220109501196,-0.0443982715496484,
-0.0109762745220466));
#42131=CARTESIAN_POINT('Ctrl Pts',(-0.00163050456530604,-0.0443983785168756,
-0.0111525082295191));
#42132=CARTESIAN_POINT('Ctrl Pts',(-0.00184765159456686,-0.0443983257609707,
-0.0116033854086035));
#42133=CARTESIAN_POINT('Ctrl Pts',(-0.00190905487174541,-0.0443980661033178,
-0.011891145752726));
#42134=CARTESIAN_POINT('Ctrl Pts',(-0.00190884695778182,-0.0443979099390777,
-0.0121758519703597));
#42135=CARTESIAN_POINT('Origin',(0.,-0.0397787743898723,-0.0121758532865581));
#42136=CARTESIAN_POINT('Ctrl Pts',(0.00249999935903926,-0.0392790584006181,
-0.0121740630901204));
#42137=CARTESIAN_POINT('Ctrl Pts',(0.00250007956807936,-0.0392713094448282,
-0.012286074568086));
#42138=CARTESIAN_POINT('Ctrl Pts',(0.00249263173726238,-0.0392635731967025,
-0.0123979738977816));
#42139=CARTESIAN_POINT('Ctrl Pts',(0.00246733605361282,-0.0392507422192454,
-0.0125861025581287));
#42140=CARTESIAN_POINT('Ctrl Pts',(0.00245337573639674,-0.0392455676519652,
-0.0126626809130144));
#42141=CARTESIAN_POINT('Ctrl Pts',(0.00242690245496861,-0.0392379021202853,
-0.0127772936630157));
#42142=CARTESIAN_POINT('Ctrl Pts',(0.00241701327554165,-0.0392353348903791,
-0.0128158791978145));
#42143=CARTESIAN_POINT('Ctrl Pts',(0.00239672010907757,-0.0392305673004155,
-0.0128878608886453));
#42144=CARTESIAN_POINT('Ctrl Pts',(0.00238652922805646,-0.0392283609778843,
-0.0129213065325673));
#42145=CARTESIAN_POINT('Ctrl Pts',(0.00236149140120812,-0.0392233368771582,
-0.0129976937533472));
#42146=CARTESIAN_POINT('Ctrl Pts',(0.00234616858500414,-0.039220534776043,
-0.0130404669269349));
#42147=CARTESIAN_POINT('Ctrl Pts',(0.00226003621061368,-0.0392060584453356,
-0.0132617162607692));
#42148=CARTESIAN_POINT('Ctrl Pts',(0.00217000806586963,-0.0391950378577499,
-0.0134320111981609));
#42149=CARTESIAN_POINT('Ctrl Pts',(0.00201939095886307,-0.0391795000751182,
-0.0136515108509263));
#42150=CARTESIAN_POINT('Ctrl Pts',(0.001974710770261,-0.0391751414655364,
-0.0137107869249371));
#42151=CARTESIAN_POINT('Ctrl Pts',(0.00189662176439386,-0.0391677668860012,
-0.0138053229027469));
#42152=CARTESIAN_POINT('Ctrl Pts',(0.00186470340147605,-0.0391648115905817,
-0.0138417542234014));
#42153=CARTESIAN_POINT('Ctrl Pts',(0.00181595056253204,-0.0391603430353711,
-0.0138942427919207));
#42154=CARTESIAN_POINT('Ctrl Pts',(0.00179991605181313,-0.0391588801778623,
-0.0139110308136084));
#42155=CARTESIAN_POINT('Ctrl Pts',(0.00176968858466169,-0.0391561294940817,
-0.0139418089392524));
#42156=CARTESIAN_POINT('Ctrl Pts',(0.00175555814557438,-0.0391548459258268,
-0.0139558568103638));
#42157=CARTESIAN_POINT('Ctrl Pts',(0.00171877666747503,-0.0391515130272924,
-0.0139915594081504));
#42158=CARTESIAN_POINT('Ctrl Pts',(0.00169588416679098,-0.0391494468417173,
-0.0140129593355787));
#42159=CARTESIAN_POINT('Ctrl Pts',(0.00156497778349947,-0.0391377063619642,
-0.0141307986675549));
#42160=CARTESIAN_POINT('Ctrl Pts',(0.00144915290219264,-0.0391276145863704,
-0.0142181357359344));
#42161=CARTESIAN_POINT('Ctrl Pts',(0.00124177240671048,-0.0391106849498419,
-0.0143479435805051));
#42162=CARTESIAN_POINT('Ctrl Pts',(0.0011540096266945,-0.0391038192518612,
-0.0143958171422466));
#42163=CARTESIAN_POINT('Ctrl Pts',(0.00100002238319515,-0.0390923647016948,
-0.0144682085245878));
#42164=CARTESIAN_POINT('Ctrl Pts',(0.000935196404764055,-0.0390877081392731,
-0.0144954106791712));
#42165=CARTESIAN_POINT('Ctrl Pts',(0.000833290456592871,-0.0390806405583546,
-0.0145332040180072));
#42166=CARTESIAN_POINT('Ctrl Pts',(0.000796971231267928,-0.0390781693712407,
-0.0145457293540501));
#42167=CARTESIAN_POINT('Ctrl Pts',(0.000727247850065306,-0.0390735116960162,
-0.0145679903896269));
#42168=CARTESIAN_POINT('Ctrl Pts',(0.000693901295168457,-0.0390713209172959,
-0.0145778754633805));
#42169=CARTESIAN_POINT('Ctrl Pts',(0.000614470762973968,-0.0390661832913899,
-0.0145996291119793));
#42170=CARTESIAN_POINT('Ctrl Pts',(0.000568232114567011,-0.0390632561072837,
-0.0146108843492146));
#42171=CARTESIAN_POINT('Ctrl Pts',(0.000327463267891536,-0.0390482919685742,
-0.0146622588559959));
#42172=CARTESIAN_POINT('Ctrl Pts',(0.000128987277406619,-0.0390369544908499,
-0.0146804112996346));
#42173=CARTESIAN_POINT('Ctrl Pts',(-0.00013624320578099,-0.0390214374052796,
-0.0146730294698443));
#42174=CARTESIAN_POINT('Ctrl Pts',(-0.000202829421000357,-0.039017503716378,
-0.0146685045567991));
#42175=CARTESIAN_POINT('Ctrl Pts',(-0.000314071396957006,-0.039010757905199,
-0.014656458185455));
#42176=CARTESIAN_POINT('Ctrl Pts',(-0.00035884877449846,-0.0390079946155222,
-0.0146503771852284));
#42177=CARTESIAN_POINT('Ctrl Pts',(-0.000425699956247967,-0.0390037646428949,
-0.0146394459046998));
#42178=CARTESIAN_POINT('Ctrl Pts',(-0.000447914917421691,-0.0390023415399719,
-0.0146355039081018));
#42179=CARTESIAN_POINT('Ctrl Pts',(-0.000489906582527642,-0.0389996132008413,
-0.0146274648684539));
#42180=CARTESIAN_POINT('Ctrl Pts',(-0.000509692497781764,-0.0389983110649594,
-0.014623427853502));
#42181=CARTESIAN_POINT('Ctrl Pts',(-0.000561475282717601,-0.0389948629593587,
-0.0146122072997597));
#42182=CARTESIAN_POINT('Ctrl Pts',(-0.000593382910862238,-0.0389926979182879,
-0.0146046331975596));
#42183=CARTESIAN_POINT('Ctrl Pts',(-0.000735342028510397,-0.0389829107024314,
-0.014567971345772));
#42184=CARTESIAN_POINT('Ctrl Pts',(-0.000843473076475308,-0.0389750425965237,
-0.0145320167176374));
#42185=CARTESIAN_POINT('Ctrl Pts',(-0.00105762428101284,-0.0389590156085835,
-0.0144441729213225));
#42186=CARTESIAN_POINT('Ctrl Pts',(-0.00116319844389065,-0.038950877181691,
-0.0143918894223511));
#42187=CARTESIAN_POINT('Ctrl Pts',(-0.00133129862955095,-0.038937704612051,
-0.0142933055960654));
#42188=CARTESIAN_POINT('Ctrl Pts',(-0.00139605428816112,-0.0389325699374373,
-0.0142511833078515));
#42189=CARTESIAN_POINT('Ctrl Pts',(-0.00149101437166873,-0.0389249507224814,
-0.0141829540249695));
#42190=CARTESIAN_POINT('Ctrl Pts',(-0.00152271138738355,-0.0389223909370783,
-0.0141590142857709));
#42191=CARTESIAN_POINT('Ctrl Pts',(-0.00158117969491548,-0.0389176335877468,
-0.01411262636824));
#42192=CARTESIAN_POINT('Ctrl Pts',(-0.00160807667283415,-0.0389154301516067,
-0.0140903529086273));
#42193=CARTESIAN_POINT('Ctrl Pts',(-0.00166889709263256,-0.0389104069701919,
-0.0140378009404544));
#42194=CARTESIAN_POINT('Ctrl Pts',(-0.00170247926496707,-0.0389076030008652,
-0.0140071455377505));
#42195=CARTESIAN_POINT('Ctrl Pts',(-0.00187108631641443,-0.0388933233397116,
-0.0138445837629436));
#42196=CARTESIAN_POINT('Ctrl Pts',(-0.00199169085157221,-0.038882473030154,
-0.0136986134107762));
#42197=CARTESIAN_POINT('Ctrl Pts',(-0.00213511309275719,-0.0388671234641056,
-0.0134784534504286));
#42198=CARTESIAN_POINT('Ctrl Pts',(-0.00217272740441468,-0.0388627738211867,
-0.0134146953108739));
#42199=CARTESIAN_POINT('Ctrl Pts',(-0.00223013028260811,-0.0388554158594305,
-0.0133067166945462));
#42200=CARTESIAN_POINT('Ctrl Pts',(-0.00225156137082834,-0.0388524674498998,
-0.0132634211630765));
#42201=CARTESIAN_POINT('Ctrl Pts',(-0.00228142560336189,-0.0388480046596076,
-0.0131984173716676));
#42202=CARTESIAN_POINT('Ctrl Pts',(-0.00229083226155805,-0.0388465401001722,
-0.0131771661984361));
#42203=CARTESIAN_POINT('Ctrl Pts',(-0.0023078237096158,-0.0388437758749244,
-0.0131372866748334));
#42204=CARTESIAN_POINT('Ctrl Pts',(-0.00231548232733165,-0.0388424802622809,
-0.013118692571443));
#42205=CARTESIAN_POINT('Ctrl Pts',(-0.00233471859492918,-0.0388390964265217,
-0.0130703411733368));
#42206=CARTESIAN_POINT('Ctrl Pts',(-0.00234595167654181,-0.0388369906162808,
-0.0130404514642194));
#42207=CARTESIAN_POINT('Ctrl Pts',(-0.00240238576789733,-0.0388257181768527,
-0.0128810835140073));
#42208=CARTESIAN_POINT('Ctrl Pts',(-0.00243744521600239,-0.0388161837378341,
-0.0127482718267893));
#42209=CARTESIAN_POINT('Ctrl Pts',(-0.00247958671686932,-0.0387995173401985,
-0.0125111304838851));
#42210=CARTESIAN_POINT('Ctrl Pts',(-0.00249136341631072,-0.0387923783133283,
-0.0124079575189453));
#42211=CARTESIAN_POINT('Ctrl Pts',(-0.00250039193627361,-0.0387805437321716,
-0.0122325258375608));
#42212=CARTESIAN_POINT('Ctrl Pts',(-0.00250098776779624,-0.0387757744929865,
-0.012160575966621));
#42213=CARTESIAN_POINT('Ctrl Pts',(-0.00249712592140333,-0.0387685681693809,
-0.0120498726853318));
#42214=CARTESIAN_POINT('Ctrl Pts',(-0.00249486692454081,-0.0387660679692394,
-0.0120110859425473));
#42215=CARTESIAN_POINT('Ctrl Pts',(-0.00248885666750585,-0.0387613670497003,
-0.0119374903312185));
#42216=CARTESIAN_POINT('Ctrl Pts',(-0.00248527653242043,-0.0387591617555307,
-0.0119026772268701));
#42217=CARTESIAN_POINT('Ctrl Pts',(-0.00247509808725708,-0.0387540039608111,
-0.0118206633971288));
#42218=CARTESIAN_POINT('Ctrl Pts',(-0.00246787867821289,-0.0387510708521218,
-0.0117735528149738));
#42219=CARTESIAN_POINT('Ctrl Pts',(-0.00242367290482959,-0.0387361070637379,
-0.0115315197676855));
#42220=CARTESIAN_POINT('Ctrl Pts',(-0.00236492917918075,-0.0387247693686716,
-0.01134130567534));
#42221=CARTESIAN_POINT('Ctrl Pts',(-0.00225728548916071,-0.0387092614922215,
-0.0110992439397178));
#42222=CARTESIAN_POINT('Ctrl Pts',(-0.00222784071222068,-0.0387053356308295,
-0.0110395653528206));
#42223=CARTESIAN_POINT('Ctrl Pts',(-0.002174480793844,-0.0386985995587368,
-0.0109414826011622));
#42224=CARTESIAN_POINT('Ctrl Pts',(-0.00215183984312562,-0.0386958373978953,
-0.0109024238744217));
#42225=CARTESIAN_POINT('Ctrl Pts',(-0.00211627130687492,-0.0386916032118865,
-0.0108447226817457));
#42226=CARTESIAN_POINT('Ctrl Pts',(-0.00210412606451918,-0.0386901742426793,
-0.0108256065135759));
#42227=CARTESIAN_POINT('Ctrl Pts',(-0.00208063853724313,-0.0386874367707865,
-0.0107897245336473));
#42228=CARTESIAN_POINT('Ctrl Pts',(-0.00206934935287574,-0.0386861313770795,
-0.0107729267776615));
#42229=CARTESIAN_POINT('Ctrl Pts',(-0.00203910020048041,-0.0386826636261566,
-0.010729076997341));
#42230=CARTESIAN_POINT('Ctrl Pts',(-0.00201980615791264,-0.0386804818293827,
-0.0107022610422355));
#42231=CARTESIAN_POINT('Ctrl Pts',(-0.00192376213987685,-0.0386697920474501,
-0.0105742045565931));
#42232=CARTESIAN_POINT('Ctrl Pts',(-0.00183990591172958,-0.0386609769460144,
-0.0104785373654807));
#42233=CARTESIAN_POINT('Ctrl Pts',(-0.00167145740923374,-0.0386446526449844,
-0.0103135818872248));
#42234=CARTESIAN_POINT('Ctrl Pts',(-0.00158887808078922,-0.0386371537149641,
-0.0102426449896635));
#42235=CARTESIAN_POINT('Ctrl Pts',(-0.00144288382669919,-0.038624833354164,
-0.0101329281848067));
#42236=CARTESIAN_POINT('Ctrl Pts',(-0.00138188907811333,-0.0386199287907678,
-0.0100911852048101));
#42237=CARTESIAN_POINT('Ctrl Pts',(-0.00128589870118461,-0.0386125726199831,
-0.0100315597127439));
#42238=CARTESIAN_POINT('Ctrl Pts',(-0.00125218619417094,-0.0386100532991229,
-0.0100116997773888));
#42239=CARTESIAN_POINT('Ctrl Pts',(-0.00118756728797422,-0.0386053402607332,
-0.00997564876379939));
#42240=CARTESIAN_POINT('Ctrl Pts',(-0.00115676144572518,-0.0386031414239712,
-0.00995929759045683));
#42241=CARTESIAN_POINT('Ctrl Pts',(-0.00108374322017955,-0.0385980350429165,
-0.00992247794073592));
#42242=CARTESIAN_POINT('Ctrl Pts',(-0.00104127628996369,-0.0385951457967156,
-0.0099025420612868));
#42243=CARTESIAN_POINT('Ctrl Pts',(-0.00083127565818442,-0.0385812032151748,
-0.00981107878006168));
#42244=CARTESIAN_POINT('Ctrl Pts',(-0.000656832093369744,-0.0385707213511682,
-0.00975681322273996));
#42245=CARTESIAN_POINT('Ctrl Pts',(-0.000402110777389722,-0.0385555872724883,
-0.0097071918123256));
#42246=CARTESIAN_POINT('Ctrl Pts',(-0.000325549435483613,-0.0385510517070664,
-0.00969593416847256));
#42247=CARTESIAN_POINT('Ctrl Pts',(-0.000199207069529726,-0.0385434246152464,
-0.00968330840647957));
#42248=CARTESIAN_POINT('Ctrl Pts',(-0.000149687379126713,-0.0385403993279406,
-0.00967984518520542));
#42249=CARTESIAN_POINT('Ctrl Pts',(-7.67321610441968E-5,-0.0385358478832761,
-0.00967692168347982));
#42250=CARTESIAN_POINT('Ctrl Pts',(-5.33523115760781E-5,-0.0385343750390019,
-0.00967631324554714));
#42251=CARTESIAN_POINT('Ctrl Pts',(-1.00075927420404E-5,-0.0385316124791532,
-0.00967579361941128));
#42252=CARTESIAN_POINT('Ctrl Pts',(9.95362974219692E-6,-0.0385303272352797,
-0.00967579342545424));
#42253=CARTESIAN_POINT('Ctrl Pts',(6.10757741388324E-5,-0.0385270047572596,
-0.00967640513049062));
#42254=CARTESIAN_POINT('Ctrl Pts',(9.22284759683785E-5,-0.0385249510554573,
-0.00967736073363271));
#42255=CARTESIAN_POINT('Ctrl Pts',(0.000270485429823215,-0.0385130625615317,
-0.00968616690447775));
#42256=CARTESIAN_POINT('Ctrl Pts',(0.000416677309051651,-0.0385027956845988,
-0.0097064251323653));
#42257=CARTESIAN_POINT('Ctrl Pts',(0.00065637852069251,-0.0384857874507535,
-0.00976154146567406));
#42258=CARTESIAN_POINT('Ctrl Pts',(0.000751145290130313,-0.0384790112117261,
-0.00978932489190344));
#42259=CARTESIAN_POINT('Ctrl Pts',(0.000909782464449212,-0.0384676725824359,
-0.00984622332900752));
#42260=CARTESIAN_POINT('Ctrl Pts',(0.000974524048473925,-0.0384630452925797,
-0.00987255473353534));
#42261=CARTESIAN_POINT('Ctrl Pts',(0.00107313182191805,-0.0384559984005605,
-0.00991756356609153));
#42262=CARTESIAN_POINT('Ctrl Pts',(0.00110780782329801,-0.0384535202176235,
-0.00993437019305436));
#42263=CARTESIAN_POINT('Ctrl Pts',(0.00117330084286178,-0.0384488355617415,
-0.00996800440018539));
#42264=CARTESIAN_POINT('Ctrl Pts',(0.00120417870502521,-0.0384466250862385,
-0.00998469254098601));
#42265=CARTESIAN_POINT('Ctrl Pts',(0.00127680679537846,-0.0384414152439737,
-0.0100259440369304));
#42266=CARTESIAN_POINT('Ctrl Pts',(0.00131821535169387,-0.0384384364649971,
-0.0100510817409769));
#42267=CARTESIAN_POINT('Ctrl Pts',(0.00152090322710265,-0.0384237633936469,
-0.0101823343308435));
#42268=CARTESIAN_POINT('Ctrl Pts',(0.00167023610750409,-0.0384127130086052,
-0.0103056715560944));
#42269=CARTESIAN_POINT('Ctrl Pts',(0.00185115424463824,-0.038397424953653,
-0.0104942209847853));
#42270=CARTESIAN_POINT('Ctrl Pts',(0.00189637391772476,-0.0383934006193565,
-0.0105453858095551));
#42271=CARTESIAN_POINT('Ctrl Pts',(0.00196839994031086,-0.038386519090943,
-0.0106339363435631));
#42272=CARTESIAN_POINT('Ctrl Pts',(0.0019963711735133,-0.0383837126128927,
-0.0106703275426845));
#42273=CARTESIAN_POINT('Ctrl Pts',(0.00203670928260101,-0.0383794239918355,
-0.0107259102872087));
#42274=CARTESIAN_POINT('Ctrl Pts',(0.00204984193175066,-0.0383779864810876,
-0.0107445366309428));
#42275=CARTESIAN_POINT('Ctrl Pts',(0.00207413791152825,-0.0383752423482606,
-0.0107800164468686));
#42276=CARTESIAN_POINT('Ctrl Pts',(0.00208535471644444,-0.0383739390558308,
-0.0107968303874377));
#42277=CARTESIAN_POINT('Ctrl Pts',(0.00211422121495514,-0.0383704910452267,
-0.0108412587094857));
#42278=CARTESIAN_POINT('Ctrl Pts',(0.00213153355996036,-0.038368327339692,
-0.0108690868658608));
#42279=CARTESIAN_POINT('Ctrl Pts',(0.0022045952139261,-0.0383587912707048,
-0.0109918437103385));
#42280=CARTESIAN_POINT('Ctrl Pts',(0.00225458365770268,-0.0383511896015644,
-0.0110900504934806));
#42281=CARTESIAN_POINT('Ctrl Pts',(0.00234516748123503,-0.0383352666144794,
-0.0113014554234975));
#42282=CARTESIAN_POINT('Ctrl Pts',(0.00238441064520533,-0.0383269647092676,
-0.0114149513149793));
#42283=CARTESIAN_POINT('Ctrl Pts',(0.00243545976366286,-0.0383135840237234,
-0.0116061105628277));
#42284=CARTESIAN_POINT('Ctrl Pts',(0.00245203421202549,-0.0383083996543626,
-0.0116822935060415));
#42285=CARTESIAN_POINT('Ctrl Pts',(0.00247164937571965,-0.0383007302028928,
-0.0117983229972484));
#42286=CARTESIAN_POINT('Ctrl Pts',(0.00247733933720076,-0.0382981678759811,
-0.0118376671647369));
#42287=CARTESIAN_POINT('Ctrl Pts',(0.00248624592811626,-0.0382934158938033,
-0.011911672479033));
#42288=CARTESIAN_POINT('Ctrl Pts',(0.00248968159609899,-0.0382912201389792,
-0.0119462970758275));
#42289=CARTESIAN_POINT('Ctrl Pts',(0.00249590484773491,-0.03828622995467,
-0.0120258927576418));
#42290=CARTESIAN_POINT('Ctrl Pts',(0.00249820182974504,-0.0382834508394078,
-0.0120708906060241));
#42291=CARTESIAN_POINT('Ctrl Pts',(0.00249976069722458,-0.0382794848074351,
-0.0121359058760536));
#42292=CARTESIAN_POINT('Ctrl Pts',(0.0025,-0.0382782729015159,-0.0121558823324649));
#42293=CARTESIAN_POINT('Ctrl Pts',(0.0025,-0.0382770671668707,-0.0121758532865581));
#42294=CARTESIAN_POINT('Ctrl Pts',(0.0025,-0.0381539840246788,-0.0121758532871986));
#42295=CARTESIAN_POINT('Ctrl Pts',(0.00250000000000082,-0.0381541705624727,
-0.0121726517269627));
#42296=CARTESIAN_POINT('Ctrl Pts',(0.00249999385000889,-0.0381543570699,
-0.0121694500843802));
#42297=CARTESIAN_POINT('Ctrl Pts',(0.00249934642527115,-0.0381641720104095,
-0.0120009373131903));
#42298=CARTESIAN_POINT('Ctrl Pts',(0.00248231629253901,-0.038173669900826,
-0.0118361168523468));
#42299=CARTESIAN_POINT('Ctrl Pts',(0.00244330343755171,-0.0381856445063766,
-0.01164564757488));
#42300=CARTESIAN_POINT('Ctrl Pts',(0.00243695525014424,-0.0381874607692292,
-0.0116171953198876));
#42301=CARTESIAN_POINT('Ctrl Pts',(0.00242544100492311,-0.0381905599441513,
-0.0115695269821681));
#42302=CARTESIAN_POINT('Ctrl Pts',(0.00242054054139413,-0.0381918291051899,
-0.0115502502884726));
#42303=CARTESIAN_POINT('Ctrl Pts',(0.00240908659999788,-0.0381946917181867,
-0.0115073453607196));
#42304=CARTESIAN_POINT('Ctrl Pts',(0.00240241509679818,-0.0381962908526318,
-0.0114837530869141));
#42305=CARTESIAN_POINT('Ctrl Pts',(0.00237901490065508,-0.0382016757004568,
-0.0114054221606092));
#42306=CARTESIAN_POINT('Ctrl Pts',(0.00236075440099767,-0.0382055292443022,
-0.0113511632280352));
#42307=CARTESIAN_POINT('Ctrl Pts',(0.00230594736017677,-0.0382161619865515,
-0.0112050987499869));
#42308=CARTESIAN_POINT('Ctrl Pts',(0.00226579512304355,-0.038223022064487,
-0.0111147552809035));
#42309=CARTESIAN_POINT('Ctrl Pts',(0.00215473521105433,-0.0382397446910621,
-0.0109001031759708));
#42310=CARTESIAN_POINT('Ctrl Pts',(0.00207829598423172,-0.0382495365701051,
-0.0107790291376534));
#42311=CARTESIAN_POINT('Ctrl Pts',(0.00196183752924849,-0.0382622776819215,
-0.0106254753901673));
#42312=CARTESIAN_POINT('Ctrl Pts',(0.00193057627244965,-0.0382655269415844,
-0.0105867170657871));
#42313=CARTESIAN_POINT('Ctrl Pts',(0.00187525049488516,-0.0382710002551838,
-0.0105221675060152));
#42314=CARTESIAN_POINT('Ctrl Pts',(0.00185176068022609,-0.0382732457418609,
-0.0104959057687032));
#42315=CARTESIAN_POINT('Ctrl Pts',(0.00180184870494172,-0.0382778624527694,
-0.010442423341932));
#42316=CARTESIAN_POINT('Ctrl Pts',(0.00177534627212186,-0.0382802295509761,
-0.0104152897460699));
#42317=CARTESIAN_POINT('Ctrl Pts',(0.00170079412703607,-0.0382866725179929,
-0.0103423582804202));
#42318=CARTESIAN_POINT('Ctrl Pts',(0.00165152093698755,-0.038290695272157,
-0.010297853219663));
#42319=CARTESIAN_POINT('Ctrl Pts',(0.00153085747719404,-0.0383000819879186,
-0.0101972928071582));
#42320=CARTESIAN_POINT('Ctrl Pts',(0.00145807226607399,-0.0383053886516684,
-0.0101430589585176));
#42321=CARTESIAN_POINT('Ctrl Pts',(0.00124484482363963,-0.0383202943420306,
-0.0100015356982766));
#42322=CARTESIAN_POINT('Ctrl Pts',(0.00109849071249593,-0.0383297869176337,
-0.00992405386014048));
#42323=CARTESIAN_POINT('Ctrl Pts',(0.000918590755929435,-0.0383417559683749,
-0.00985054867963535));
#42324=CARTESIAN_POINT('Ctrl Pts',(0.00089140450199058,-0.0383435729546521,
-0.00983999191742967));
#42325=CARTESIAN_POINT('Ctrl Pts',(0.000845375814920642,-0.0383466728590269,
-0.00982303893141305));
#42326=CARTESIAN_POINT('Ctrl Pts',(0.000826630905350146,-0.0383479420045997,
-0.0098163878867729));
#42327=CARTESIAN_POINT('Ctrl Pts',(0.000784617852132649,-0.0383508037453525,
-0.00980204299940726));
#42328=CARTESIAN_POINT('Ctrl Pts',(0.000761314061312069,-0.0383524020046748,
-0.00979446687441789));
#42329=CARTESIAN_POINT('Ctrl Pts',(0.000683289026682467,-0.0383577809641004,
-0.00977036299646431));
#42330=CARTESIAN_POINT('Ctrl Pts',(0.000628115623028511,-0.0383616293253011,
-0.00975537043930304));
#42331=CARTESIAN_POINT('Ctrl Pts',(0.000476552075874866,-0.0383722407912966,
-0.00971971611300622));
#42332=CARTESIAN_POINT('Ctrl Pts',(0.000379375206622141,-0.0383790844868964,
-0.00970284195134638));
#42333=CARTESIAN_POINT('Ctrl Pts',(0.000139112964132458,-0.0383958160809537,
-0.00967561926094437));
#42334=CARTESIAN_POINT('Ctrl Pts',(-4.37271060656557E-6,-0.0384056330848951,
-0.00967175399304792));
#42335=CARTESIAN_POINT('Ctrl Pts',(-0.000197110386961847,-0.0384183976563063,
-0.00968313874680747));
#42336=CARTESIAN_POINT('Ctrl Pts',(-0.000246709905085807,-0.0384216470531593,
-0.00968755807429891));
#42337=CARTESIAN_POINT('Ctrl Pts',(-0.00033112332366197,-0.0384271201885602,
-0.00969762850313059));
#42338=CARTESIAN_POINT('Ctrl Pts',(-0.000366008573806928,-0.0384293653731207,
-0.00970253999124724));
#42339=CARTESIAN_POINT('Ctrl Pts',(-0.000438200452295828,-0.038433981055254,
-0.00971426485574402));
#42340=CARTESIAN_POINT('Ctrl Pts',(-0.000475479414601754,-0.0384363474363587,
-0.00972119306509451));
#42341=CARTESIAN_POINT('Ctrl Pts',(-0.000577502517495833,-0.038442787034568,
-0.0097425654566891));
#42342=CARTESIAN_POINT('Ctrl Pts',(-0.000641853564258747,-0.0384468072145951,
-0.0097587426400268));
#42343=CARTESIAN_POINT('Ctrl Pts',(-0.000792413387206625,-0.038456186016707,
-0.00980302994649983));
#42344=CARTESIAN_POINT('Ctrl Pts',(-0.000877886642595209,-0.0384614874763449,
-0.00983330639311861));
#42345=CARTESIAN_POINT('Ctrl Pts',(-0.00111423740165229,-0.0384764005485237,
-0.00993178491872894));
#42346=CARTESIAN_POINT('Ctrl Pts',(-0.00126023318113975,-0.0384859047842912,
-0.010010404835257));
#42347=CARTESIAN_POINT('Ctrl Pts',(-0.00142153644882803,-0.038497886085101,
-0.0101191367193451));
#42348=CARTESIAN_POINT('Ctrl Pts',(-0.00144540839605377,-0.0384997014487062,
-0.0101358426708262));
#42349=CARTESIAN_POINT('Ctrl Pts',(-0.00148507293385394,-0.0385027994238487,
-0.0101646462237679));
#42350=CARTESIAN_POINT('Ctrl Pts',(-0.00150102255975954,-0.0385040683017685,
-0.0101765217204181));
#42351=CARTESIAN_POINT('Ctrl Pts',(-0.00153631714380791,-0.0385069305295438,
-0.0102034611765283));
#42352=CARTESIAN_POINT('Ctrl Pts',(-0.00155558383418402,-0.0385085295667161,
-0.0102186205902852));
#42353=CARTESIAN_POINT('Ctrl Pts',(-0.00161908492923169,-0.0385139147863003,
-0.0102701143981229));
#42354=CARTESIAN_POINT('Ctrl Pts',(-0.00166229164401142,-0.038517768838684,
-0.010307682463096));
#42355=CARTESIAN_POINT('Ctrl Pts',(-0.00177645234352948,-0.0385284033171046,
-0.0104140424140648));
#42356=CARTESIAN_POINT('Ctrl Pts',(-0.00184467929833496,-0.0385352646839569,
-0.0104856113857629));
#42357=CARTESIAN_POINT('Ctrl Pts',(-0.00200083375238739,-0.0385519928568928,
-0.0106701633155684));
#42358=CARTESIAN_POINT('Ctrl Pts',(-0.00208365614888532,-0.0385617889204118,
-0.0107870319204679));
#42359=CARTESIAN_POINT('Ctrl Pts',(-0.00218124216654747,-0.0385745342973122,
-0.0109532898898803));
#42360=CARTESIAN_POINT('Ctrl Pts',(-0.0022051569554232,-0.0385777839596734,
-0.010996971609131));
#42361=CARTESIAN_POINT('Ctrl Pts',(-0.00224373895101086,-0.0385832575811734,
-0.0110727320422425));
#42362=CARTESIAN_POINT('Ctrl Pts',(-0.0022590605830719,-0.0385855029874871,
-0.0111044586616928));
#42363=CARTESIAN_POINT('Ctrl Pts',(-0.00228947006757324,-0.0385901191693694,
-0.0111709829646241));
#42364=CARTESIAN_POINT('Ctrl Pts',(-0.00230444704965679,-0.0385924858270522,
-0.0112058215411856));
#42365=CARTESIAN_POINT('Ctrl Pts',(-0.00234343226594881,-0.0385989264635807,
-0.0113025116553677));
#42366=CARTESIAN_POINT('Ctrl Pts',(-0.00236578092009217,-0.0386029473906875,
-0.0113650005976482));
#42367=CARTESIAN_POINT('Ctrl Pts',(-0.00241272021049882,-0.0386123286768818,
-0.01151479666479));
#42368=CARTESIAN_POINT('Ctrl Pts',(-0.00243509935406213,-0.0386176318392299,
-0.0116026978687232));
#42369=CARTESIAN_POINT('Ctrl Pts',(-0.00248467829252718,-0.0386325407226579,
-0.0118538184627112));
#42370=CARTESIAN_POINT('Ctrl Pts',(-0.00250052883380926,-0.038642039492982,
-0.0120187702971199));
#42371=CARTESIAN_POINT('Ctrl Pts',(-0.00249989090737695,-0.0386540149464972,
-0.0122132049603197));
#42372=CARTESIAN_POINT('Ctrl Pts',(-0.00249928546707395,-0.0386558311273124,
-0.012242349006102));
#42373=CARTESIAN_POINT('Ctrl Pts',(-0.00249740964900756,-0.0386589305545246,
-0.0122913561495992));
#42374=CARTESIAN_POINT('Ctrl Pts',(-0.0024964114253466,-0.0386602000629332,
-0.0123112262134441));
#42375=CARTESIAN_POINT('Ctrl Pts',(-0.00249365237209801,-0.0386630644519539,
-0.0123555753639932));
#42376=CARTESIAN_POINT('Ctrl Pts',(-0.00249176821676331,-0.0386646650376619,
-0.0123800424688974));
#42377=CARTESIAN_POINT('Ctrl Pts',(-0.00248428018473284,-0.0386700584900563,
-0.0124615810786516));
#42378=CARTESIAN_POINT('Ctrl Pts',(-0.00247707319844085,-0.0386739194021167,
-0.0125184839774196));
#42379=CARTESIAN_POINT('Ctrl Pts',(-0.00245208809609394,-0.0386845828625149,
-0.0126729338391774));
#42380=CARTESIAN_POINT('Ctrl Pts',(-0.00243045421006269,-0.0386914666641234,
-0.0127697525762979));
#42381=CARTESIAN_POINT('Ctrl Pts',(-0.00236390107356713,-0.0387081694153858,
-0.0130018211908673));
#42382=CARTESIAN_POINT('Ctrl Pts',(-0.00231305860326874,-0.0387179181450143,
-0.0131350304199771));
#42383=CARTESIAN_POINT('Ctrl Pts',(-0.00222950165528394,-0.0387306184707593,
-0.0133080191354538));
#42384=CARTESIAN_POINT('Ctrl Pts',(-0.00220651970562422,-0.0387338669896611,
-0.0133521816792891));
#42385=CARTESIAN_POINT('Ctrl Pts',(-0.00216504003097869,-0.0387393401469098,
-0.0134263905324124));
#42386=CARTESIAN_POINT('Ctrl Pts',(-0.002147197793653,-0.0387415861795271,
-0.0134567840318599));
#42387=CARTESIAN_POINT('Ctrl Pts',(-0.00210881831015474,-0.0387462050882495,
-0.0135191051302542));
#42388=CARTESIAN_POINT('Ctrl Pts',(-0.00208818446062511,-0.0387485738136454,
-0.0135509627648386));
#42389=CARTESIAN_POINT('Ctrl Pts',(-0.00202943520538178,-0.0387550247851162,
-0.0136372948247452));
#42390=CARTESIAN_POINT('Ctrl Pts',(-0.00198985916723715,-0.0387590537203214,
-0.0136907394795097));
#42391=CARTESIAN_POINT('Ctrl Pts',(-0.00189122147994072,-0.0387684592594367,
-0.0138133963399071));
#42392=CARTESIAN_POINT('Ctrl Pts',(-0.00183042108274609,-0.0387737782323989,
-0.0138810881466482));
#42393=CARTESIAN_POINT('Ctrl Pts',(-0.0016494666492127,-0.038788668536376,
-0.0140616948377055));
#42394=CARTESIAN_POINT('Ctrl Pts',(-0.00152166415045526,-0.0387981354467401,
-0.0141662461622445));
#42395=CARTESIAN_POINT('Ctrl Pts',(-0.00136019816630597,-0.0388100776589811,
-0.0142736413717688));
#42396=CARTESIAN_POINT('Ctrl Pts',(-0.00133558637285986,-0.0388118981312168,
-0.0142893959929954));
#42397=CARTESIAN_POINT('Ctrl Pts',(-0.00129376564683746,-0.0388150016437606,
-0.0143151443325941));
#42398=CARTESIAN_POINT('Ctrl Pts',(-0.00127670373178246,-0.0388162708107099,
-0.014325370273962));
#42399=CARTESIAN_POINT('Ctrl Pts',(-0.00123840317315041,-0.0388191287941554,
-0.0143477085349456));
#42400=CARTESIAN_POINT('Ctrl Pts',(-0.00121710719233605,-0.0388207231919584,
-0.0143597139993317));
#42401=CARTESIAN_POINT('Ctrl Pts',(-0.0011457327398832,-0.0388260759543795,
-0.0143985826500701));
#42402=CARTESIAN_POINT('Ctrl Pts',(-0.00109491731420809,-0.0388299012209369,
-0.0144240491060759));
#42403=CARTESIAN_POINT('Ctrl Pts',(-0.000954660070359158,-0.0388404184066393,
-0.0144884566441129));
#42404=CARTESIAN_POINT('Ctrl Pts',(-0.000863735013469948,-0.0388471896278612,
-0.0145239314082387));
#42405=CARTESIAN_POINT('Ctrl Pts',(-0.000633224283974524,-0.0388639605164184,
-0.0145986607716618));
#42406=CARTESIAN_POINT('Ctrl Pts',(-0.000491839383571248,-0.0388738884426874,
-0.0146312704023529));
#42407=CARTESIAN_POINT('Ctrl Pts',(-0.000299115103153614,-0.0388867559307366,
-0.0146583939942214));
#42408=CARTESIAN_POINT('Ctrl Pts',(-0.000249620515464944,-0.0388900053641852,
-0.0146638581836792));
#42409=CARTESIAN_POINT('Ctrl Pts',(-0.00016490382937219,-0.0388954771094111,
-0.0146706570654864));
#42410=CARTESIAN_POINT('Ctrl Pts',(-0.000129757936991223,-0.0388977209113932,
-0.0146727317870172));
#42411=CARTESIAN_POINT('Ctrl Pts',(-5.67420519562254E-5,-0.0389023322616905,
-0.0146754960583138));
#42412=CARTESIAN_POINT('Ctrl Pts',(-1.88765179014198E-5,-0.0389046957291191,
-0.0146760687894049));
#42413=CARTESIAN_POINT('Ctrl Pts',(8.51414429488758E-5,-0.0389111220835623,
-0.0146752786859037));
#42414=CARTESIAN_POINT('Ctrl Pts',(0.000151251255901054,-0.0389151322283889,
-0.0146721506443055));
#42415=CARTESIAN_POINT('Ctrl Pts',(0.000307074464708355,-0.0389244802779819,
-0.0146585636473454));
#42416=CARTESIAN_POINT('Ctrl Pts',(0.000396498523842506,-0.03892976153709,
-0.0146458605141264));
#42417=CARTESIAN_POINT('Ctrl Pts',(0.000648175173277603,-0.038944703853889,
-0.0145960850933967));
#42418=CARTESIAN_POINT('Ctrl Pts',(0.000807661391825655,-0.0389542538528716,
-0.014547629573628));
#42419=CARTESIAN_POINT('Ctrl Pts',(0.000987932963469518,-0.0389662832808593,
-0.0144725533308203));
#42420=CARTESIAN_POINT('Ctrl Pts',(0.00101453239613327,-0.0389680921686267,
-0.0144609280080553));
#42421=CARTESIAN_POINT('Ctrl Pts',(0.00105898316035181,-0.0389711822944906,
-0.0144405716535904));
#42422=CARTESIAN_POINT('Ctrl Pts',(0.00107694326699847,-0.0389724499489362,
-0.0144320863823738));
#42423=CARTESIAN_POINT('Ctrl Pts',(0.0011168732102256,-0.0389753133933625,
-0.0144126360189723));
#42424=CARTESIAN_POINT('Ctrl Pts',(0.00113878447881048,-0.038976914954726,
-0.0144015604911461));
#42425=CARTESIAN_POINT('Ctrl Pts',(0.00121147683354711,-0.0389823216371654,
-0.014363462181737));
#42426=CARTESIAN_POINT('Ctrl Pts',(0.00126148515472098,-0.038986195375057,
-0.0143350112252988));
#42427=CARTESIAN_POINT('Ctrl Pts',(0.00139532051531692,-0.0389969092163965,
-0.0142526319094823));
#42428=CARTESIAN_POINT('Ctrl Pts',(0.00147697606317126,-0.0390038315090007,
-0.0141953753644116));
#42429=CARTESIAN_POINT('Ctrl Pts',(0.00166621912727251,-0.0390205555538059,
-0.0140450485340773));
#42430=CARTESIAN_POINT('Ctrl Pts',(0.00176972424034835,-0.0390302870575528,
-0.013947367539907));
#42431=CARTESIAN_POINT('Ctrl Pts',(0.00189756114235087,-0.0390429736575671,
-0.013804270334125));
#42432=CARTESIAN_POINT('Ctrl Pts',(0.00192962573124047,-0.0390462245870136,
-0.0137661442873352));
#42433=CARTESIAN_POINT('Ctrl Pts',(0.00198239638551046,-0.0390517001987144,
-0.0136994497731451));
#42434=CARTESIAN_POINT('Ctrl Pts',(0.00200367512871736,-0.0390539463436724,
-0.0136713558315795));
#42435=CARTESIAN_POINT('Ctrl Pts',(0.00204660704290472,-0.0390585639141946,
-0.0136121115660901));
#42436=CARTESIAN_POINT('Ctrl Pts',(0.0020681595910738,-0.0390609312232226,
-0.0135808993274417));
#42437=CARTESIAN_POINT('Ctrl Pts',(0.00212544510123207,-0.0390673737801507,
-0.0134937629408868));
#42438=CARTESIAN_POINT('Ctrl Pts',(0.00215967574304779,-0.0390713959738459,
-0.0134368863849838));
#42439=CARTESIAN_POINT('Ctrl Pts',(0.00223523865355963,-0.0390807820641926,
-0.0132992109336272));
#42440=CARTESIAN_POINT('Ctrl Pts',(0.00227451593090324,-0.0390860887191309,
-0.0132173919782099));
#42441=CARTESIAN_POINT('Ctrl Pts',(0.00237247999309516,-0.0391009843188402,
-0.0129811909976451));
#42442=CARTESIAN_POINT('Ctrl Pts',(0.00242044395373002,-0.0391104675045367,
-0.0128228990157841));
#42443=CARTESIAN_POINT('Ctrl Pts',(0.00245812802713222,-0.0391224260989022,
-0.012632425952674));
#42444=CARTESIAN_POINT('Ctrl Pts',(0.00246329091039689,-0.039124244699187,
-0.0126036963861636));
#42445=CARTESIAN_POINT('Ctrl Pts',(0.00247113200339487,-0.0391273492930154,
-0.0125552003768462));
#42446=CARTESIAN_POINT('Ctrl Pts',(0.00247407872878765,-0.0391286215627706,
-0.0125354808750266));
#42447=CARTESIAN_POINT('Ctrl Pts',(0.00248014228871132,-0.0391314966252482,
-0.0124912934162562));
#42448=CARTESIAN_POINT('Ctrl Pts',(0.00248313327375542,-0.0391331052280717,
-0.01246681253051));
#42449=CARTESIAN_POINT('Ctrl Pts',(0.00249193257048902,-0.0391385434541255,
-0.0123847189511998));
#42450=CARTESIAN_POINT('Ctrl Pts',(0.00249610112657119,-0.0391424421493603,
-0.0123269524689338));
#42451=CARTESIAN_POINT('Ctrl Pts',(0.00249942029500609,-0.0391485070700073,
-0.0122380236399158));
#42452=CARTESIAN_POINT('Ctrl Pts',(0.00249999999972546,-0.039150639079543,
-0.0122069366733935));
#42453=CARTESIAN_POINT('Ctrl Pts',(0.0025,-0.0391527785410365,-0.0121758533086393));
#42454=CARTESIAN_POINT('Origin',(0.,-0.0320674495244671,-0.0121758532865581));
#42455=CARTESIAN_POINT('',(0.00199999982444772,-0.0355681130672164,-0.0121766912657388));
#42456=CARTESIAN_POINT('',(0.00199999947635761,-0.0395674495244771,-0.0121744060238692));
#42457=CARTESIAN_POINT('Ctrl Pts',(0.00199999982024451,-0.0355681123252202,
-0.012176701238172));
#42458=CARTESIAN_POINT('Ctrl Pts',(0.00200006372026205,-0.0355794597712501,
-0.0120241914541404));
#42459=CARTESIAN_POINT('Ctrl Pts',(0.00198268576079593,-0.0355906127106426,
-0.0118721885649424));
#42460=CARTESIAN_POINT('Ctrl Pts',(0.00193848766546422,-0.0356055917189111,
-0.0116817755903345));
#42461=CARTESIAN_POINT('Ctrl Pts',(0.00192742358701769,-0.0356089198116543,
-0.0116402368105887));
#42462=CARTESIAN_POINT('Ctrl Pts',(0.00190503977995606,-0.0356150065308702,
-0.0115659157952878));
#42463=CARTESIAN_POINT('Ctrl Pts',(0.00189418901858273,-0.0356177493846711,
-0.0115330096239274));
#42464=CARTESIAN_POINT('Ctrl Pts',(0.00186779778516884,-0.0356239990331276,
-0.0114594567864354));
#42465=CARTESIAN_POINT('Ctrl Pts',(0.00185177489705482,-0.0356275202053536,
-0.0114190034607499));
#42466=CARTESIAN_POINT('Ctrl Pts',(0.00178163648056277,-0.035641937928567,
-0.0112575150145211));
#42467=CARTESIAN_POINT('Ctrl Pts',(0.0017168759052299,-0.0356531670735535,
-0.0111414938200488));
#42468=CARTESIAN_POINT('Ctrl Pts',(0.00158630110163576,-0.0356726271273577,
-0.0109540300345471));
#42469=CARTESIAN_POINT('Ctrl Pts',(0.00152587214325114,-0.035680796332212,
-0.0108793499726965));
#42470=CARTESIAN_POINT('Ctrl Pts',(0.00144138352066207,-0.0356910127280173,
-0.0107890653288063));
#42471=CARTESIAN_POINT('Ctrl Pts',(0.0014220370205924,-0.0356932797316201,
-0.0107692338527021));
#42472=CARTESIAN_POINT('Ctrl Pts',(0.00138807260355076,-0.0356971286291267,
-0.0107358353475258));
#42473=CARTESIAN_POINT('Ctrl Pts',(0.00137365409092878,-0.035698723266576,
-0.0107220748466189));
#42474=CARTESIAN_POINT('Ctrl Pts',(0.00133834199944169,-0.0357025365378354,
-0.0106893688930189));
#42475=CARTESIAN_POINT('Ctrl Pts',(0.00131724931101274,-0.0357047402412553,
-0.0106706457762239));
#42476=CARTESIAN_POINT('Ctrl Pts',(0.00121130063664286,-0.0357154932467055,
-0.0105805331791964));
#42477=CARTESIAN_POINT('Ctrl Pts',(0.00112099543299248,-0.0357236923468493,
-0.0105158318527037));
#42478=CARTESIAN_POINT('Ctrl Pts',(0.000921758513265947,-0.0357408903643568,
-0.010396796125477));
#42479=CARTESIAN_POINT('Ctrl Pts',(0.000812315465694571,-0.0357498646982703,
-0.0103442359697735));
#42480=CARTESIAN_POINT('Ctrl Pts',(0.000659580232080265,-0.0357623763237561,
-0.0102872808846941));
#42481=CARTESIAN_POINT('Ctrl Pts',(0.000619917109655637,-0.0357656222333493,
-0.0102738926916546));
#42482=CARTESIAN_POINT('Ctrl Pts',(0.000546667388170452,-0.0357716313162415,
-0.0102517020323112));
#42483=CARTESIAN_POINT('Ctrl Pts',(0.000513215134607283,-0.0357743809373372,
-0.0102425107890887));
#42484=CARTESIAN_POINT('Ctrl Pts',(0.000436764745341417,-0.0357806864999606,
-0.0102236293904429));
#42485=CARTESIAN_POINT('Ctrl Pts',(0.000393652824776714,-0.0357842578177142,
-0.0102144817173615));
#42486=CARTESIAN_POINT('Ctrl Pts',(0.000240790077661422,-0.0357969897704358,
-0.0101872892550173));
#42487=CARTESIAN_POINT('Ctrl Pts',(0.000129885668804329,-0.0358063652388844,
-0.0101769812420771));
#42488=CARTESIAN_POINT('Ctrl Pts',(-6.11586135789818E-5,-0.0358226233301814,
-0.010175193354002));
#42489=CARTESIAN_POINT('Ctrl Pts',(-0.000141008646280326,-0.0358294462804263,
-0.0101792316712571));
#42490=CARTESIAN_POINT('Ctrl Pts',(-0.000254445753695718,-0.0358390538608624,
-0.0101918093448361));
#42491=CARTESIAN_POINT('Ctrl Pts',(-0.000288385940867445,-0.0358419168192868,
-0.0101964577098354));
#42492=CARTESIAN_POINT('Ctrl Pts',(-0.000349699788095021,-0.0358470510388757,
-0.0102064658446794));
#42493=CARTESIAN_POINT('Ctrl Pts',(-0.000377112774462912,-0.0358493326318625,
-0.0102115307511461));
#42494=CARTESIAN_POINT('Ctrl Pts',(-0.000423932077242514,-0.0358531961727089,
-0.0102211976045163));
#42495=CARTESIAN_POINT('Ctrl Pts',(-0.000443389608732699,-0.0358547912056612,
-0.0102255192136858));
#42496=CARTESIAN_POINT('Ctrl Pts',(-0.000490050054016354,-0.0358585917999575,
-0.0102366172123026));
#42497=CARTESIAN_POINT('Ctrl Pts',(-0.000517180748175394,-0.0358607827895064,
-0.0102436757807234));
#42498=CARTESIAN_POINT('Ctrl Pts',(-0.000652679796783529,-0.0358716721326215,
-0.010281987393025));
#42499=CARTESIAN_POINT('Ctrl Pts',(-0.00075842854558731,-0.035880005855045,
-0.0103218004766724));
#42500=CARTESIAN_POINT('Ctrl Pts',(-0.00096794045489743,-0.0358972030104413,
-0.0104216250891795));
#42501=CARTESIAN_POINT('Ctrl Pts',(-0.00107079616282311,-0.0359060409762,
-0.0104824495340128));
#42502=CARTESIAN_POINT('Ctrl Pts',(-0.00120169692900742,-0.0359184136484365,
-0.01057657635546));
#42503=CARTESIAN_POINT('Ctrl Pts',(-0.00123499658228157,-0.035921668618646,
-0.0106021490013148));
#42504=CARTESIAN_POINT('Ctrl Pts',(-0.0012942905310538,-0.0359276858318921,
-0.0106507255484452));
#42505=CARTESIAN_POINT('Ctrl Pts',(-0.00132053825984378,-0.0359304342716035,
-0.0106733949658894));
#42506=CARTESIAN_POINT('Ctrl Pts',(-0.00137864976963684,-0.0359367251809057,
-0.0107262836388159));
#42507=CARTESIAN_POINT('Ctrl Pts',(-0.00141013315643489,-0.0359402827313761,
-0.0107568919643324));
#42508=CARTESIAN_POINT('Ctrl Pts',(-0.00152408621630788,-0.0359537509296682,
-0.0108752178177149));
#42509=CARTESIAN_POINT('Ctrl Pts',(-0.00159957882847991,-0.0359639230180368,
-0.0109692753529544));
#42510=CARTESIAN_POINT('Ctrl Pts',(-0.00170710264158098,-0.035980475882862,
-0.0111312088692722));
#42511=CARTESIAN_POINT('Ctrl Pts',(-0.0017446018404604,-0.0359867916363548,
-0.0111951154771363));
#42512=CARTESIAN_POINT('Ctrl Pts',(-0.00179356410142959,-0.0359957910075969,
-0.0112902934412212));
#42513=CARTESIAN_POINT('Ctrl Pts',(-0.00180792867997445,-0.0359985452964401,
-0.011320001321169));
#42514=CARTESIAN_POINT('Ctrl Pts',(-0.00183276148622826,-0.0360035101793772,
-0.0113747775774794));
#42515=CARTESIAN_POINT('Ctrl Pts',(-0.00184346673962206,-0.0360057301245718,
-0.0113997298737214));
#42516=CARTESIAN_POINT('Ctrl Pts',(-0.00186115029722121,-0.036009533059476,
-0.0114433798230547));
#42517=CARTESIAN_POINT('Ctrl Pts',(-0.00186836208859691,-0.0360111276722849,
-0.0114619758484414));
#42518=CARTESIAN_POINT('Ctrl Pts',(-0.00188531037198073,-0.036014988136515,
-0.0115076953942276));
#42519=CARTESIAN_POINT('Ctrl Pts',(-0.00189474105435947,-0.0360172377768593,
-0.0115349268048528));
#42520=CARTESIAN_POINT('Ctrl Pts',(-0.00193115712472691,-0.0360264065448639,
-0.0116479195779665));
#42521=CARTESIAN_POINT('Ctrl Pts',(-0.00195293644909198,-0.0360331073892564,
-0.0117352572024554));
#42522=CARTESIAN_POINT('Ctrl Pts',(-0.0019853316361911,-0.0360467624467822,
-0.011916405108863));
#42523=CARTESIAN_POINT('Ctrl Pts',(-0.00199533846551933,-0.036053698626972,
-0.0120100868097281));
#42524=CARTESIAN_POINT('Ctrl Pts',(-0.0020003881931414,-0.0360642836288285,
-0.0121507930589636));
#42525=CARTESIAN_POINT('Ctrl Pts',(-0.00200042786321385,-0.0360678238759117,
-0.0121975048735993));
#42526=CARTESIAN_POINT('Ctrl Pts',(-0.00199740348698823,-0.0360746195085124,
-0.012285989610768));
#42527=CARTESIAN_POINT('Ctrl Pts',(-0.00199466240655691,-0.0360778644388145,
-0.012327748354794));
#42528=CARTESIAN_POINT('Ctrl Pts',(-0.00198725762500653,-0.036083872349982,
-0.0124039108243686));
#42529=CARTESIAN_POINT('Ctrl Pts',(-0.00198300386623346,-0.0360866217990032,
-0.0124383384854523));
#42530=CARTESIAN_POINT('Ctrl Pts',(-0.00197131777385926,-0.0360929277669059,
-0.0125162184114001));
#42531=CARTESIAN_POINT('Ctrl Pts',(-0.00196333996898166,-0.0360964996806398,
-0.0125595689953699));
#42532=CARTESIAN_POINT('Ctrl Pts',(-0.0019300162148669,-0.0361093061827661,
-0.0127121416170955));
#42533=CARTESIAN_POINT('Ctrl Pts',(-0.00189693212423113,-0.0361187599113526,
-0.012819444070496));
#42534=CARTESIAN_POINT('Ctrl Pts',(-0.00182541617002246,-0.0361350437807657,
-0.0129969125567394));
#42535=CARTESIAN_POINT('Ctrl Pts',(-0.00179144520815108,-0.0361418133250543,
-0.013068605977944));
#42536=CARTESIAN_POINT('Ctrl Pts',(-0.0017368920806125,-0.0361513571589629,
-0.0131680075523525));
#42537=CARTESIAN_POINT('Ctrl Pts',(-0.00171971231131524,-0.0361542089908726,
-0.0131974961040721));
#42538=CARTESIAN_POINT('Ctrl Pts',(-0.00168718221683256,-0.0361593258803548,
-0.013250185112041));
#42539=CARTESIAN_POINT('Ctrl Pts',(-0.00167208643035337,-0.0361616011693833,
-0.0132735326120951));
#42540=CARTESIAN_POINT('Ctrl Pts',(-0.00164533981366778,-0.0361654583374121,
-0.0133130665932397));
#42541=CARTESIAN_POINT('Ctrl Pts',(-0.00163392606599862,-0.0361670531549552,
-0.0133294055898316));
#42542=CARTESIAN_POINT('Ctrl Pts',(-0.0016058338486083,-0.0361708590092413,
-0.0133683662851926));
#42543=CARTESIAN_POINT('Ctrl Pts',(-0.00158891961221953,-0.0361730553229059,
-0.0133908118462923));
#42544=CARTESIAN_POINT('Ctrl Pts',(-0.00150226140911318,-0.0361838887961957,
-0.0135009023416009));
#42545=CARTESIAN_POINT('Ctrl Pts',(-0.00142570636290487,-0.0361921672906417,
-0.0135829468599513));
#42546=CARTESIAN_POINT('Ctrl Pts',(-0.00125386045995633,-0.036209348524211,
-0.0137386052476914));
#42547=CARTESIAN_POINT('Ctrl Pts',(-0.00115800658124893,-0.036218226208243,
-0.0138108994262984));
#42548=CARTESIAN_POINT('Ctrl Pts',(-0.00102060073360294,-0.0362306433212439,
-0.0138963585029053));
#42549=CARTESIAN_POINT('Ctrl Pts',(-0.000984248091122991,-0.0362338998993086,
-0.0139174098533958));
#42550=CARTESIAN_POINT('Ctrl Pts',(-0.00091672024282943,-0.0362399186717001,
-0.0139537246461715));
#42551=CARTESIAN_POINT('Ctrl Pts',(-0.000885758358559603,-0.0362426670206583,
-0.013969351100869));
#42552=CARTESIAN_POINT('Ctrl Pts',(-0.000814735762173941,-0.0362489558175553,
-0.0140029085308272));
#42553=CARTESIAN_POINT('Ctrl Pts',(-0.000774460978011599,-0.0362525112998127,
-0.0140203409726528));
#42554=CARTESIAN_POINT('Ctrl Pts',(-0.00062117534750794,-0.0362660197545799,
-0.0140807832834877));
#42555=CARTESIAN_POINT('Ctrl Pts',(-0.000504929781915352,-0.0362762370013897,
-0.0141148360713988));
#42556=CARTESIAN_POINT('Ctrl Pts',(-0.00031400039851391,-0.0362928084016039,
-0.0141524260297192));
#42557=CARTESIAN_POINT('Ctrl Pts',(-0.00024092448432737,-0.0362990974789354,
-0.014162657831295));
#42558=CARTESIAN_POINT('Ctrl Pts',(-0.000134640675424076,-0.0363080646695565,
-0.0141715876893407));
#42559=CARTESIAN_POINT('Ctrl Pts',(-0.000101768181975097,-0.0363108130403072,
-0.0141735337982387));
#42560=CARTESIAN_POINT('Ctrl Pts',(-4.17693200385002E-5,-0.0363157686887946,
-0.014175600804675));
#42561=CARTESIAN_POINT('Ctrl Pts',(-1.46597800301764E-5,-0.0363179852644014,
-0.0141759833116636));
#42562=CARTESIAN_POINT('Ctrl Pts',(3.23980952306466E-5,-0.0363217850113142,
-0.0141756903456227));
#42563=CARTESIAN_POINT('Ctrl Pts',(5.23414829159846E-5,-0.0363233797236368,
-0.0141752677896181));
#42564=CARTESIAN_POINT('Ctrl Pts',(0.000101121151082956,-0.0363272440808545,
-0.0141735037880477));
#42565=CARTESIAN_POINT('Ctrl Pts',(0.000129940499311205,-0.0363294974133465,
-0.0141718364356037));
#42566=CARTESIAN_POINT('Ctrl Pts',(0.000239504866029927,-0.0363379854765585,
-0.0141631141299244));
#42567=CARTESIAN_POINT('Ctrl Pts',(0.000319837839623694,-0.0363440477291476,
-0.0141517771136954));
#42568=CARTESIAN_POINT('Ctrl Pts',(0.000496974397509341,-0.0363574810042967,
-0.0141156880795133));
#42569=CARTESIAN_POINT('Ctrl Pts',(0.000593051196616829,-0.0363648169862106,
-0.0140885038413577));
#42570=CARTESIAN_POINT('Ctrl Pts',(0.000731652186469292,-0.0363758987839011,
-0.0140378350200237));
#42571=CARTESIAN_POINT('Ctrl Pts',(0.000775998466777736,-0.0363795227651278,
-0.0140197938329827));
#42572=CARTESIAN_POINT('Ctrl Pts',(0.000858440401884898,-0.0363864530415998,
-0.013982753471274));
#42573=CARTESIAN_POINT('Ctrl Pts',(0.000896659778307296,-0.0363897477997356,
-0.0139640951468769));
#42574=CARTESIAN_POINT('Ctrl Pts',(0.000964897014594833,-0.0363958025841946,
-0.0139280447441654));
#42575=CARTESIAN_POINT('Ctrl Pts',(0.000995112987960803,-0.0363985477368804,
-0.0139110624957629));
#42576=CARTESIAN_POINT('Ctrl Pts',(0.00106266552078047,-0.0364048421383324,
-0.0138707512482148));
#42577=CARTESIAN_POINT('Ctrl Pts',(0.00109970233186019,-0.0364084067253401,
-0.0138469580969806));
#42578=CARTESIAN_POINT('Ctrl Pts',(0.00123997348430849,-0.0364223726537744,
-0.0137501620768282));
#42579=CARTESIAN_POINT('Ctrl Pts',(0.0013369667065856,-0.0364330687912483,
-0.0136686669071304));
#42580=CARTESIAN_POINT('Ctrl Pts',(0.00149610190982521,-0.0364523943736247,
-0.0135069361771168));
#42581=CARTESIAN_POINT('Ctrl Pts',(0.00156110230431907,-0.0364609645555744,
-0.0134300724832778));
#42582=CARTESIAN_POINT('Ctrl Pts',(0.00163634900559828,-0.036471568196491,
-0.0133261290362688));
#42583=CARTESIAN_POINT('Ctrl Pts',(0.00165217600870689,-0.0364738429721809,
-0.0133032782432026));
#42584=CARTESIAN_POINT('Ctrl Pts',(0.00167852654934271,-0.036477699626104,
-0.0132634864187557));
#42585=CARTESIAN_POINT('Ctrl Pts',(0.00168928124936084,-0.0364792944308592,
-0.0132467062950394));
#42586=CARTESIAN_POINT('Ctrl Pts',(0.00171459537322141,-0.0364831007346985,
-0.0132058788423459));
#42587=CARTESIAN_POINT('Ctrl Pts',(0.00172890187146586,-0.0364852974979562,
-0.0131816805546013));
#42588=CARTESIAN_POINT('Ctrl Pts',(0.00179761640926801,-0.0364961260347862,
-0.0130596543222264));
#42589=CARTESIAN_POINT('Ctrl Pts',(0.0018442609683476,-0.0365043996609087,
-0.0129576698337327));
#42590=CARTESIAN_POINT('Ctrl Pts',(0.00192282970617978,-0.0365216129858041,
-0.012739063849049));
#42591=CARTESIAN_POINT('Ctrl Pts',(0.00195322242421475,-0.0365305277238056,
-0.0126223929710588));
#42592=CARTESIAN_POINT('Ctrl Pts',(0.00197980524934267,-0.0365429744671278,
-0.0124624235186765));
#42593=CARTESIAN_POINT('Ctrl Pts',(0.00198536747266429,-0.0365462199454981,
-0.0124209386791781));
#42594=CARTESIAN_POINT('Ctrl Pts',(0.00199315274703356,-0.0365522284004654,
-0.012344806646019));
#42595=CARTESIAN_POINT('Ctrl Pts',(0.00199578285507167,-0.0365549778312713,
-0.0123102170112996));
#42596=CARTESIAN_POINT('Ctrl Pts',(0.00199970923124176,-0.0365612831174252,
-0.012231571082258));
#42597=CARTESIAN_POINT('Ctrl Pts',(0.00200045121779198,-0.0365648543519947,
-0.0121875067441161));
#42598=CARTESIAN_POINT('Ctrl Pts',(0.00199787936999445,-0.0365778743717673,
-0.0120287527085681));
#42599=CARTESIAN_POINT('Ctrl Pts',(0.00198615585864129,-0.0365875550820124,
-0.0119144382283467));
#42600=CARTESIAN_POINT('Ctrl Pts',(0.00195020696594567,-0.0366039162872233,
-0.0117256297574465));
#42601=CARTESIAN_POINT('Ctrl Pts',(0.00193129384625522,-0.0366105340398136,
-0.0116503884201844));
#42602=CARTESIAN_POINT('Ctrl Pts',(0.00189794514378554,-0.0366198964107415,
-0.011544233682504));
#42603=CARTESIAN_POINT('Ctrl Pts',(0.00188701570073092,-0.0366227162880287,
-0.0115122938507159));
#42604=CARTESIAN_POINT('Ctrl Pts',(0.00186569357881676,-0.0366277834698879,
-0.0114547787914556));
#42605=CARTESIAN_POINT('Ctrl Pts',(0.00185556992208626,-0.0366300407145318,
-0.0114291127388221));
#42606=CARTESIAN_POINT('Ctrl Pts',(0.00183722180171872,-0.0366338800318558,
-0.0113852754187023));
#42607=CARTESIAN_POINT('Ctrl Pts',(0.00182925162866056,-0.0366354746151612,
-0.0113670047917613));
#42608=CARTESIAN_POINT('Ctrl Pts',(0.00180929696405246,-0.0366392973887674,
-0.0113230656920839));
#42609=CARTESIAN_POINT('Ctrl Pts',(0.00179703810793846,-0.0366415103902769,
-0.0112975273427616));
#42610=CARTESIAN_POINT('Ctrl Pts',(0.00173484031386666,-0.0366521513416018,
-0.0111747117790803));
#42611=CARTESIAN_POINT('Ctrl Pts',(0.00167751805348371,-0.0366602404907024,
-0.0110813695613111));
#42612=CARTESIAN_POINT('Ctrl Pts',(0.00154221229859184,-0.0366771959744809,
-0.0108968505532088));
#42613=CARTESIAN_POINT('Ctrl Pts',(0.00146310180609141,-0.0366860378516589,
-0.0108070598422564));
#42614=CARTESIAN_POINT('Ctrl Pts',(0.00134533816331753,-0.0366984779481924,
-0.0106953447984558));
#42615=CARTESIAN_POINT('Ctrl Pts',(0.00131327719910589,-0.0367018000737338,
-0.0106668328586224));
#42616=CARTESIAN_POINT('Ctrl Pts',(0.00125370667310763,-0.0367078813130874,
-0.0106171935308863));
#42617=CARTESIAN_POINT('Ctrl Pts',(0.00122651659506477,-0.0367106248218075,
-0.0105957085450076));
#42618=CARTESIAN_POINT('Ctrl Pts',(0.00116388285386699,-0.036716883315838,
-0.0105488075646894));
#42619=CARTESIAN_POINT('Ctrl Pts',(0.00112813952302434,-0.0367204128576432,
-0.0105238237142059));
#42620=CARTESIAN_POINT('Ctrl Pts',(0.000981421472766178,-0.0367347536325225,
-0.0104282533735347));
#42621=CARTESIAN_POINT('Ctrl Pts',(0.000864438985207459,-0.0367458906898303,
-0.0103675314923803));
#42622=CARTESIAN_POINT('Ctrl Pts',(0.000651008998317222,-0.036765469335323,
-0.0102822146053174));
#42623=CARTESIAN_POINT('Ctrl Pts',(0.000557070931437676,-0.0367738493888426,
-0.0102524823325248));
#42624=CARTESIAN_POINT('Ctrl Pts',(0.000435079241419324,-0.0367841961595787,
-0.0102235640634526));
#42625=CARTESIAN_POINT('Ctrl Pts',(0.000408715479801509,-0.0367864006928543,
-0.0102178749861448));
#42626=CARTESIAN_POINT('Ctrl Pts',(0.000362656642195421,-0.0367901888975908,
-0.0102089068399541));
#42627=CARTESIAN_POINT('Ctrl Pts',(0.000343015162755336,-0.0367917838218753,
-0.010205386629613));
#42628=CARTESIAN_POINT('Ctrl Pts',(0.000294672083937837,-0.0367956614092112,
-0.0101974672831097));
#42629=CARTESIAN_POINT('Ctrl Pts',(0.000265921688213696,-0.0367979274068945,
-0.0101933980596849));
#42630=CARTESIAN_POINT('Ctrl Pts',(0.00011077062147708,-0.0368099910242354,
-0.0101748750056979));
#42631=CARTESIAN_POINT('Ctrl Pts',(-1.6717160445149E-5,-0.0368193305906831,
-0.0101718789178745));
#42632=CARTESIAN_POINT('Ctrl Pts',(-0.000231171361878576,-0.0368352761668842,
-0.0101873208122118));
#42633=CARTESIAN_POINT('Ctrl Pts',(-0.000318186300452089,-0.0368418104483716,
-0.0101993773882134));
#42634=CARTESIAN_POINT('Ctrl Pts',(-0.00045092032500571,-0.0368521353863758,
-0.0102267627141409));
#42635=CARTESIAN_POINT('Ctrl Pts',(-0.000497352755849111,-0.0368558155848458,
-0.0102380909765576));
#42636=CARTESIAN_POINT('Ctrl Pts',(-0.000576916653033613,-0.0368622724481259,
-0.0102605504405343));
#42637=CARTESIAN_POINT('Ctrl Pts',(-0.000610245388870597,-0.0368650239699315,
-0.0102709075957314));
#42638=CARTESIAN_POINT('Ctrl Pts',(-0.000681156106117241,-0.0368709897004767,
-0.0102949954651788));
#42639=CARTESIAN_POINT('Ctrl Pts',(-0.000718630676713551,-0.0368742114057743,
-0.0103089924779559));
#42640=CARTESIAN_POINT('Ctrl Pts',(-0.000831041777317918,-0.0368840994627731,
-0.010354864923161));
#42641=CARTESIAN_POINT('Ctrl Pts',(-0.000904466566600802,-0.0368908714180335,
-0.0103901976627558));
#42642=CARTESIAN_POINT('Ctrl Pts',(-0.000987785497383913,-0.0368989222239252,
-0.0104367509228298));
#42643=CARTESIAN_POINT('Ctrl Pts',(-0.000999972495799115,-0.0369001092775983,
-0.0104437296716397));
#42644=CARTESIAN_POINT('Ctrl Pts',(-0.00109879587062757,-0.0369098109023126,
-0.0105017103330895));
#42645=CARTESIAN_POINT('Ctrl Pts',(-0.00118154606627001,-0.0369184242447914,
-0.0105590491440091));
#42646=CARTESIAN_POINT('Ctrl Pts',(-0.00128919238539798,-0.0369301266041836,
-0.0106463333847669));
#42647=CARTESIAN_POINT('Ctrl Pts',(-0.00131806276453473,-0.0369333187145092,
-0.0106711410037714));
#42648=CARTESIAN_POINT('Ctrl Pts',(-0.00136839499946266,-0.036938959943791,
-0.0107169512809244));
#42649=CARTESIAN_POINT('Ctrl Pts',(-0.0013901252578126,-0.0369414225563398,
-0.0107376419039902));
#42650=CARTESIAN_POINT('Ctrl Pts',(-0.00142543442538057,-0.0369454587846278,
-0.0107728101682445));
#42651=CARTESIAN_POINT('Ctrl Pts',(-0.00143927695279488,-0.0369470500152991,
-0.0107870137439042));
#42652=CARTESIAN_POINT('Ctrl Pts',(-0.00147053087133148,-0.0369506624780771,
-0.0108200522015299));
#42653=CARTESIAN_POINT('Ctrl Pts',(-0.00148779527697202,-0.0369526738235214,
-0.0108390200791985));
#42654=CARTESIAN_POINT('Ctrl Pts',(-0.00155897217816492,-0.0369610613967223,
-0.0109203075463372));
#42655=CARTESIAN_POINT('Ctrl Pts',(-0.00160937733924054,-0.036967241439652,
-0.0109856023280882));
#42656=CARTESIAN_POINT('Ctrl Pts',(-0.00171350945493643,-0.0369810495953943,
-0.0111392555550667));
#42657=CARTESIAN_POINT('Ctrl Pts',(-0.00176470394910575,-0.0369886335850651,
-0.011229032829568));
#42658=CARTESIAN_POINT('Ctrl Pts',(-0.0018294590485119,-0.0370000211949638,
-0.0113662630171804));
#42659=CARTESIAN_POINT('Ctrl Pts',(-0.00184856959207488,-0.0370036944030231,
-0.0114109044497765));
#42660=CARTESIAN_POINT('Ctrl Pts',(-0.00188148061587224,-0.0370107037148611,
-0.0114962409344938));
#42661=CARTESIAN_POINT('Ctrl Pts',(-0.0018956307601921,-0.037014027630454,
-0.0115367713091516));
#42662=CARTESIAN_POINT('Ctrl Pts',(-0.00191882798860973,-0.0370201106104126,
-0.0116107871117771));
#42663=CARTESIAN_POINT('Ctrl Pts',(-0.00192832895619941,-0.0370228540218132,
-0.0116441129603315));
#42664=CARTESIAN_POINT('Ctrl Pts',(-0.00194781330731927,-0.0370291102407018,
-0.0117198685063456));
#42665=CARTESIAN_POINT('Ctrl Pts',(-0.00195728459814625,-0.0370326375550902,
-0.0117624101640019));
#42666=CARTESIAN_POINT('Ctrl Pts',(-0.0019897824076701,-0.0370469995970621,
-0.0119347382856186));
#42667=CARTESIAN_POINT('Ctrl Pts',(-0.00200134048048048,-0.0370581619933841,
-0.0120663288976307));
#42668=CARTESIAN_POINT('Ctrl Pts',(-0.0019988059355266,-0.0370775923151151,
-0.0122944239437779));
#42669=CARTESIAN_POINT('Ctrl Pts',(-0.00199077393651083,-0.0370857986141568,
-0.0123905780112073));
#42670=CARTESIAN_POINT('Ctrl Pts',(-0.00197153582218788,-0.0370960567668822,
-0.0125132221870122));
#42671=CARTESIAN_POINT('Ctrl Pts',(-0.00196666080265298,-0.0370983298646916,
-0.0125405679533566));
#42672=CARTESIAN_POINT('Ctrl Pts',(-0.00195731153504465,-0.0371021848574262,
-0.0125873490594598));
#42673=CARTESIAN_POINT('Ctrl Pts',(-0.00195311386903877,-0.0371037796389771,
-0.0126068330177357));
#42674=CARTESIAN_POINT('Ctrl Pts',(-0.00194229091888752,-0.0371075875064836,
-0.0126536577298692));
#42675=CARTESIAN_POINT('Ctrl Pts',(-0.00193537897328492,-0.0371097858136657,
-0.0126809271075952));
#42676=CARTESIAN_POINT('Ctrl Pts',(-0.00189816994216949,-0.0371205977682293,
-0.0128157192134525));
#42677=CARTESIAN_POINT('Ctrl Pts',(-0.00185947375669505,-0.0371288550220459,
-0.0129207300905785));
#42678=CARTESIAN_POINT('Ctrl Pts',(-0.00176120925056366,-0.0371460665145463,
-0.0131311917990515));
#42679=CARTESIAN_POINT('Ctrl Pts',(-0.00170045076154391,-0.037154995894315,
-0.0132355665520264));
#42680=CARTESIAN_POINT('Ctrl Pts',(-0.00160644511961943,-0.0371674580160518,
-0.0133679459171712));
#42681=CARTESIAN_POINT('Ctrl Pts',(-0.00158115616002576,-0.0371707030051337,
-0.0134012901425602));
#42682=CARTESIAN_POINT('Ctrl Pts',(-0.00153302480183524,-0.0371767110129889,
-0.0134607805598211));
#42683=CARTESIAN_POINT('Ctrl Pts',(-0.00151051139103103,-0.0371794604993252,
-0.0134871725392997));
#42684=CARTESIAN_POINT('Ctrl Pts',(-0.00145786078653481,-0.0371857665470215,
-0.0135457380101189));
#42685=CARTESIAN_POINT('Ctrl Pts',(-0.00142732432145111,-0.0371893385032907,
-0.0135775261818474));
#42686=CARTESIAN_POINT('Ctrl Pts',(-0.00131545127428182,-0.0372021476010341,
-0.0136865361389192));
#42687=CARTESIAN_POINT('Ctrl Pts',(-0.00122870996426901,-0.0372116040285329,
-0.0137578897501099));
#42688=CARTESIAN_POINT('Ctrl Pts',(-0.00107125703818745,-0.0372278887889061,
-0.013866618653536));
#42689=CARTESIAN_POINT('Ctrl Pts',(-0.00100343167043015,-0.0372346564956022,
-0.0139077322759927));
#42690=CARTESIAN_POINT('Ctrl Pts',(-0.000903170860836162,-0.0372441981456313,
-0.0139606351466137));
#42691=CARTESIAN_POINT('Ctrl Pts',(-0.000872593367725354,-0.0372470496030501,
-0.0139757824517772));
#42692=CARTESIAN_POINT('Ctrl Pts',(-0.000816427285820691,-0.0372521659157054,
-0.0140018376941819));
#42693=CARTESIAN_POINT('Ctrl Pts',(-0.000790970096741173,-0.0372544409988147,
-0.014013008452615));
#42694=CARTESIAN_POINT('Ctrl Pts',(-0.000746873103090543,-0.0372582979665442,
-0.0140312717779441));
#42695=CARTESIAN_POINT('Ctrl Pts',(-0.000728347129689305,-0.0372598927847343,
-0.0140386221308174));
#42696=CARTESIAN_POINT('Ctrl Pts',(-0.000683438077299609,-0.037263698846043,
-0.0140556676781315));
#42697=CARTESIAN_POINT('Ctrl Pts',(-0.00065695519819512,-0.0372658953605332,
-0.0140650858965379));
#42698=CARTESIAN_POINT('Ctrl Pts',(-0.000524015625016074,-0.0372767265915936,
-0.0141092298703231));
#42699=CARTESIAN_POINT('Ctrl Pts',(-0.000414960476630937,-0.0372850028772857,
-0.0141355348438161));
#42700=CARTESIAN_POINT('Ctrl Pts',(-0.000185360621513893,-0.0373022167577775,
-0.0141708757046039));
#42701=CARTESIAN_POINT('Ctrl Pts',(-6.50619379126704E-5,-0.0373111293749187,
-0.0141784104682219));
#42702=CARTESIAN_POINT('Ctrl Pts',(9.70094164269938E-5,-0.0373235738184182,
-0.0141739374913336));
#42703=CARTESIAN_POINT('Ctrl Pts',(0.000138792623795986,-0.0373268192916294,
-0.0141714703469583));
#42704=CARTESIAN_POINT('Ctrl Pts',(0.00021500953180113,-0.0373328277511859,
-0.0141645649348134));
#42705=CARTESIAN_POINT('Ctrl Pts',(0.000249464513071551,-0.037335577192105,
-0.0141605372109731));
#42706=CARTESIAN_POINT('Ctrl Pts',(0.000327412140380952,-0.0373418825234562,
-0.0141493635626145));
#42707=CARTESIAN_POINT('Ctrl Pts',(0.000370806766784288,-0.0373454537936954,
-0.0141416720108122));
#42708=CARTESIAN_POINT('Ctrl Pts',(0.000522683727167805,-0.037358183766739,
-0.0141095448719654));
#42709=CARTESIAN_POINT('Ctrl Pts',(0.000629334272877263,-0.0373675572091138,
-0.0140775085577029));
#42710=CARTESIAN_POINT('Ctrl Pts',(0.000807103959575631,-0.0373838155596301,
-0.0140075104228064));
#42711=CARTESIAN_POINT('Ctrl Pts',(0.000879632852575996,-0.0373906408150592,
-0.0139738053109617));
#42712=CARTESIAN_POINT('Ctrl Pts',(0.000980096178100673,-0.0374002511035641,
-0.0139195805664092));
#42713=CARTESIAN_POINT('Ctrl Pts',(0.0010098187561663,-0.037403114511219,
-0.0139025378901922));
#42714=CARTESIAN_POINT('Ctrl Pts',(0.0010629075960811,-0.0374082493948992,
-0.0138702571393256));
#42715=CARTESIAN_POINT('Ctrl Pts',(0.0010864209962758,-0.0374105312083792,
-0.0138552777780935));
#42716=CARTESIAN_POINT('Ctrl Pts',(0.00112619627987677,-0.0374143948753308,
-0.0138287535047519));
#42717=CARTESIAN_POINT('Ctrl Pts',(0.00114261087437365,-0.0374159898217041,
-0.0138174493639702));
#42718=CARTESIAN_POINT('Ctrl Pts',(0.00118169433289094,-0.0374197897866691,
-0.013789663595829));
#42719=CARTESIAN_POINT('Ctrl Pts',(0.0012041905540118,-0.0374219802457077,
-0.0137729476962217));
#42720=CARTESIAN_POINT('Ctrl Pts',(0.001315479341029,-0.0374328750306482,
-0.0136865650922548));
#42721=CARTESIAN_POINT('Ctrl Pts',(0.00139862431276907,-0.0374412141337442,
-0.0136099358648364));
#42722=CARTESIAN_POINT('Ctrl Pts',(0.00155539022228087,-0.0374584130200933,
-0.0134387761293495));
#42723=CARTESIAN_POINT('Ctrl Pts',(0.00162788127348689,-0.0374672472908509,
-0.0133438476403939));
#42724=CARTESIAN_POINT('Ctrl Pts',(0.00171388313790786,-0.0374796158601278,
-0.0132075347606267));
#42725=CARTESIAN_POINT('Ctrl Pts',(0.00173515687398948,-0.0374828707101665,
-0.0131713392086822));
#42726=CARTESIAN_POINT('Ctrl Pts',(0.00177189728981138,-0.0374888878380479,
-0.0131040680357225));
#42727=CARTESIAN_POINT('Ctrl Pts',(0.00178772426159953,-0.0374916363163615,
-0.013073207338985));
#42728=CARTESIAN_POINT('Ctrl Pts',(0.00182175300593214,-0.0374979275150254,
-0.0130023783042651));
#42729=CARTESIAN_POINT('Ctrl Pts',(0.00183945604787153,-0.0375014853212653,
-0.0129621919344909));
#42730=CARTESIAN_POINT('Ctrl Pts',(0.00190066855119462,-0.0375149470228309,
-0.0128098332313055));
#42731=CARTESIAN_POINT('Ctrl Pts',(0.00193534634612376,-0.0375251119061988,
-0.0126944064368557));
#42732=CARTESIAN_POINT('Ctrl Pts',(0.00197428570357736,-0.0375416613458246,
-0.0125040054806906));
#42733=CARTESIAN_POINT('Ctrl Pts',(0.00198508546783883,-0.0375479808965758,
-0.0124306560179852));
#42734=CARTESIAN_POINT('Ctrl Pts',(0.00199477796909831,-0.037556984851982,
-0.0123240083659955));
#42735=CARTESIAN_POINT('Ctrl Pts',(0.00199695119287043,-0.0375597399821034,
-0.0122910716876289));
#42736=CARTESIAN_POINT('Ctrl Pts',(0.00199942492100401,-0.0375647061858646,
-0.012230964590769));
#42737=CARTESIAN_POINT('Ctrl Pts',(0.0019999889362052,-0.0375669266170007,
-0.0122038128945948));
#42738=CARTESIAN_POINT('Ctrl Pts',(0.00200000784605045,-0.0375707300545887,
-0.0121567109876418));
#42739=CARTESIAN_POINT('Ctrl Pts',(0.00199971752824393,-0.0375723246956571,
-0.0121367673907308));
#42740=CARTESIAN_POINT('Ctrl Pts',(0.00199827865261496,-0.0375761848052306,
-0.012088033542739));
#42741=CARTESIAN_POINT('Ctrl Pts',(0.00199680636677368,-0.0375784340739312,
-0.0120592579837219));
#42742=CARTESIAN_POINT('Ctrl Pts',(0.00198863664519388,-0.0375871173561157,
-0.0119471261388361));
#42743=CARTESIAN_POINT('Ctrl Pts',(0.00197733578988694,-0.0375933658567144,
-0.0118641832568899));
#42744=CARTESIAN_POINT('Ctrl Pts',(0.00193199160779409,-0.0376104764635744,
-0.0116383236231266));
#42745=CARTESIAN_POINT('Ctrl Pts',(0.00188737037779793,-0.037621240369542,
-0.0114980939080775));
#42746=CARTESIAN_POINT('Ctrl Pts',(0.00181076746343494,-0.0376357217226709,
-0.011325626688677));
#42747=CARTESIAN_POINT('Ctrl Pts',(0.00179251476470957,-0.0376389783127346,
-0.011287791117484));
#42748=CARTESIAN_POINT('Ctrl Pts',(0.00175719588939473,-0.0376449710021385,
-0.0112201115652511));
#42749=CARTESIAN_POINT('Ctrl Pts',(0.00174052526988488,-0.0376476927582319,
-0.0111900789058641));
#42750=CARTESIAN_POINT('Ctrl Pts',(0.00170053544453039,-0.0376539978464694,
-0.0111222152772039));
#42751=CARTESIAN_POINT('Ctrl Pts',(0.00167671293918052,-0.0376575978266976,
-0.011084703914326));
#42752=CARTESIAN_POINT('Ctrl Pts',(0.0015976780758644,-0.0376690892594782,
-0.0109689608135697));
#42753=CARTESIAN_POINT('Ctrl Pts',(0.00153809393351182,-0.0376771270225727,
-0.0108938911192655));
#42754=CARTESIAN_POINT('Ctrl Pts',(0.0013871396130019,-0.0376960811339597,
-0.0107294421765821));
#42755=CARTESIAN_POINT('Ctrl Pts',(0.00129211542301816,-0.0377070332348158,
-0.010643958141956));
#42756=CARTESIAN_POINT('Ctrl Pts',(0.00116628818021785,-0.0377199898750456,
-0.0105508571697274));
#42757=CARTESIAN_POINT('Ctrl Pts',(0.00114260872823566,-0.0377223667357724,
-0.0105341206508794));
#42758=CARTESIAN_POINT('Ctrl Pts',(0.00110203233628788,-0.0377263271991535,
-0.0105067448989099));
#42759=CARTESIAN_POINT('Ctrl Pts',(0.00108532655081619,-0.0377279261293796,
-0.010495834097586));
#42760=CARTESIAN_POINT('Ctrl Pts',(0.00104563437170556,-0.0377316514175624,
-0.0104707498530013));
#42761=CARTESIAN_POINT('Ctrl Pts',(0.00102251944689131,-0.0377337653641723,
-0.0104567886714004));
#42762=CARTESIAN_POINT('Ctrl Pts',(0.000913135513759129,-0.0377435476955092,
-0.010393709286691));
#42763=CARTESIAN_POINT('Ctrl Pts',(0.000823559401920711,-0.0377509308597381,
-0.0103505837734056));
#42764=CARTESIAN_POINT('Ctrl Pts',(0.000609913314534462,-0.0377679524822781,
-0.0102666731944105));
#42765=CARTESIAN_POINT('Ctrl Pts',(0.000484338160591787,-0.0377775499413346,
-0.0102310203974994));
#42766=CARTESIAN_POINT('Ctrl Pts',(0.00031318480157617,-0.0377908652199709,
-0.010200043121726));
#42767=CARTESIAN_POINT('Ctrl Pts',(0.000269933614756223,-0.0377942468263184,
-0.0101936711953994));
#42768=CARTESIAN_POINT('Ctrl Pts',(0.000192081988798559,-0.0378003870508134,
-0.0101847969620219));
#42769=CARTESIAN_POINT('Ctrl Pts',(0.000157558763748098,-0.0378031284829236,
-0.0101817681027072));
#42770=CARTESIAN_POINT('Ctrl Pts',(8.02601991222002E-5,-0.0378093178668174,
-0.0101770061458459));
#42771=CARTESIAN_POINT('Ctrl Pts',(3.74741157882117E-5,-0.037812778840363,
-0.0101757466079817));
#42772=CARTESIAN_POINT('Ctrl Pts',(-0.000119439652899614,-0.0378256156577653,
-0.010176163712007));
#42773=CARTESIAN_POINT('Ctrl Pts',(-0.000233309468688445,-0.0378352265053964,
-0.010186234454147));
#42774=CARTESIAN_POINT('Ctrl Pts',(-0.000460272407019546,-0.037854832108227,
-0.0102260623594481));
#42775=CARTESIAN_POINT('Ctrl Pts',(-0.000572898115018368,-0.0378647928096336,
-0.0102561326654076));
#42776=CARTESIAN_POINT('Ctrl Pts',(-0.000708305517464874,-0.0378766942117564,
-0.0103052731690095));
#42777=CARTESIAN_POINT('Ctrl Pts',(-0.000734136555291568,-0.0378789602662475,
-0.0103152591807939));
#42778=CARTESIAN_POINT('Ctrl Pts',(-0.000778190739800792,-0.0378828082752215,
-0.0103333505260722));
#42779=CARTESIAN_POINT('Ctrl Pts',(-0.000796513180758882,-0.0378844029495056,
-0.0103411968884309));
#42780=CARTESIAN_POINT('Ctrl Pts',(-0.000840483662182668,-0.0378882173428055,
-0.0103608097132594));
#42781=CARTESIAN_POINT('Ctrl Pts',(-0.00086600533456494,-0.0378904221027663,
-0.010372847197548));
#42782=CARTESIAN_POINT('Ctrl Pts',(-0.000922462327936118,-0.0378952976082513,
-0.0104009511326673));
#42783=CARTESIAN_POINT('Ctrl Pts',(-0.000953249933725808,-0.0378979552284288,
-0.0104172944203574));
#42784=CARTESIAN_POINT('Ctrl Pts',(-0.00105570219694375,-0.0379068484286634,
-0.0104751620232309));
#42785=CARTESIAN_POINT('Ctrl Pts',(-0.00112521300116565,-0.0379129685014775,
-0.0105203306333061));
#42786=CARTESIAN_POINT('Ctrl Pts',(-0.00127779940184788,-0.0379270488797308,
-0.0106335447107695));
#42787=CARTESIAN_POINT('Ctrl Pts',(-0.00135859092995394,-0.0379350038016011,
-0.0107042166929915));
#42788=CARTESIAN_POINT('Ctrl Pts',(-0.00146399011277126,-0.0379465622199433,
-0.0108125242863669));
#42789=CARTESIAN_POINT('Ctrl Pts',(-0.001493603242113,-0.0379499603303875,
-0.0108450333008675));
#42790=CARTESIAN_POINT('Ctrl Pts',(-0.00154461631564727,-0.0379561171799667,
-0.0109048838850407));
#42791=CARTESIAN_POINT('Ctrl Pts',(-0.00156642154377424,-0.0379588583090676,
-0.010931857291425));
#42792=CARTESIAN_POINT('Ctrl Pts',(-0.00161301394457054,-0.0379649747119398,
-0.0109926610896534));
#42793=CARTESIAN_POINT('Ctrl Pts',(-0.00163745984551324,-0.0379683613307496,
-0.0110267307994885));
#42794=CARTESIAN_POINT('Ctrl Pts',(-0.00172650473410387,-0.0379814189809069,
-0.0111594468537029));
#42795=CARTESIAN_POINT('Ctrl Pts',(-0.00178339720749385,-0.0379913478302212,
-0.011262953321342));
#42796=CARTESIAN_POINT('Ctrl Pts',(-0.00187701245352657,-0.0380111392656663,
-0.0114758642272042));
#42797=CARTESIAN_POINT('Ctrl Pts',(-0.00191406948471588,-0.0380209576811575,
-0.0115846658969556));
#42798=CARTESIAN_POINT('Ctrl Pts',(-0.00194827554810133,-0.0380327409405725,
-0.0117230863763989));
#42799=CARTESIAN_POINT('Ctrl Pts',(-0.00195439133817699,-0.0380350204854707,
-0.0117502593335966));
#42800=CARTESIAN_POINT('Ctrl Pts',(-0.00196390691663225,-0.0380388818505571,
-0.0117970831734445));
#42801=CARTESIAN_POINT('Ctrl Pts',(-0.00196758365527947,-0.0380404767110245,
-0.0118166711122663));
#42802=CARTESIAN_POINT('Ctrl Pts',(-0.00197572896531307,-0.0380442785245321,
-0.0118639531783277));
#42803=CARTESIAN_POINT('Ctrl Pts',(-0.0019799088898604,-0.0380464708642459,
-0.0118916919884722));
#42804=CARTESIAN_POINT('Ctrl Pts',(-0.00199605023909678,-0.0380562095646285,
-0.0120165894677957));
#42805=CARTESIAN_POINT('Ctrl Pts',(-0.00200145408979447,-0.0380634870219811,
-0.0121144701986351));
#42806=CARTESIAN_POINT('Ctrl Pts',(-0.00199731153593474,-0.0380803134791257,
-0.0123413561098355));
#42807=CARTESIAN_POINT('Ctrl Pts',(-0.00198248144568392,-0.0380898236921549,
-0.0124698047553217));
#42808=CARTESIAN_POINT('Ctrl Pts',(-0.00194618537572517,-0.0381030510275557,
-0.0126387593561005));
#42809=CARTESIAN_POINT('Ctrl Pts',(-0.00193557881838683,-0.0381064401727976,
-0.0126812775162492));
#42810=CARTESIAN_POINT('Ctrl Pts',(-0.00191409822173182,-0.0381125879388726,
-0.0127567395422326));
#42811=CARTESIAN_POINT('Ctrl Pts',(-0.00190374692082494,-0.0381153291720509,
-0.0127898143704626));
#42812=CARTESIAN_POINT('Ctrl Pts',(-0.00187873404632049,-0.0381215103173969,
-0.0128630080940655));
#42813=CARTESIAN_POINT('Ctrl Pts',(-0.00186363639818402,-0.0381249630681109,
-0.0129029586219866));
#42814=CARTESIAN_POINT('Ctrl Pts',(-0.00180216363623665,-0.0381380824302724,
-0.0130511010363636));
#42815=CARTESIAN_POINT('Ctrl Pts',(-0.00174755377819325,-0.0381480026027225,
-0.0131555979925288));
#42816=CARTESIAN_POINT('Ctrl Pts',(-0.00162358878327254,-0.0381675624529433,
-0.0133491130223898));
#42817=CARTESIAN_POINT('Ctrl Pts',(-0.00155524949633392,-0.0381771562219628,
-0.0134383040426665));
#42818=CARTESIAN_POINT('Ctrl Pts',(-0.00146089134015479,-0.0381887517609584,
-0.0135420836852323));
#42819=CARTESIAN_POINT('Ctrl Pts',(-0.00144155781384415,-0.0381910518695265,
-0.0135624679820263));
#42820=CARTESIAN_POINT('Ctrl Pts',(-0.00140778240823205,-0.0381949339587745,
-0.0135966086989769));
#42821=CARTESIAN_POINT('Ctrl Pts',(-0.00139355415013042,-0.0381965294619312,
-0.0136105672596134));
#42822=CARTESIAN_POINT('Ctrl Pts',(-0.00135897495918084,-0.0382003139014703,
-0.0136434910454913));
#42823=CARTESIAN_POINT('Ctrl Pts',(-0.00133843302066023,-0.0382024887189372,
-0.0136622485263724));
#42824=CARTESIAN_POINT('Ctrl Pts',(-0.00129181546836941,-0.0382072821999684,
-0.0137030660070713));
#42825=CARTESIAN_POINT('Ctrl Pts',(-0.00126555243225979,-0.0382098884490764,
-0.0137248992007725));
#42826=CARTESIAN_POINT('Ctrl Pts',(-0.00117642234843681,-0.0382184761592371,
-0.0137952146576192));
#42827=CARTESIAN_POINT('Ctrl Pts',(-0.00111122759664908,-0.038224350204512,
-0.0138406282217031));
#42828=CARTESIAN_POINT('Ctrl Pts',(-0.000948034191794875,-0.0382385254756857,
-0.0139404366672938));
#42829=CARTESIAN_POINT('Ctrl Pts',(-0.000847843732767766,-0.0382468178552304,
-0.0139907033234199));
#42830=CARTESIAN_POINT('Ctrl Pts',(-0.000703072476874712,-0.0382587446283123,
-0.0140487204686366));
#42831=CARTESIAN_POINT('Ctrl Pts',(-0.000661635084892373,-0.0382621505658226,
-0.0140637571153293));
#42832=CARTESIAN_POINT('Ctrl Pts',(-0.00058675622901919,-0.0382683157921436,
-0.0140881609082087));
#42833=CARTESIAN_POINT('Ctrl Pts',(-0.000553502921073503,-0.0382710572738542,
-0.0140980493054214));
#42834=CARTESIAN_POINT('Ctrl Pts',(-0.000479603364999026,-0.0382771674742592,
-0.014117947979369));
#42835=CARTESIAN_POINT('Ctrl Pts',(-0.000438867166580089,-0.0382805473791945,
-0.0141275567149277));
#42836=CARTESIAN_POINT('Ctrl Pts',(-0.00028081590054678,-0.0382937222060191,
-0.0141596392710825));
#42837=CARTESIAN_POINT('Ctrl Pts',(-0.000161895817778599,-0.03830378332686,
-0.0141728623356128));
#42838=CARTESIAN_POINT('Ctrl Pts',(7.05325538605727E-5,-0.0383235685854632,
-0.0141778056755301));
#42839=CARTESIAN_POINT('Ctrl Pts',(0.000183600635649123,-0.0383332437427695,
-0.0141706171883384));
#42840=CARTESIAN_POINT('Ctrl Pts',(0.000323159407938675,-0.038344907592274,
-0.0141497712793331));
#42841=CARTESIAN_POINT('Ctrl Pts',(0.000350768658249815,-0.0383472004703621,
-0.0141450525720751));
#42842=CARTESIAN_POINT('Ctrl Pts',(0.000397840836073238,-0.0383510751404662,
-0.0141359858915574));
#42843=CARTESIAN_POINT('Ctrl Pts',(0.000417352300280133,-0.0383526702886812,
-0.0141319244302668));
#42844=CARTESIAN_POINT('Ctrl Pts',(0.000464017986272079,-0.0383564602177103,
-0.0141214804571578));
#42845=CARTESIAN_POINT('Ctrl Pts',(0.000491105055873706,-0.0383586407149533,
-0.0141148204943532));
#42846=CARTESIAN_POINT('Ctrl Pts',(0.000551156226446959,-0.0383634498457881,
-0.0140987162431857));
#42847=CARTESIAN_POINT('Ctrl Pts',(0.000584034979678977,-0.0383660659261672,
-0.0140889864722992));
#42848=CARTESIAN_POINT('Ctrl Pts',(0.000692782076354716,-0.0383747117753444,
-0.0140537398831911));
#42849=CARTESIAN_POINT('Ctrl Pts',(0.000767369744519523,-0.0383806325754964,
-0.0140245150544803));
#42850=CARTESIAN_POINT('Ctrl Pts',(0.000940729463619783,-0.0383947875991112,
-0.0139442835154794));
#42851=CARTESIAN_POINT('Ctrl Pts',(0.00103738482507462,-0.0384030139209357,
-0.0138893720281325));
#42852=CARTESIAN_POINT('Ctrl Pts',(0.00116535119373253,-0.0384148691110817,
-0.0138018600371267));
#42853=CARTESIAN_POINT('Ctrl Pts',(0.00120088617449846,-0.03841827413626,
-0.0137757949156857));
#42854=CARTESIAN_POINT('Ctrl Pts',(0.00126280191070961,-0.0384244379026909,
-0.013727154089493));
#42855=CARTESIAN_POINT('Ctrl Pts',(0.00128951092926202,-0.038427178847001,
-0.013705024341986));
#42856=CARTESIAN_POINT('Ctrl Pts',(0.00134714257232176,-0.0384332879193722,
-0.0136546898122304));
#42857=CARTESIAN_POINT('Ctrl Pts',(0.00137778161647662,-0.0384366672335894,
-0.0136261869984806));
#42858=CARTESIAN_POINT('Ctrl Pts',(0.00144068024534243,-0.0384438997234916,
-0.0135638811471868));
#42859=CARTESIAN_POINT('Ctrl Pts',(0.00147269431986616,-0.0384477601675629,
-0.0135298664699847));
#42860=CARTESIAN_POINT('Ctrl Pts',(0.00156554601470379,-0.0384595163259991,
-0.0134240206792137));
#42861=CARTESIAN_POINT('Ctrl Pts',(0.0016225300483719,-0.0384675211216179,
-0.0133489899076143));
#42862=CARTESIAN_POINT('Ctrl Pts',(0.00172320968516587,-0.0384831932744022,
-0.0131949856253024));
#42863=CARTESIAN_POINT('Ctrl Pts',(0.00176727787477499,-0.0384908413644903,
-0.0131164988831206));
#42864=CARTESIAN_POINT('Ctrl Pts',(0.00181829914083528,-0.0385006670117318,
-0.0130092909552669));
#42865=CARTESIAN_POINT('Ctrl Pts',(0.00183011762917312,-0.0385030286043635,
-0.0129830086783471));
#42866=CARTESIAN_POINT('Ctrl Pts',(0.00184914858536509,-0.0385069730492785,
-0.0129381178088366));
#42867=CARTESIAN_POINT('Ctrl Pts',(0.00185665728260757,-0.038508570877622,
-0.0129196419273955));
#42868=CARTESIAN_POINT('Ctrl Pts',(0.00187373007036264,-0.0385123058288285,
-0.0128757619656744));
#42869=CARTESIAN_POINT('Ctrl Pts',(0.00188305564672636,-0.0385144302377396,
-0.0128502702064181));
#42870=CARTESIAN_POINT('Ctrl Pts',(0.00190255726831701,-0.0385190867654835,
-0.012793399565067));
#42871=CARTESIAN_POINT('Ctrl Pts',(0.00191248194411514,-0.0385216076079525,
-0.0127619425805678));
#42872=CARTESIAN_POINT('Ctrl Pts',(0.00194213069085138,-0.0385297100461789,
-0.0126591759170012));
#42873=CARTESIAN_POINT('Ctrl Pts',(0.00195867880380338,-0.0385351965342661,
-0.0125870115839811));
#42874=CARTESIAN_POINT('Ctrl Pts',(0.00199157150403463,-0.0385496109676425,
-0.0123953192453778));
#42875=CARTESIAN_POINT('Ctrl Pts',(0.00200117372027142,-0.0385585161049327,
-0.0122749595176973));
#42876=CARTESIAN_POINT('Ctrl Pts',(0.00199941647148352,-0.0385710900101807,
-0.0121105772634695));
#42877=CARTESIAN_POINT('Ctrl Pts',(0.0019975020771425,-0.0385744832550496,
-0.0120667106936694));
#42878=CARTESIAN_POINT('Ctrl Pts',(0.00199149496027503,-0.0385806350369663,
-0.0119883689046225));
#42879=CARTESIAN_POINT('Ctrl Pts',(0.00198794502271778,-0.0385833760892058,
-0.011953869360343));
#42880=CARTESIAN_POINT('Ctrl Pts',(0.00197811920335749,-0.0385894968676683,
-0.0118778488280213));
#42881=CARTESIAN_POINT('Ctrl Pts',(0.00197142908283395,-0.0385928880427132,
-0.0118363991877451));
#42882=CARTESIAN_POINT('Ctrl Pts',(0.0019407326261264,-0.0386060660318903,
-0.0116780670179382));
#42883=CARTESIAN_POINT('Ctrl Pts',(0.00190759372731417,-0.0386161178177868,
-0.011563226552101));
#42884=CARTESIAN_POINT('Ctrl Pts',(0.00182363663131297,-0.0386358613029376,
-0.0113469658975532));
#42885=CARTESIAN_POINT('Ctrl Pts',(0.00177403136633091,-0.0386455040279907,
-0.011245519170315));
#42886=CARTESIAN_POINT('Ctrl Pts',(0.00170174007060536,-0.038657140703491,
-0.0111247267953279));
#42887=CARTESIAN_POINT('Ctrl Pts',(0.00168683581550337,-0.0386594364849881,
-0.0111009712775625));
#42888=CARTESIAN_POINT('Ctrl Pts',(0.00166048637217388,-0.0386633148367904,
-0.0110608723201784));
#42889=CARTESIAN_POINT('Ctrl Pts',(0.00164928853731533,-0.0386649108110946,
-0.0110443741793974));
#42890=CARTESIAN_POINT('Ctrl Pts',(0.00162183762097585,-0.0386687017917325,
-0.011005203628449));
#42891=CARTESIAN_POINT('Ctrl Pts',(0.00160535380731262,-0.0386708825337648,
-0.0109826989485342));
#42892=CARTESIAN_POINT('Ctrl Pts',(0.00152853376919155,-0.0386806617268341,
-0.0108822954586132));
#42893=CARTESIAN_POINT('Ctrl Pts',(0.00146295583648381,-0.0386879864424875,
-0.0108085667429993));
#42894=CARTESIAN_POINT('Ctrl Pts',(0.00129992593189615,-0.0387048253973154,
-0.0106504969271482));
#42895=CARTESIAN_POINT('Ctrl Pts',(0.00119925030815946,-0.0387143018343294,
-0.0105701404332164));
#42896=CARTESIAN_POINT('Ctrl Pts',(0.00105482590507667,-0.0387274947805248,
-0.0104760694790257));
#42897=CARTESIAN_POINT('Ctrl Pts',(0.00101730987124912,-0.0387308866944521,
-0.0104533542950851));
#42898=CARTESIAN_POINT('Ctrl Pts',(0.000948848476877909,-0.0387370386136422,
-0.0104149192761649));
#42899=CARTESIAN_POINT('Ctrl Pts',(0.000918182503645546,-0.0387397811943162,
-0.0103987369095612));
#42900=CARTESIAN_POINT('Ctrl Pts',(0.000848831002929154,-0.0387459647772771,
-0.0103644145171097));
#42901=CARTESIAN_POINT('Ctrl Pts',(0.000809954729837285,-0.038749418609445,
-0.0103467012235863));
#42902=CARTESIAN_POINT('Ctrl Pts',(0.000656348837988446,-0.0387630341016132,
-0.0102825704688347));
#42903=CARTESIAN_POINT('Ctrl Pts',(0.000537993840605165,-0.0387734815002861,
-0.0102456028975493));
#42904=CARTESIAN_POINT('Ctrl Pts',(0.000314162457675591,-0.038792969085903,
-0.0101978848996542));
#42905=CARTESIAN_POINT('Ctrl Pts',(0.000209744086835203,-0.0388019493781763,
-0.0101841032912974));
#42906=CARTESIAN_POINT('Ctrl Pts',(7.62098950558415E-5,-0.0388130110308991,
-0.0101771019148088));
#42907=CARTESIAN_POINT('Ctrl Pts',(4.76700322510099E-5,-0.0388153501473621,
-0.0101762176181587));
#42908=CARTESIAN_POINT('Ctrl Pts',(-8.0978828752807E-7,-0.0388192710984081,
-0.0101757541551425));
#42909=CARTESIAN_POINT('Ctrl Pts',(-2.07402249733232E-5,-0.0388208673944913,
-0.010175861500156));
#42910=CARTESIAN_POINT('Ctrl Pts',(-6.80134958519161E-5,-0.0388246169837417,
-0.0101768229667554));
#42911=CARTESIAN_POINT('Ctrl Pts',(-9.53461652196843E-5,-0.0388267571028226,
-0.0101779400294083));
#42912=CARTESIAN_POINT('Ctrl Pts',(-0.00021910429435872,-0.0388363563210289,
-0.0101855437635411));
#42913=CARTESIAN_POINT('Ctrl Pts',(-0.000315015879592685,-0.0388435486839813,
-0.010198453860677));
#42914=CARTESIAN_POINT('Ctrl Pts',(-0.000539503968791133,-0.0388605581307301,
-0.0102454280303853));
#42915=CARTESIAN_POINT('Ctrl Pts',(-0.000666339487880301,-0.0388703281950098,
-0.0102854582655062));
#42916=CARTESIAN_POINT('Ctrl Pts',(-0.000828230377753176,-0.0388838160644624,
-0.0103548851839165));
#42917=CARTESIAN_POINT('Ctrl Pts',(-0.000867617073926069,-0.038887180490065,
-0.0103733188261862));
#42918=CARTESIAN_POINT('Ctrl Pts',(-0.000937227764646918,-0.0388933008146155,
-0.0104087079959825));
#42919=CARTESIAN_POINT('Ctrl Pts',(-0.000967671728618498,-0.0388960399147139,
-0.0104251935556203));
#42920=CARTESIAN_POINT('Ctrl Pts',(-0.00103487342660241,-0.0389022376515323,
-0.0104638721203979));
#42921=CARTESIAN_POINT('Ctrl Pts',(-0.00107137402146666,-0.0389057096215286,
-0.0104864748012229));
#42922=CARTESIAN_POINT('Ctrl Pts',(-0.00114756650722974,-0.0389131957874466,
-0.0105371189615908));
#42923=CARTESIAN_POINT('Ctrl Pts',(-0.00118702022961977,-0.0389172188178244,
-0.0105654678260557));
#42924=CARTESIAN_POINT('Ctrl Pts',(-0.00130710441675965,-0.0389299311215999,
-0.0106585643158108));
#42925=CARTESIAN_POINT('Ctrl Pts',(-0.00138376868745635,-0.0389387523314952,
-0.0107281417222787));
#42926=CARTESIAN_POINT('Ctrl Pts',(-0.00151106740732872,-0.0389545389278394,
-0.0108630621805033));
#42927=CARTESIAN_POINT('Ctrl Pts',(-0.0015637026512866,-0.0389614957662427,
-0.0109262205302713));
#42928=CARTESIAN_POINT('Ctrl Pts',(-0.00162747895202746,-0.038970375950535,
-0.0110131110317425));
#42929=CARTESIAN_POINT('Ctrl Pts',(-0.00164225117205757,-0.0389724687551532,
-0.0110340702234264));
#42930=CARTESIAN_POINT('Ctrl Pts',(-0.00166771936987987,-0.0389761347155219,
-0.011071722515502));
#42931=CARTESIAN_POINT('Ctrl Pts',(-0.0016785763962559,-0.0389777167945088,
-0.0110882991468602));
#42932=CARTESIAN_POINT('Ctrl Pts',(-0.00170521428469145,-0.0389816512994129,
-0.0111303197582263));
#42933=CARTESIAN_POINT('Ctrl Pts',(-0.00172067341628377,-0.038983984867415,
-0.0111559614363426));
#42934=CARTESIAN_POINT('Ctrl Pts',(-0.00175440504553163,-0.0389892178713042,
-0.0112148631019774));
#42935=CARTESIAN_POINT('Ctrl Pts',(-0.00177231872958831,-0.0389921008736996,
-0.0112483157364037));
#42936=CARTESIAN_POINT('Ctrl Pts',(-0.00183384494869554,-0.0390024734347505,
-0.0113715116800154));
#42937=CARTESIAN_POINT('Ctrl Pts',(-0.00187168042820106,-0.0390098052098159,
-0.011463977560093));
#42938=CARTESIAN_POINT('Ctrl Pts',(-0.00193185239169798,-0.039024293295583,
-0.0116495213394445));
#42939=CARTESIAN_POINT('Ctrl Pts',(-0.00195472805560331,-0.0390314244176959,
-0.0117421322785678));
#42940=CARTESIAN_POINT('Ctrl Pts',(-0.00197779129677471,-0.0390418652493989,
-0.0118758884714093));
#42941=CARTESIAN_POINT('Ctrl Pts',(-0.00198345468803974,-0.039045009713617,
-0.0119159602858768));
#42942=CARTESIAN_POINT('Ctrl Pts',(-0.0019917244849381,-0.0390509306214746,
-0.0119907943745484));
#42943=CARTESIAN_POINT('Ctrl Pts',(-0.00199464504219202,-0.0390536963278605,
-0.0120255067525328));
#42944=CARTESIAN_POINT('Ctrl Pts',(-0.00199937083401339,-0.039060255758042,
-0.012107146991131));
#42945=CARTESIAN_POINT('Ctrl Pts',(-0.00200043248984103,-0.0390640703900177,
-0.012154095191338));
#42946=CARTESIAN_POINT('Ctrl Pts',(-0.00199914063173659,-0.0390725095052458,
-0.0122566957420391));
#42947=CARTESIAN_POINT('Ctrl Pts',(-0.00199611627667757,-0.0390771493744292,
-0.0123122995149277));
#42948=CARTESIAN_POINT('Ctrl Pts',(-0.0019761031886314,-0.0390947112710543,
-0.0125199732177311));
#42949=CARTESIAN_POINT('Ctrl Pts',(-0.00194400827975716,-0.0391079186545807,
-0.0126700523661867));
#42950=CARTESIAN_POINT('Ctrl Pts',(-0.00188450618699411,-0.0391234094647331,
-0.0128464797337211));
#42951=CARTESIAN_POINT('Ctrl Pts',(-0.00187310730703759,-0.0391261459905812,
-0.0128776885765298));
#42952=CARTESIAN_POINT('Ctrl Pts',(-0.00185354202130938,-0.0391304824674267,
-0.0129273778656509));
#42953=CARTESIAN_POINT('Ctrl Pts',(-0.00184586449283688,-0.0391321063495913,
-0.0129460426449891));
#42954=CARTESIAN_POINT('Ctrl Pts',(-0.00182824197818174,-0.0391356649585445,
-0.0129871063988338));
#42955=CARTESIAN_POINT('Ctrl Pts',(-0.00181816558567162,-0.0391375924958856,
-0.0130094445599979));
#42956=CARTESIAN_POINT('Ctrl Pts',(-0.00178035220529878,-0.0391444751045524,
-0.0130893222113692));
#42957=CARTESIAN_POINT('Ctrl Pts',(-0.00175027099708755,-0.0391493157868255,
-0.0131457155108037));
#42958=CARTESIAN_POINT('Ctrl Pts',(-0.00163858331329163,-0.0391656487626147,
-0.0133329149747651));
#42959=CARTESIAN_POINT('Ctrl Pts',(-0.00154460123708137,-0.0391768630169473,
-0.0134556791309526));
#42960=CARTESIAN_POINT('Ctrl Pts',(-0.00140203440492122,-0.0391924390950184,
-0.01360305156302));
#42961=CARTESIAN_POINT('Ctrl Pts',(-0.00136522964147225,-0.0391963522425618,
-0.0136382973499277));
#42962=CARTESIAN_POINT('Ctrl Pts',(-0.00130069999596002,-0.0392030762145198,
-0.0136955331519979));
#42963=CARTESIAN_POINT('Ctrl Pts',(-0.00127366327754493,-0.0392058557164568,
-0.0137182633888239));
#42964=CARTESIAN_POINT('Ctrl Pts',(-0.00121565059777392,-0.039211753309896,
-0.0137644700040737));
#42965=CARTESIAN_POINT('Ctrl Pts',(-0.00118456401256669,-0.0392148761858583,
-0.0137877829167457));
#42966=CARTESIAN_POINT('Ctrl Pts',(-0.00108865866217099,-0.0392244125808423,
-0.0138554328099652));
#42967=CARTESIAN_POINT('Ctrl Pts',(-0.00102189614895441,-0.0392309245681077,
-0.0138968676099053));
#42968=CARTESIAN_POINT('Ctrl Pts',(-0.000821271249900922,-0.0392501283527807,
-0.0140055856613206));
#42969=CARTESIAN_POINT('Ctrl Pts',(-0.000682079727168703,-0.03926304420327,
-0.0140619000518252));
#42970=CARTESIAN_POINT('Ctrl Pts',(-0.000503581911005871,-0.039278502301198,
-0.0141117447326403));
#42971=CARTESIAN_POINT('Ctrl Pts',(-0.000468999049084978,-0.039281445824025,
-0.0141204125555864));
#42972=CARTESIAN_POINT('Ctrl Pts',(-0.000416004516991219,-0.0392858619195975,
-0.0141321987829423));
#42973=CARTESIAN_POINT('Ctrl Pts',(-0.000397751866308258,-0.0392873660366728,
-0.0141359912947632));
#42974=CARTESIAN_POINT('Ctrl Pts',(-0.000357560853455187,-0.0392906373508532,
-0.0141437575398385));
#42975=CARTESIAN_POINT('Ctrl Pts',(-0.000335603531156165,-0.0392923984221514,
-0.0141476208476875));
#42976=CARTESIAN_POINT('Ctrl Pts',(-0.000267570151130193,-0.0392977876116455,
-0.0141584215510888));
#42977=CARTESIAN_POINT('Ctrl Pts',(-0.000221309693191029,-0.0393013572144864,
-0.0141641172492253));
#42978=CARTESIAN_POINT('Ctrl Pts',(-9.88980477596605E-5,-0.0393106544945962,
-0.0141748625823675));
#42979=CARTESIAN_POINT('Ctrl Pts',(-2.25835548107882E-5,-0.0393163019321686,
-0.0141771804639402));
#42980=CARTESIAN_POINT('Ctrl Pts',(0.000170954832808541,-0.0393306361910164,
-0.0141719839168146));
#42981=CARTESIAN_POINT('Ctrl Pts',(0.000287712108264512,-0.0393393069220895,
-0.0141585234126676));
#42982=CARTESIAN_POINT('Ctrl Pts',(0.000445635672679678,-0.0393516298942125,
-0.0141260682093816));
#42983=CARTESIAN_POINT('Ctrl Pts',(0.000488355158622234,-0.0393550229659414,
-0.0141158115596219));
#42984=CARTESIAN_POINT('Ctrl Pts',(0.000563917641588812,-0.0393611558751002,
-0.0140950155808122));
#42985=CARTESIAN_POINT('Ctrl Pts',(0.000596891768233525,-0.0393638777338799,
-0.0140850172254602));
#42986=CARTESIAN_POINT('Ctrl Pts',(0.000668837126536266,-0.0393699272511997,
-0.0140611561073833));
#42987=CARTESIAN_POINT('Ctrl Pts',(0.000707668701079003,-0.0393732656475689,
-0.0140469263291254));
#42988=CARTESIAN_POINT('Ctrl Pts',(0.000858546179152205,-0.0393865441104755,
-0.0139862689568736));
#42989=CARTESIAN_POINT('Ctrl Pts',(0.000966697141236107,-0.0393967639454479,
-0.013930901308442));
#42990=CARTESIAN_POINT('Ctrl Pts',(0.0011637925083519,-0.0394166207138157,
-0.0138062298084821));
#42991=CARTESIAN_POINT('Ctrl Pts',(0.00125324523339048,-0.0394262037351952,
-0.0137385179806201));
#42992=CARTESIAN_POINT('Ctrl Pts',(0.0013574102062589,-0.0394377832544203,
-0.0136449423714233));
#42993=CARTESIAN_POINT('Ctrl Pts',(0.00137786138051014,-0.0394400785240584,
-0.0136257786146584));
#42994=CARTESIAN_POINT('Ctrl Pts',(0.00141211123224659,-0.0394439509147715,
-0.0135923053619283));
#42995=CARTESIAN_POINT('Ctrl Pts',(0.00142611010389813,-0.0394455415596819,
-0.0135782101187051));
#42996=CARTESIAN_POINT('Ctrl Pts',(0.00145907054647678,-0.0394493070334893,
-0.0135440185682288));
#42997=CARTESIAN_POINT('Ctrl Pts',(0.00147782980878293,-0.0394514680107137,
-0.0135237339854722));
#42998=CARTESIAN_POINT('Ctrl Pts',(0.00151858969053321,-0.0394562217629058,
-0.0134777854478266));
#42999=CARTESIAN_POINT('Ctrl Pts',(0.0015403724221204,-0.0394588024886933,
-0.0134519391380417));
#43000=CARTESIAN_POINT('Ctrl Pts',(0.00160992706431918,-0.039467226826154,
-0.013365031001043));
#43001=CARTESIAN_POINT('Ctrl Pts',(0.00165480677781664,-0.0394729671599579,
-0.0133017417542357));
#43002=CARTESIAN_POINT('Ctrl Pts',(0.00175738242048589,-0.0394873042258206,
-0.0131376534881175));
#43003=CARTESIAN_POINT('Ctrl Pts',(0.00181018557107691,-0.0394958875859548,
-0.0130341521249923));
#43004=CARTESIAN_POINT('Ctrl Pts',(0.00187034280351365,-0.0395081420186117,
-0.012885626680233));
#43005=CARTESIAN_POINT('Ctrl Pts',(0.00188559610556518,-0.0395115639560029,
-0.0128440503054837));
#43006=CARTESIAN_POINT('Ctrl Pts',(0.00191036306444168,-0.039517757296807,
-0.0127689187199605));
#43007=CARTESIAN_POINT('Ctrl Pts',(0.00192040277636825,-0.0395205107533981,
-0.0127355554633069));
#43008=CARTESIAN_POINT('Ctrl Pts',(0.00194062379721181,-0.0395266485841883,
-0.0126613906611914));
#43009=CARTESIAN_POINT('Ctrl Pts',(0.00195039963330021,-0.0395300441949069,
-0.0126204969751554));
#43010=CARTESIAN_POINT('Ctrl Pts',(0.00198632348889163,-0.0395445915931025,
-0.0124460860663658));
#43011=CARTESIAN_POINT('Ctrl Pts',(0.00200009662524726,-0.03955610137136,
-0.0123104149942915));
#43012=CARTESIAN_POINT('Ctrl Pts',(0.00199999948980097,-0.0395676761865485,
-0.0121744247222927));
#43013=CARTESIAN_POINT('',(0.000482654256486283,-0.0397787742883183,-0.0102349656368742));
#43014=CARTESIAN_POINT('Ctrl Pts',(0.00199999947635761,-0.0395674495244771,
-0.0121744060238692));
#43015=CARTESIAN_POINT('Ctrl Pts',(0.00199970133985987,-0.0396002714048904,
-0.0117624056013177));
#43016=CARTESIAN_POINT('Ctrl Pts',(0.00186786604409727,-0.0396330932853036,
-0.0113509752358264));
#43017=CARTESIAN_POINT('Ctrl Pts',(0.00162916607223383,-0.0396659151657169,
-0.0110157593640319));
#43018=CARTESIAN_POINT('Ctrl Pts',(0.00161171964220948,-0.0396683140962045,
-0.0109912586479042));
#43019=CARTESIAN_POINT('Ctrl Pts',(0.00159372379493088,-0.0396707130266921,
-0.0109671563065562));
#43020=CARTESIAN_POINT('Ctrl Pts',(0.00157519789408884,-0.0396731119571797,
-0.0109434768852674));
#43021=CARTESIAN_POINT('Ctrl Pts',(0.00132172873142575,-0.0397059338375929,
-0.0106194978713678));
#43022=CARTESIAN_POINT('Ctrl Pts',(0.000964809959487887,-0.0397387557180061,
-0.0103761444985597));
#43023=CARTESIAN_POINT('Ctrl Pts',(0.000569808126240931,-0.0397715775984193,
-0.0102587412138639));
#43024=CARTESIAN_POINT('Ctrl Pts',(0.000540938099421197,-0.0397739764950523,
-0.0102501604031116));
#43025=CARTESIAN_POINT('Ctrl Pts',(0.000511876681535767,-0.0397763753916852,
-0.010242232583956));
#43026=CARTESIAN_POINT('Ctrl Pts',(0.000482654256486283,-0.0397787742883183,
-0.0102349656368742));
#43027=CARTESIAN_POINT('',(0.00171294960380956,-0.0397787743898723,-0.0132082309571848));
#43028=CARTESIAN_POINT('Origin',(0.,-0.0397787743898823,-0.0121758532865581));
#43029=CARTESIAN_POINT('',(0.00200022123764237,-0.0388647801189106,-0.0121764013269251));
#43030=CARTESIAN_POINT('Ctrl Pts',(0.00171294960381192,-0.0397787743898746,
-0.0132082309571895));
#43031=CARTESIAN_POINT('Ctrl Pts',(0.00150023895600091,-0.0397459829392836,
-0.0135611696787567));
#43032=CARTESIAN_POINT('Ctrl Pts',(0.00117410400373796,-0.0397157788326738,
-0.0138446217122324));
#43033=CARTESIAN_POINT('Ctrl Pts',(0.000797086095659716,-0.0396816687630686,
-0.0140093584080663));
#43034=CARTESIAN_POINT('Ctrl Pts',(0.000736412247895586,-0.039676179397375,
-0.0140358696399999));
#43035=CARTESIAN_POINT('Ctrl Pts',(0.000674460279395142,-0.0396706371456081,
-0.0140593805035415));
#43036=CARTESIAN_POINT('Ctrl Pts',(0.000611556020093166,-0.0396651474264523,
-0.0140798888792547));
#43037=CARTESIAN_POINT('Ctrl Pts',(0.000445016881923535,-0.039650613385242,
-0.0141341848403619));
#43038=CARTESIAN_POINT('Ctrl Pts',(0.000271030019870124,-0.0396363857556918,
-0.0141675943600055));
#43039=CARTESIAN_POINT('Ctrl Pts',(9.55329015372549E-5,-0.0396224105418801,
-0.0141760494170015));
#43040=CARTESIAN_POINT('Ctrl Pts',(-0.000134486275857888,-0.0396040936189845,
-0.014187131224347));
#43041=CARTESIAN_POINT('Ctrl Pts',(-0.000367011478658409,-0.0395862103113343,
-0.0141552106327799));
#43042=CARTESIAN_POINT('Ctrl Pts',(-0.000586810089275476,-0.0395686390442518,
-0.0140872852007923));
#43043=CARTESIAN_POINT('Ctrl Pts',(-0.000656254715950111,-0.0395630874619223,
-0.0140658243905858));
#43044=CARTESIAN_POINT('Ctrl Pts',(-0.000724490650272098,-0.0395574729195111,
-0.01404062219394));
#43045=CARTESIAN_POINT('Ctrl Pts',(-0.00079111974273048,-0.0395517690003329,
-0.01401186117842));
#43046=CARTESIAN_POINT('Ctrl Pts',(-0.00111283477109543,-0.039524227930021,
-0.013872990145026));
#43047=CARTESIAN_POINT('Ctrl Pts',(-0.00140093978232607,-0.0394943332468839,
-0.0136494145148475));
#43048=CARTESIAN_POINT('Ctrl Pts',(-0.00160907269804482,-0.0394657536876124,
-0.0133670741484452));
#43049=CARTESIAN_POINT('Ctrl Pts',(-0.00164226047277757,-0.0394611965421374,
-0.0133220536458219));
#43050=CARTESIAN_POINT('Ctrl Pts',(-0.00167343521716749,-0.0394566728347468,
-0.013275530438109));
#43051=CARTESIAN_POINT('Ctrl Pts',(-0.00170259000105306,-0.0394521974394702,
-0.0132277122546873));
#43052=CARTESIAN_POINT('Ctrl Pts',(-0.00173976013966668,-0.0394464916498667,
-0.0131667476969321));
#43053=CARTESIAN_POINT('Ctrl Pts',(-0.0017736876517133,-0.0394409546118393,
-0.0131038721225565));
#43054=CARTESIAN_POINT('Ctrl Pts',(-0.00180431702090932,-0.0394355645485264,
-0.0130394962385674));
#43055=CARTESIAN_POINT('Ctrl Pts',(-0.00197895506842673,-0.0394048322756237,
-0.0126724472596901));
#43056=CARTESIAN_POINT('Ctrl Pts',(-0.0020388440641331,-0.0393726943386263,
-0.0122505409511816));
#43057=CARTESIAN_POINT('Ctrl Pts',(-0.00197333802583864,-0.0393387239466838,
-0.0118491932184949));
#43058=CARTESIAN_POINT('Ctrl Pts',(-0.00196182927015393,-0.0393327556886184,
-0.0117786804364619));
#43059=CARTESIAN_POINT('Ctrl Pts',(-0.00194654553881331,-0.0393268034253514,
-0.011708817545723));
#43060=CARTESIAN_POINT('Ctrl Pts',(-0.00192778629130493,-0.039321097665926,
-0.0116399298725016));
#43061=CARTESIAN_POINT('Ctrl Pts',(-0.00191507534885312,-0.0393172315417828,
-0.0115932527736699));
#43062=CARTESIAN_POINT('Ctrl Pts',(-0.00190064394040254,-0.0393134035700773,
-0.0115470667176046));
#43063=CARTESIAN_POINT('Ctrl Pts',(-0.0018844539399446,-0.0393096042577624,
-0.0115015044103732));
#43064=CARTESIAN_POINT('Ctrl Pts',(-0.00176464438577769,-0.0392814885133697,
-0.0111643333441717));
#43065=CARTESIAN_POINT('Ctrl Pts',(-0.00154755482971262,-0.0392549422502329,
-0.0108606452113747));
#43066=CARTESIAN_POINT('Ctrl Pts',(-0.00127120349410412,-0.0392261183157976,
-0.010632760170493));
#43067=CARTESIAN_POINT('Ctrl Pts',(-0.00121609041974493,-0.0392203699243945,
-0.0105873127867277));
#43068=CARTESIAN_POINT('Ctrl Pts',(-0.00115860135483299,-0.0392145367366959,
-0.010544809906072));
#43069=CARTESIAN_POINT('Ctrl Pts',(-0.00109906668667438,-0.0392086411984728,
-0.0105054936416087));
#43070=CARTESIAN_POINT('Ctrl Pts',(-0.000912724758827148,-0.0391901883206427,
-0.0103824347795632));
#43071=CARTESIAN_POINT('Ctrl Pts',(-0.000705466934213524,-0.0391718322911769,
-0.0102884889069067));
#43072=CARTESIAN_POINT('Ctrl Pts',(-0.000488260829398752,-0.0391539022648083,
-0.0102339312550549));
#43073=CARTESIAN_POINT('Ctrl Pts',(-0.000310359136001515,-0.039139216756515,
-0.0101892460531335));
#43074=CARTESIAN_POINT('Ctrl Pts',(-0.000125860786950418,-0.0391248170262699,
-0.0101709505916726));
#43075=CARTESIAN_POINT('Ctrl Pts',(5.72982369894981E-5,-0.0391108839264696,
-0.0101767492571837));
#43076=CARTESIAN_POINT('Ctrl Pts',(0.000128621592728783,-0.0391054582837017,
-0.0101790072965321));
#43077=CARTESIAN_POINT('Ctrl Pts',(0.000199778699520524,-0.0391000352921531,
-0.0101850193738325));
#43078=CARTESIAN_POINT('Ctrl Pts',(0.000270361469596534,-0.039094544851949,
-0.0101947616994797));
#43079=CARTESIAN_POINT('Ctrl Pts',(0.000665306963198104,-0.0390638231246187,
-0.0102492748279304));
#43080=CARTESIAN_POINT('Ctrl Pts',(0.00104544158884886,-0.0390292888960902,
-0.0104228400803495));
#43081=CARTESIAN_POINT('Ctrl Pts',(0.00134169711478715,-0.0389972610858596,
-0.0106906329936509));
#43082=CARTESIAN_POINT('Ctrl Pts',(0.00134641586989222,-0.0389967509472131,
-0.0106948983965417));
#43083=CARTESIAN_POINT('Ctrl Pts',(0.00135111369317754,-0.0389962414444471,
-0.0106991880265136));
#43084=CARTESIAN_POINT('Ctrl Pts',(0.00135579052697412,-0.038995732603096,
-0.0107035016074603));
#43085=CARTESIAN_POINT('Ctrl Pts',(0.00140924983375533,-0.0389899162095538,
-0.0107528086936603));
#43086=CARTESIAN_POINT('Ctrl Pts',(0.0014597357188015,-0.0389841037191059,
-0.0108052585006679));
#43087=CARTESIAN_POINT('Ctrl Pts',(0.00150735437408238,-0.0389785280511923,
-0.0108600840695627));
#43088=CARTESIAN_POINT('Ctrl Pts',(0.00177724857175393,-0.0389469261420425,
-0.011170825791299));
#43089=CARTESIAN_POINT('Ctrl Pts',(0.00194813388996565,-0.0389156432761473,
-0.0115672436940755));
#43090=CARTESIAN_POINT('Ctrl Pts',(0.00199002028125891,-0.0388811955851008,
-0.0119772040445301));
#43091=CARTESIAN_POINT('Ctrl Pts',(0.0019967610977407,-0.0388756518856701,
-0.0120431793506355));
#43092=CARTESIAN_POINT('Ctrl Pts',(0.00200023005550795,-0.0388700852750759,
-0.0121094851408837));
#43093=CARTESIAN_POINT('Ctrl Pts',(0.00200038122575368,-0.0388645498389405,
-0.0121757929019176));
#43094=CARTESIAN_POINT('',(0.0019999997328271,-0.0378650183082204,-0.0121752053157853));
#43095=CARTESIAN_POINT('Ctrl Pts',(0.00199999951611709,-0.0388650992552875,
-0.0121772445203322));
#43096=CARTESIAN_POINT('Ctrl Pts',(0.00199971375497249,-0.0388324006779061,
-0.0125880469041955));
#43097=CARTESIAN_POINT('Ctrl Pts',(0.0018685951062426,-0.0387997021005247,
-0.0129985667414531));
#43098=CARTESIAN_POINT('Ctrl Pts',(0.00163102667195928,-0.0387670035231434,
-0.0133333298501901));
#43099=CARTESIAN_POINT('Ctrl Pts',(0.00156586986390711,-0.0387580354338581,
-0.013425143797126));
#43100=CARTESIAN_POINT('Ctrl Pts',(0.00149299350802138,-0.0387490673445728,
-0.0135113667208478));
#43101=CARTESIAN_POINT('Ctrl Pts',(0.00141349983230828,-0.0387400992552875,
-0.01359078021897));
#43102=CARTESIAN_POINT('Ctrl Pts',(0.00112899622298658,-0.0387080029438829,
-0.0138749968769863));
#43103=CARTESIAN_POINT('Ctrl Pts',(0.000754664908831541,-0.0386759066324783,
-0.0140714186061737));
#43104=CARTESIAN_POINT('Ctrl Pts',(0.000357828226795811,-0.0386438103210738,
-0.0141435826785498));
#43105=CARTESIAN_POINT('Ctrl Pts',(0.000239500984134324,-0.0386342399658117,
-0.0141651002853892));
#43106=CARTESIAN_POINT('Ctrl Pts',(0.000119335163155483,-0.0386246696105496,
-0.0141758907958467));
#43107=CARTESIAN_POINT('Ctrl Pts',(-6.26990510425628E-7,-0.0386150992552875,
-0.0141758531882788));
#43108=CARTESIAN_POINT('Ctrl Pts',(-0.000404434472395409,-0.0385828842529636,
-0.014175726596543));
#43109=CARTESIAN_POINT('Ctrl Pts',(-0.000809412778774544,-0.0385506692506397,
-0.0140490048166835));
#43110=CARTESIAN_POINT('Ctrl Pts',(-0.00114175084775083,-0.0385184542483158,
-0.0138179266715383));
#43111=CARTESIAN_POINT('Ctrl Pts',(-0.00123925659506402,-0.038509002583973,
-0.0137501299027253));
#43112=CARTESIAN_POINT('Ctrl Pts',(-0.00133062013334003,-0.0384995509196303,
-0.0136736807710986));
#43113=CARTESIAN_POINT('Ctrl Pts',(-0.0014143867001888,-0.0384900992552875,
-0.0135898936899162));
#43114=CARTESIAN_POINT('Ctrl Pts',(-0.001699842495272,-0.0384578903148794,
-0.0133043679870447));
#43115=CARTESIAN_POINT('Ctrl Pts',(-0.00189665011598153,-0.0384256813744713,
-0.0129285118578515));
#43116=CARTESIAN_POINT('Ctrl Pts',(-0.00196835538740126,-0.0383934724340632,
-0.0125302218360774));
#43117=CARTESIAN_POINT('Ctrl Pts',(-0.00198941068508536,-0.0383840147078046,
-0.0124132692772625));
#43118=CARTESIAN_POINT('Ctrl Pts',(-0.00199999185979339,-0.038374556981546,
-0.0122945381296574));
#43119=CARTESIAN_POINT('Ctrl Pts',(-0.00199999999529041,-0.0383650992552875,
-0.012175990539403));
#43120=CARTESIAN_POINT('Ctrl Pts',(-0.00200002770128779,-0.0383328903148794,
-0.0117722685278277));
#43121=CARTESIAN_POINT('Ctrl Pts',(-0.00187351208327366,-0.0383006813744713,
-0.0113673119004809));
#43122=CARTESIAN_POINT('Ctrl Pts',(-0.00164264075488384,-0.0382684724340632,
-0.0110349188667098));
#43123=CARTESIAN_POINT('Ctrl Pts',(-0.00157484846500414,-0.0382590147078046,
-0.010937316080532));
#43124=CARTESIAN_POINT('Ctrl Pts',(-0.00149838955109543,-0.0382495569815461,
-0.0108458593477331));
#43125=CARTESIAN_POINT('Ctrl Pts',(-0.00141458076793401,-0.0382400992552875,
-0.0107620070251169));
#43126=CARTESIAN_POINT('Ctrl Pts',(-0.00112911044763666,-0.0382078842529635,
-0.0104763884002906));
#43127=CARTESIAN_POINT('Ctrl Pts',(-0.000753248182734186,-0.0381756692506395,
-0.0102794205933449));
#43128=CARTESIAN_POINT('Ctrl Pts',(-0.00035490072884417,-0.0381434542483154,
-0.010207593783173));
#43129=CARTESIAN_POINT('Ctrl Pts',(-0.000238028273332784,-0.0381340025839728,
-0.0101865202816497));
#43130=CARTESIAN_POINT('Ctrl Pts',(-0.000119375880855756,-0.0381245509196302,
-0.01017590689184));
#43131=CARTESIAN_POINT('Ctrl Pts',(-9.01496180030455E-7,-0.0381150992552875,
-0.010175853489732));
#43132=CARTESIAN_POINT('Ctrl Pts',(0.000401418201829956,-0.0380830029438829,
-0.0101756721448781));
#43133=CARTESIAN_POINT('Ctrl Pts',(0.000805137298915929,-0.0380509066324782,
-0.0103011892691929));
#43134=CARTESIAN_POINT('Ctrl Pts',(0.00113689908351052,-0.0380188103210737,
-0.0105304170301468));
#43135=CARTESIAN_POINT('Ctrl Pts',(0.00123582254237512,-0.0380092399658116,
-0.0105987672863677));
#43136=CARTESIAN_POINT('Ctrl Pts',(0.00132846178825258,-0.0379996696105496,
-0.0106759973698235));
#43137=CARTESIAN_POINT('Ctrl Pts',(0.00141330561624802,-0.0379900992552875,
-0.010760732360601));
#43138=CARTESIAN_POINT('Ctrl Pts',(0.00170318748573643,-0.0379574006779062,
-0.0110502423711461));
#43139=CARTESIAN_POINT('Ctrl Pts',(0.00190167861782618,-0.037924702100525,
-0.0114324535509333));
#43140=CARTESIAN_POINT('Ctrl Pts',(0.00197119882455475,-0.0378920035231438,
-0.0118376592681693));
#43141=CARTESIAN_POINT('Ctrl Pts',(0.00199026581373331,-0.0378830354338584,
-0.0119487931872009));
#43142=CARTESIAN_POINT('Ctrl Pts',(0.00199990546780057,-0.0378740673445729,
-0.0120615186677999));
#43143=CARTESIAN_POINT('Ctrl Pts',(0.00199999930632796,-0.0378650992552875,
-0.0121741875471745));
#43144=CARTESIAN_POINT('',(0.00199999975724282,-0.0368651541991762,-0.0121765544739802));
#43145=CARTESIAN_POINT('Ctrl Pts',(0.00199999999997258,-0.0378649676055565,
-0.0121758428136169));
#43146=CARTESIAN_POINT('Ctrl Pts',(0.00200000215106864,-0.0378322885229654,
-0.0125866340168838));
#43147=CARTESIAN_POINT('Ctrl Pts',(0.00186917812243619,-0.0377996106305976,
-0.0129972356615072));
#43148=CARTESIAN_POINT('Ctrl Pts',(0.00163185633020602,-0.0377669292674898,
-0.0133321598711483));
#43149=CARTESIAN_POINT('Ctrl Pts',(0.0015666975511292,-0.0377579563126732,
-0.0134241162497783));
#43150=CARTESIAN_POINT('Ctrl Pts',(0.00149379912816242,-0.0377489830962234,
-0.0135104753770261));
#43151=CARTESIAN_POINT('Ctrl Pts',(0.00141426605178541,-0.037740009521673,
-0.0135900143575706));
#43152=CARTESIAN_POINT('Ctrl Pts',(0.00112991319882504,-0.0377079264985973,
-0.0138743883195708));
#43153=CARTESIAN_POINT('Ctrl Pts',(0.000755682143339694,-0.0376758388980586,
-0.0140710149774864));
#43154=CARTESIAN_POINT('Ctrl Pts',(0.000358876233171651,-0.0376437599461721,
-0.0141433918120423));
#43155=CARTESIAN_POINT('Ctrl Pts',(0.000240460523385157,-0.037634186873394,
-0.0141649906693587));
#43156=CARTESIAN_POINT('Ctrl Pts',(0.000120197207218872,-0.0376246145708288,
-0.0141758452605839));
#43157=CARTESIAN_POINT('Ctrl Pts',(1.33621037764426E-7,-0.037615043389977,
-0.0141758532820945));
#43158=CARTESIAN_POINT('Ctrl Pts',(-0.000403695574715009,-0.0375828510959709,
-0.0141758802621326));
#43159=CARTESIAN_POINT('Ctrl Pts',(-0.000808740639887077,-0.0375506714917629,
-0.0140492994009556));
#43160=CARTESIAN_POINT('Ctrl Pts',(-0.00114117588555066,-0.037518455536669,
-0.0138183262994985));
#43161=CARTESIAN_POINT('Ctrl Pts',(-0.00123877723638862,-0.0375089970909214,
-0.0137505137344847));
#43162=CARTESIAN_POINT('Ctrl Pts',(-0.00133023040427276,-0.0374995355117976,
-0.0136740338122211));
#43163=CARTESIAN_POINT('Ctrl Pts',(-0.00141407707748936,-0.037490069558209,
-0.0135902033206441));
#43164=CARTESIAN_POINT('Ctrl Pts',(-0.00169937545959153,-0.0374578605135292,
-0.0133049599985155));
#43165=CARTESIAN_POINT('Ctrl Pts',(-0.00189619771625313,-0.0374256008220651,
-0.0129294796373532));
#43166=CARTESIAN_POINT('Ctrl Pts',(-0.00196811542615174,-0.0373934727199154,
-0.0125315521329768));
#43167=CARTESIAN_POINT('Ctrl Pts',(-0.00198932393384032,-0.0373839981537422,
-0.0124142034500451));
#43168=CARTESIAN_POINT('Ctrl Pts',(-0.00199998497219453,-0.0373745350313396,
-0.0122950597653228));
#43169=CARTESIAN_POINT('Ctrl Pts',(-0.00199999998407383,-0.0373650880263686,
-0.0121761056844425));
#43170=CARTESIAN_POINT('Ctrl Pts',(-0.00200005102695467,-0.0373329666417254,
-0.0117716420688781));
#43171=CARTESIAN_POINT('Ctrl Pts',(-0.00187311158569394,-0.0373010315927791,
-0.0113660240936564));
#43172=CARTESIAN_POINT('Ctrl Pts',(-0.00164149534947217,-0.037269036273748,
-0.0110332715530873));
#43173=CARTESIAN_POINT('Ctrl Pts',(-0.00157400171920308,-0.0372597127467438,
-0.0109363065159611));
#43174=CARTESIAN_POINT('Ctrl Pts',(-0.00149794572979849,-0.037250384101868,
-0.0108454195059611));
#43175=CARTESIAN_POINT('Ctrl Pts',(-0.0014146164566859,-0.0372410442369463,
-0.0107620427333108));
#43176=CARTESIAN_POINT('Ctrl Pts',(-0.00112956846034967,-0.0372090949629093,
-0.0104768322532812));
#43177=CARTESIAN_POINT('Ctrl Pts',(-0.000754297942754812,-0.0371770143977276,
-0.0102799430662898));
#43178=CARTESIAN_POINT('Ctrl Pts',(-0.000356493832770366,-0.0371448730653759,
-0.0102078817046503));
#43179=CARTESIAN_POINT('Ctrl Pts',(-0.000238930692126867,-0.0371353743299911,
-0.0101865853937758));
#43180=CARTESIAN_POINT('Ctrl Pts',(-0.000119558078688254,-0.037125870287316,
-0.0101758755274922));
#43181=CARTESIAN_POINT('Ctrl Pts',(-3.72633079933872E-7,-0.0371163627576488,
-0.010175853321272));
#43182=CARTESIAN_POINT('Ctrl Pts',(0.000402000380372829,-0.0370842651022417,
-0.010175778352523));
#43183=CARTESIAN_POINT('Ctrl Pts',(0.000805732491409436,-0.0370521277036917,
-0.0103014342785915));
#43184=CARTESIAN_POINT('Ctrl Pts',(0.00113745747156368,-0.0370199314595979,
-0.0105308029832592));
#43185=CARTESIAN_POINT('Ctrl Pts',(0.00123647545702504,-0.0370103210671936,
-0.0105992682132624));
#43186=CARTESIAN_POINT('Ctrl Pts',(0.00132919144468881,-0.0370007054317224,
-0.0106766325077531));
#43187=CARTESIAN_POINT('Ctrl Pts',(0.00141408952576617,-0.0369910840451469,
-0.010761515698456));
#43188=CARTESIAN_POINT('Ctrl Pts',(0.00170382515047177,-0.0369582486922789,
-0.011051200506089));
#43189=CARTESIAN_POINT('Ctrl Pts',(0.0019021080795554,-0.0369253463572291,
-0.0114335426878814));
#43190=CARTESIAN_POINT('Ctrl Pts',(0.0019713954509908,-0.0368923837711043,
-0.0118388073315122));
#43191=CARTESIAN_POINT('Ctrl Pts',(0.00199042635448992,-0.0368833300607004,
-0.0119501198573703));
#43192=CARTESIAN_POINT('Ctrl Pts',(0.00200000049791846,-0.0368742718048616,
-0.0120630233263041));
#43193=CARTESIAN_POINT('Ctrl Pts',(0.00199999999998053,-0.036865209143065,
-0.0121758621122101));
#43194=CARTESIAN_POINT('',(0.00199999993113723,-0.0358650692048068,-0.0121754868239693));
#43195=CARTESIAN_POINT('Ctrl Pts',(0.0019999995145051,-0.0368650992552875,
-0.0121772468357502));
#43196=CARTESIAN_POINT('Ctrl Pts',(0.00199971327855225,-0.0368324031647462,
-0.0125880480977315));
#43197=CARTESIAN_POINT('Ctrl Pts',(0.00186859482625184,-0.036799707074205,
-0.0129985668623653));
#43198=CARTESIAN_POINT('Ctrl Pts',(0.0016310271184896,-0.0367670109836637,
-0.0133333292209738));
#43199=CARTESIAN_POINT('Ctrl Pts',(0.00156584748471249,-0.0367580404075383,
-0.0134251754072337));
#43200=CARTESIAN_POINT('Ctrl Pts',(0.00149294287498649,-0.0367490698314129,
-0.013511426630081));
#43201=CARTESIAN_POINT('Ctrl Pts',(0.00141341672260997,-0.0367400992552875,
-0.0135908632399671));
#43202=CARTESIAN_POINT('Ctrl Pts',(0.00112889816887164,-0.036708005468915,
-0.0138750614399711));
#43203=CARTESIAN_POINT('Ctrl Pts',(0.000754557696843852,-0.0366759116825424,
-0.0140714608728529));
#43204=CARTESIAN_POINT('Ctrl Pts',(0.000357718917181035,-0.0366438178961698,
-0.0141436025531799));
#43205=CARTESIAN_POINT('Ctrl Pts',(0.000239350517464174,-0.0366342450158757,
-0.0141651208515188));
#43206=CARTESIAN_POINT('Ctrl Pts',(0.000119142893453722,-0.0366246721355816,
-0.01417590468007));
#43207=CARTESIAN_POINT('Ctrl Pts',(-8.59619391707486E-7,-0.0366150992552875,
-0.0141758531018217));
#43208=CARTESIAN_POINT('Ctrl Pts',(-0.00040466476463091,-0.0365828867771829,
-0.014175679542439));
#43209=CARTESIAN_POINT('Ctrl Pts',(-0.000809626539648802,-0.0365506742990785,
-0.014048912036177));
#43210=CARTESIAN_POINT('Ctrl Pts',(-0.0011419369127495,-0.0365184618209739,
-0.0138177972829539));
#43211=CARTESIAN_POINT('Ctrl Pts',(-0.00123946821469572,-0.0365090076324118,
-0.0137499663495692));
#43212=CARTESIAN_POINT('Ctrl Pts',(-0.00133085212103917,-0.0364995534438496,
-0.0136734778336607));
#43213=CARTESIAN_POINT('Ctrl Pts',(-0.00141463257027406,-0.0364900992552875,
-0.0135896477168484));
#43214=CARTESIAN_POINT('Ctrl Pts',(-0.00170003711586502,-0.036457892834635,
-0.0133040739748339));
#43215=CARTESIAN_POINT('Ctrl Pts',(-0.00189677909075885,-0.0364256864139827,
-0.0129281858052638));
#43216=CARTESIAN_POINT('Ctrl Pts',(-0.00196841594664184,-0.0363934799933302,
-0.012529885292182));
#43217=CARTESIAN_POINT('Ctrl Pts',(-0.0019894584054625,-0.036384019747316,
-0.0124128893402874));
#43218=CARTESIAN_POINT('Ctrl Pts',(-0.00200001928488183,-0.0363745595013017,
-0.0122941153820976));
#43219=CARTESIAN_POINT('Ctrl Pts',(-0.00199999997348158,-0.0363650992552875,
-0.0121755275970281));
#43220=CARTESIAN_POINT('Ctrl Pts',(-0.00199993422983402,-0.0363328928346353,
-0.0117718078539671));
#43221=CARTESIAN_POINT('Ctrl Pts',(-0.0018733262230654,-0.0363006864139831,
-0.0113668822653373));
#43222=CARTESIAN_POINT('Ctrl Pts',(-0.00164237995384072,-0.0362684799933309,
-0.0110345434744465));
#43223=CARTESIAN_POINT('Ctrl Pts',(-0.00157454228424741,-0.0362590197473164,
-0.0109369229795792));
#43224=CARTESIAN_POINT('Ctrl Pts',(-0.00149803348157776,-0.036249559501302,
-0.0108454547200247));
#43225=CARTESIAN_POINT('Ctrl Pts',(-0.00141417203720899,-0.0362400992552875,
-0.0107615982002402));
#43226=CARTESIAN_POINT('Ctrl Pts',(-0.00112862080139359,-0.0362078867771829,
-0.0104760637328111));
#43227=CARTESIAN_POINT('Ctrl Pts',(-0.000752703850683686,-0.0361756742990784,
-0.0102792048728464));
#43228=CARTESIAN_POINT('Ctrl Pts',(-0.000354337681183733,-0.0361434618209737,
-0.0102074923420936));
#43229=CARTESIAN_POINT('Ctrl Pts',(-0.000237419359315358,-0.0361340076324117,
-0.0101864451011517));
#43230=CARTESIAN_POINT('Ctrl Pts',(-0.000118722882568433,-0.0361245534438496,
-0.0101758656371648));
#43231=CARTESIAN_POINT('Ctrl Pts',(-2.08240354928347E-7,-0.0361150992552875,
-0.0101758532973991));
#43232=CARTESIAN_POINT('Ctrl Pts',(0.000402109058929343,-0.036083005468915,
-0.0101758114080503));
#43233=CARTESIAN_POINT('Ctrl Pts',(0.000805782738187552,-0.0360509116825423,
-0.0103014670235892));
#43234=CARTESIAN_POINT('Ctrl Pts',(0.0011374641750515,-0.0360188178961697,
-0.0105308076183548));
#43235=CARTESIAN_POINT('Ctrl Pts',(0.00123639755280903,-0.0360092450158756,
-0.0105992149428997));
#43236=CARTESIAN_POINT('Ctrl Pts',(0.00132903940203891,-0.0359996721355816,
-0.0106765059496287));
#43237=CARTESIAN_POINT('Ctrl Pts',(0.00141387750156739,-0.0359900992552875,
-0.0107613037432188));
#43238=CARTESIAN_POINT('Ctrl Pts',(0.00170364130288576,-0.0359574031647456,
-0.0110509298799503));
#43239=CARTESIAN_POINT('Ctrl Pts',(0.00190197781676828,-0.0359247070742038,
-0.0114332199240294));
#43240=CARTESIAN_POINT('Ctrl Pts',(0.00197133477400979,-0.035892010983662,
-0.0118384526215028));
#43241=CARTESIAN_POINT('Ctrl Pts',(0.00199036371154978,-0.0358830404075371,
-0.0119496332152899));
#43242=CARTESIAN_POINT('Ctrl Pts',(0.00199995803787705,-0.0358740698314123,
-0.012062402698519));
#43243=CARTESIAN_POINT('Ctrl Pts',(0.00199999986229583,-0.0358650992552875,
-0.0121751111163331));
#43244=CARTESIAN_POINT('',(0.00199999998396862,-0.0348650992552875,-0.0121756000563658));
#43245=CARTESIAN_POINT('Ctrl Pts',(0.00199999999997863,-0.0358650391543261,
-0.0121758625316054));
#43246=CARTESIAN_POINT('Ctrl Pts',(0.00199999810105016,-0.0358323500840859,
-0.0125866616126267));
#43247=CARTESIAN_POINT('Ctrl Pts',(0.00186916518615,-0.0357996610138456,
-0.0129972691594506));
#43248=CARTESIAN_POINT('Ctrl Pts',(0.00163183150648035,-0.0357669719436053,
-0.0133321949032346));
#43249=CARTESIAN_POINT('Ctrl Pts',(0.00156666930865016,-0.0357579968513856,
-0.0134241519217465));
#43250=CARTESIAN_POINT('Ctrl Pts',(0.00149376720214781,-0.035749021759166,
-0.0135105113347003));
#43251=CARTESIAN_POINT('Ctrl Pts',(0.00141423022479208,-0.0357400466669462,
-0.0135900501863159));
#43252=CARTESIAN_POINT('Ctrl Pts',(0.00112987870759773,-0.0357079599423248,
-0.0138744084041501));
#43253=CARTESIAN_POINT('Ctrl Pts',(0.000755656078176272,-0.0356758732177034,
-0.0140710224466294));
#43254=CARTESIAN_POINT('Ctrl Pts',(0.000358863204303028,-0.0356437864930819,
-0.0141433941884449));
#43255=CARTESIAN_POINT('Ctrl Pts',(0.000240426089604611,-0.0356342090552434,
-0.0141649961396156));
#43256=CARTESIAN_POINT('Ctrl Pts',(0.000120140973166075,-0.0356246316174049,
-0.0141758499009532));
#43257=CARTESIAN_POINT('Ctrl Pts',(5.63737627424982E-8,-0.0356150541795664,
-0.0141758532857636));
#43258=CARTESIAN_POINT('Ctrl Pts',(-0.000403744092267254,-0.0355828487686996,
-0.0141758646676394));
#43259=CARTESIAN_POINT('Ctrl Pts',(-0.000808760244496433,-0.0355506433578327,
-0.0140492854455321));
#43260=CARTESIAN_POINT('Ctrl Pts',(-0.00114117477149515,-0.0355184379469659,
-0.013818327073534));
#43261=CARTESIAN_POINT('Ctrl Pts',(-0.00123880514950277,-0.0355089791953728,
-0.0137504944388842));
#43262=CARTESIAN_POINT('Ctrl Pts',(-0.00133028359890378,-0.0354995204437797,
-0.0136739893304062));
#43263=CARTESIAN_POINT('Ctrl Pts',(-0.00141415049894442,-0.0354900616921866,
-0.0135901299095478));
#43264=CARTESIAN_POINT('Ctrl Pts',(-0.00169964914213271,-0.0354578623293297,
-0.0133046567268976));
#43265=CARTESIAN_POINT('Ctrl Pts',(-0.00189651867363536,-0.035425662966473,
-0.012928840079799));
#43266=CARTESIAN_POINT('Ctrl Pts',(-0.0019682930311079,-0.0353934636036161,
-0.0125305680222149));
#43267=CARTESIAN_POINT('Ctrl Pts',(-0.00198939065074527,-0.035383998804013,
-0.0124134984631273));
#43268=CARTESIAN_POINT('Ctrl Pts',(-0.00199999275787943,-0.0353745340044099,
-0.0122946447989551));
#43269=CARTESIAN_POINT('Ctrl Pts',(-0.00199999999627945,-0.0353650692048068,
-0.0121759752791308));
#43270=CARTESIAN_POINT('Ctrl Pts',(-0.00200002462140399,-0.0353328698419498,
-0.0117722601357449));
#43271=CARTESIAN_POINT('Ctrl Pts',(-0.00187350998838232,-0.0353006704790928,
-0.0113673097625285));
#43272=CARTESIAN_POINT('Ctrl Pts',(-0.0016426421671473,-0.0352684711162358,
-0.0110349208999945));
#43273=CARTESIAN_POINT('Ctrl Pts',(-0.00157478002737553,-0.0352590063166328,
-0.0109372172905127));
#43274=CARTESIAN_POINT('Ctrl Pts',(-0.00149823330755494,-0.0352495415170299,
-0.0108456724683233));
#43275=CARTESIAN_POINT('Ctrl Pts',(-0.00141432301966507,-0.0352400767174269,
-0.0107617491899494));
#43276=CARTESIAN_POINT('Ctrl Pts',(-0.00112880558550729,-0.03520787130656,
-0.0104761875537067));
#43277=CARTESIAN_POINT('Ctrl Pts',(-0.000752914192981799,-0.035175665895693,
-0.0102792891629694));
#43278=CARTESIAN_POINT('Ctrl Pts',(-0.000354559808701529,-0.0351434604848261,
-0.010207532341678));
#43279=CARTESIAN_POINT('Ctrl Pts',(-0.000237562848704204,-0.0351340017332331,
-0.0101864573133077));
#43280=CARTESIAN_POINT('Ctrl Pts',(-0.00011878408890704,-0.0351245429816401,
-0.0101758644203822));
#43281=CARTESIAN_POINT('Ctrl Pts',(-1.87611382613396E-7,-0.0351150842300471,
-0.0101758532953576));
#43282=CARTESIAN_POINT('Ctrl Pts',(0.000402124731635335,-0.0350829975054256,
-0.01017581555617));
#43283=CARTESIAN_POINT('Ctrl Pts',(0.000805793279976232,-0.0350509107808041,
-0.010301472403883));
#43284=CARTESIAN_POINT('Ctrl Pts',(0.00113747058010921,-0.0350188240561825,
-0.0105308120471401));
#43285=CARTESIAN_POINT('Ctrl Pts',(0.00123647160816373,-0.0350092466183441,
-0.010599266718132));
#43286=CARTESIAN_POINT('Ctrl Pts',(0.00132917239425267,-0.0349996691805057,
-0.0106766172816647));
#43287=CARTESIAN_POINT('Ctrl Pts',(0.0014140576927508,-0.0349900917426673,
-0.0107614838717402));
#43288=CARTESIAN_POINT('Ctrl Pts',(0.00170378251600591,-0.034957402672427,
-0.0110511448406587));
#43289=CARTESIAN_POINT('Ctrl Pts',(0.00190207010452223,-0.0349247136021869,
-0.0114334574315659));
#43290=CARTESIAN_POINT('Ctrl Pts',(0.00197137654199078,-0.0348920245319466,
-0.0118386967506753));
#43291=CARTESIAN_POINT('Ctrl Pts',(0.00199040527737932,-0.0348830494397269,
-0.0119499590237631));
#43292=CARTESIAN_POINT('Ctrl Pts',(0.00199998570320917,-0.0348740743475072,
-0.0120628112991658));
#43293=CARTESIAN_POINT('Ctrl Pts',(0.00199999998396862,-0.0348650992552875,
-0.0121756000563658));
#43294=CARTESIAN_POINT('',(0.00151022347084785,-0.033978774491363,-0.0108646610549993));
#43295=CARTESIAN_POINT('Ctrl Pts',(0.00199999999999937,-0.0348650793296435,
-0.0121758517007548));
#43296=CARTESIAN_POINT('Ctrl Pts',(0.00200000032705075,-0.0348322521293468,
-0.012588325784795));
#43297=CARTESIAN_POINT('Ctrl Pts',(0.0018681630713516,-0.0347994249290503,
-0.0130003324786179));
#43298=CARTESIAN_POINT('Ctrl Pts',(0.00162913623717455,-0.0347665977287537,
-0.0133359891065054));
#43299=CARTESIAN_POINT('Ctrl Pts',(0.00159926749830595,-0.0347624956492662,
-0.0133779326824323));
#43300=CARTESIAN_POINT('Ctrl Pts',(0.00156778734423012,-0.0347583935697786,
-0.0134187091307775));
#43301=CARTESIAN_POINT('Ctrl Pts',(0.00153479466821863,-0.0347542914902911,
-0.0134581969715379));
#43302=CARTESIAN_POINT('Ctrl Pts',(0.00127462777450834,-0.0347219441512135,
-0.0137695821064207));
#43303=CARTESIAN_POINT('Ctrl Pts',(0.000915968269259364,-0.0346895968121359,
-0.0139996029213947));
#43304=CARTESIAN_POINT('Ctrl Pts',(0.000523877086159381,-0.0346572494730582,
-0.0141060223979567));
#43305=CARTESIAN_POINT('Ctrl Pts',(0.000468336811576201,-0.0346526674264021,
-0.0141210968683962));
#43306=CARTESIAN_POINT('Ctrl Pts',(0.000412168092072666,-0.034648085379746,
-0.0141337662396896));
#43307=CARTESIAN_POINT('Ctrl Pts',(0.000355589182912084,-0.0346435033330899,
-0.0141439885291154));
#43308=CARTESIAN_POINT('Ctrl Pts',(-4.50978435600636E-5,-0.034611053668064,
-0.0142163819141155));
#43309=CARTESIAN_POINT('Ctrl Pts',(-0.000469128586302042,-0.0345786040030382,
-0.0141623070471811));
#43310=CARTESIAN_POINT('Ctrl Pts',(-0.000839059891153366,-0.0345461543380124,
-0.0139913362798846));
#43311=CARTESIAN_POINT('Ctrl Pts',(-0.000890129414537668,-0.0345416746173045,
-0.0139677335312554));
#43312=CARTESIAN_POINT('Ctrl Pts',(-0.000940182994600609,-0.0345371948965965,
-0.0139419834046748));
#43313=CARTESIAN_POINT('Ctrl Pts',(-0.000989039558319999,-0.0345327151758886,
-0.0139141860372357));
#43314=CARTESIAN_POINT('Ctrl Pts',(-0.00134282545405926,-0.0345002760953913,
-0.0137128964705946));
#43315=CARTESIAN_POINT('Ctrl Pts',(-0.0016334871013328,-0.0344678370148941,
-0.013399653616246));
#43316=CARTESIAN_POINT('Ctrl Pts',(-0.00180776228675333,-0.0344353979343968,
-0.0130314206507045));
#43317=CARTESIAN_POINT('Ctrl Pts',(-0.00183188592915287,-0.0344309076291604,
-0.012980448847926));
#43318=CARTESIAN_POINT('Ctrl Pts',(-0.00185384300905548,-0.0344264173239238,
-0.0129284757178915));
#43319=CARTESIAN_POINT('Ctrl Pts',(-0.00187355828541564,-0.0344219270186873,
-0.0128756956624903));
#43320=CARTESIAN_POINT('Ctrl Pts',(-0.00201598633945715,-0.0343894879381893,
-0.0124943994307929));
#43321=CARTESIAN_POINT('Ctrl Pts',(-0.0020382020764351,-0.0343570488576914,
-0.01206765550411));
#43322=CARTESIAN_POINT('Ctrl Pts',(-0.00193583731724208,-0.0343246097771934,
-0.0116733257936057));
#43323=CARTESIAN_POINT('Ctrl Pts',(-0.00192166771048669,-0.0343201194719576,
-0.0116187416088349));
#43324=CARTESIAN_POINT('Ctrl Pts',(-0.00190519331909169,-0.0343156291667219,
-0.0115647779859285));
#43325=CARTESIAN_POINT('Ctrl Pts',(-0.00188648100612665,-0.0343111388614861,
-0.0115116323793869));
#43326=CARTESIAN_POINT('Ctrl Pts',(-0.00175125450020657,-0.0342786891964616,
-0.0111275700408051));
#43327=CARTESIAN_POINT('Ctrl Pts',(-0.00149456243379751,-0.0342462395314371,
-0.0107857583555539));
#43328=CARTESIAN_POINT('Ctrl Pts',(-0.00116302081515074,-0.0342137898664127,
-0.0105487753586376));
#43329=CARTESIAN_POINT('Ctrl Pts',(-0.00111725104051885,-0.0342093101457034,
-0.0105160595312711));
#43330=CARTESIAN_POINT('Ctrl Pts',(-0.00107011722766352,-0.0342048304249941,
-0.0104852886495492));
#43331=CARTESIAN_POINT('Ctrl Pts',(-0.00102179595564649,-0.0342003507042848,
-0.0104565705800132));
#43332=CARTESIAN_POINT('Ctrl Pts',(-0.000672875861731956,-0.0341680033652071,
-0.0102492020422803));
#43333=CARTESIAN_POINT('Ctrl Pts',(-0.000258148398025065,-0.0341356560261293,
-0.0101514162840617));
#43334=CARTESIAN_POINT('Ctrl Pts',(0.000146938291752795,-0.0341033086870516,
-0.0101812583055114));
#43335=CARTESIAN_POINT('Ctrl Pts',(0.000204319398366628,-0.0340987266403956,
-0.0101854854703568));
#43336=CARTESIAN_POINT('Ctrl Pts',(0.000261492385574115,-0.0340941445937395,
-0.010192188646196));
#43337=CARTESIAN_POINT('Ctrl Pts',(0.000318237676841534,-0.0340895625470835,
-0.0102013344132529));
#43338=CARTESIAN_POINT('Ctrl Pts',(0.000724778513515946,-0.0340567353461015,
-0.0102668575202505));
#43339=CARTESIAN_POINT('Ctrl Pts',(0.00111065972736407,-0.0340239081451195,
-0.0104621803986175));
#43340=CARTESIAN_POINT('Ctrl Pts',(0.00140441949822839,-0.0339910809441375,
-0.0107519130234164));
#43341=CARTESIAN_POINT('Ctrl Pts',(0.00144112829092725,-0.0339869787932127,
-0.0107881185761051));
#43342=CARTESIAN_POINT('Ctrl Pts',(0.00147643170979932,-0.0339828766422878,
-0.0108257399041348));
#43343=CARTESIAN_POINT('Ctrl Pts',(0.00151022347084785,-0.033978774491363,
-0.0108646610549993));
#43344=CARTESIAN_POINT('',(-0.00169751808661698,-0.0339787743898723,-0.0111182936685657));
#43345=CARTESIAN_POINT('Origin',(0.,-0.0339787743898823,-0.0121758532865581));
#43346=CARTESIAN_POINT('',(0.0020000130015625,-0.0345673401423348,-0.0121758452034492));
#43347=CARTESIAN_POINT('Ctrl Pts',(-0.00169751808661312,-0.0339787743898749,
-0.0111182936685678));
#43348=CARTESIAN_POINT('Ctrl Pts',(-0.0019133302484519,-0.03401125030809,
-0.0114646937499832));
#43349=CARTESIAN_POINT('Ctrl Pts',(-0.00201817591253676,-0.034041195055471,
-0.0118800195650646));
#43350=CARTESIAN_POINT('Ctrl Pts',(-0.00199618519646481,-0.0340749668219992,
-0.012287326618901));
#43351=CARTESIAN_POINT('Ctrl Pts',(-0.00198495985050248,-0.0340922059042464,
-0.0124952399300115));
#43352=CARTESIAN_POINT('Ctrl Pts',(-0.00194135350589726,-0.0341100889178837,
-0.012701077025495));
#43353=CARTESIAN_POINT('Ctrl Pts',(-0.00186710706940351,-0.0341270620260995,
-0.0128946273200806));
#43354=CARTESIAN_POINT('Ctrl Pts',(-0.00185372474489184,-0.034130121292683,
-0.0129295132078591));
#43355=CARTESIAN_POINT('Ctrl Pts',(-0.00183936109686421,-0.0341331408248404,
-0.0129640224176434));
#43356=CARTESIAN_POINT('Ctrl Pts',(-0.00182399630821732,-0.0341361278602697,
-0.0129980955529474));
#43357=CARTESIAN_POINT('Ctrl Pts',(-0.00167662706547824,-0.0341647775969737,
-0.0133249033120966));
#43358=CARTESIAN_POINT('Ctrl Pts',(-0.0014356238739396,-0.0341904378226505,
-0.0136128782517713));
#43359=CARTESIAN_POINT('Ctrl Pts',(-0.0011393861182615,-0.0342194947185986,
-0.0138186255099517));
#43360=CARTESIAN_POINT('Ctrl Pts',(-0.00095945763406348,-0.0342371432564478,
-0.0139435919991406));
#43361=CARTESIAN_POINT('Ctrl Pts',(-0.000759448108284487,-0.0342558025273501,
-0.0140389235176684));
#43362=CARTESIAN_POINT('Ctrl Pts',(-0.000550305419734492,-0.034273777241299,
-0.0140995996071181));
#43363=CARTESIAN_POINT('Ctrl Pts',(-0.00047822934401059,-0.034279971800873,
-0.0141205101847153));
#43364=CARTESIAN_POINT('Ctrl Pts',(-0.000404945039041054,-0.0342860347339131,
-0.0141374504388133));
#43365=CARTESIAN_POINT('Ctrl Pts',(-0.000330820056329016,-0.0342920074279103,
-0.0141499875472947));
#43366=CARTESIAN_POINT('Ctrl Pts',(-1.38987420090911E-5,-0.0343175436771257,
-0.0142035899462743));
#43367=CARTESIAN_POINT('Ctrl Pts',(0.000319303757953489,-0.034341430366152,
-0.0141758977409307));
#43368=CARTESIAN_POINT('Ctrl Pts',(0.000625857835872285,-0.0343669021623781,
-0.0140747561372667));
#43369=CARTESIAN_POINT('Ctrl Pts',(0.000833909794261486,-0.0343841893474794,
-0.0140061134075409));
#43370=CARTESIAN_POINT('Ctrl Pts',(0.00103028204907868,-0.0344024350641547,
-0.0139035910702775));
#43371=CARTESIAN_POINT('Ctrl Pts',(0.00120436386342799,-0.0344205562780359,
-0.0137730316152375));
#43372=CARTESIAN_POINT('Ctrl Pts',(0.00129433949622915,-0.034429922378063,
-0.0137055508756249));
#43373=CARTESIAN_POINT('Ctrl Pts',(0.00137898091997455,-0.0344389951962281,
-0.0136307290564667));
#43374=CARTESIAN_POINT('Ctrl Pts',(0.0014564302820324,-0.0344478989440412,
-0.0135488195897293));
#43375=CARTESIAN_POINT('Ctrl Pts',(0.00165855072246001,-0.0344711351513078,
-0.013335059565731));
#43376=CARTESIAN_POINT('Ctrl Pts',(0.00181152170565784,-0.0344932198896048,
-0.0130723078730732));
#43377=CARTESIAN_POINT('Ctrl Pts',(0.00190227021810968,-0.0345163608536293,
-0.0127910916953787));
#43378=CARTESIAN_POINT('Ctrl Pts',(0.00196634393264011,-0.0345326997167445,
-0.0125925367592799));
#43379=CARTESIAN_POINT('Ctrl Pts',(0.0019995103779209,-0.0345498932533823,
-0.0123841045160361));
#43380=CARTESIAN_POINT('Ctrl Pts',(0.0020000130015625,-0.0345673401423348,
-0.0121758452034492));
#43381=CARTESIAN_POINT('Ctrl Pts',(0.00199999995026977,-0.0345673849471511,
-0.0121754072810601));
#43382=CARTESIAN_POINT('Ctrl Pts',(0.00199997483940943,-0.0345769756133014,
-0.0120628039170363));
#43383=CARTESIAN_POINT('Ctrl Pts',(0.00199044020054723,-0.0345866097090282,
-0.0119503946982784));
#43384=CARTESIAN_POINT('Ctrl Pts',(0.00196689070359113,-0.0345981735004672,
-0.0118124124127049));
#43385=CARTESIAN_POINT('Ctrl Pts',(0.00196173542751688,-0.0346004120463131,
-0.0117855423331393));
#43386=CARTESIAN_POINT('Ctrl Pts',(0.0019519162326337,-0.0346042167170265,
-0.0117394908298653));
#43387=CARTESIAN_POINT('Ctrl Pts',(0.00194751723602006,-0.0346057952830513,
-0.0117202592932969));
#43388=CARTESIAN_POINT('Ctrl Pts',(0.00193622838000297,-0.0346095634041527,
-0.0116740625413711));
#43389=CARTESIAN_POINT('Ctrl Pts',(0.0019290591281148,-0.0346117384194698,
-0.0116471705825984));
#43390=CARTESIAN_POINT('Ctrl Pts',(0.00188992727544227,-0.0346226345829043,
-0.0115118037274921));
#43391=CARTESIAN_POINT('Ctrl Pts',(0.00184936335889547,-0.0346309859424247,
-0.011406016331714));
#43392=CARTESIAN_POINT('Ctrl Pts',(0.00174871055688625,-0.0346480914081593,
-0.0111981529790634));
#43393=CARTESIAN_POINT('Ctrl Pts',(0.00168808606614052,-0.0346568196365459,
-0.011096850275457));
#43394=CARTESIAN_POINT('Ctrl Pts',(0.00159420933613803,-0.0346690772020404,
-0.0109674390119659));
#43395=CARTESIAN_POINT('Ctrl Pts',(0.00156845062042185,-0.0346723350491007,
-0.0109341888235039));
#43396=CARTESIAN_POINT('Ctrl Pts',(0.0015198909108764,-0.0346783141498106,
-0.0108754303230239));
#43397=CARTESIAN_POINT('Ctrl Pts',(0.00149744660900956,-0.0346810206556933,
-0.0108496475581069));
#43398=CARTESIAN_POINT('Ctrl Pts',(0.00144520509277452,-0.0346872046453558,
-0.0107926529359178));
#43399=CARTESIAN_POINT('Ctrl Pts',(0.00141503726758382,-0.0346906966565683,
-0.0107618059292982));
#43400=CARTESIAN_POINT('Ctrl Pts',(0.0012870616409788,-0.0347052139341774,
-0.010639147773148));
#43401=CARTESIAN_POINT('Ctrl Pts',(0.00118114979711425,-0.0347165846630359,
-0.0105563271783615));
#43402=CARTESIAN_POINT('Ctrl Pts',(0.000987151030180866,-0.0347361398669616,
-0.0104338362117405));
#43403=CARTESIAN_POINT('Ctrl Pts',(0.000902987008983808,-0.0347442619514332,
-0.0103887582938902));
#43404=CARTESIAN_POINT('Ctrl Pts',(0.000790806107578523,-0.0347544167303081,
-0.0103386319094809));
#43405=CARTESIAN_POINT('Ctrl Pts',(0.000765460603026857,-0.0347566686338392,
-0.0103279282403209));
#43406=CARTESIAN_POINT('Ctrl Pts',(0.000721582832399333,-0.0347604858640932,
-0.0103104560210856));
#43407=CARTESIAN_POINT('Ctrl Pts',(0.000703158745241538,-0.0347620639457492,
-0.0103034332983042));
#43408=CARTESIAN_POINT('Ctrl Pts',(0.000658663085280927,-0.0347658175142602,
-0.0102872223561991));
#43409=CARTESIAN_POINT('Ctrl Pts',(0.000632499734172252,-0.034767978883676,
-0.0102783000826411));
#43410=CARTESIAN_POINT('Ctrl Pts',(0.00049542523263479,-0.0347791082681094,
-0.0102347052184396));
#43411=CARTESIAN_POINT('Ctrl Pts',(0.000381818583535505,-0.0347876849627012,
-0.010209200331013));
#43412=CARTESIAN_POINT('Ctrl Pts',(0.000152699183736938,-0.0348048163840472,
-0.0101783805649375));
#43413=CARTESIAN_POINT('Ctrl Pts',(3.76752542759658E-5,-0.0348133421599191,
-0.0101729077919167));
#43414=CARTESIAN_POINT('Ctrl Pts',(-0.000119663222632085,-0.0348254146126436,
-0.010178983556825));
#43415=CARTESIAN_POINT('Ctrl Pts',(-0.000162085934081661,-0.0348287088161045,
-0.0101819787509695));
#43416=CARTESIAN_POINT('Ctrl Pts',(-0.000238718750367696,-0.0348347518383239,
-0.010189851002067));
#43417=CARTESIAN_POINT('Ctrl Pts',(-0.000272959951319575,-0.0348374856203169,
-0.0101942669799029));
#43418=CARTESIAN_POINT('Ctrl Pts',(-0.000350188852032124,-0.0348437374656436,
-0.0102062665053244));
#43419=CARTESIAN_POINT('Ctrl Pts',(-0.000393075562394101,-0.0348472703156863,
-0.0102143754414659));
#43420=CARTESIAN_POINT('Ctrl Pts',(-0.000561439542848433,-0.0348613991661833,
-0.010251952482215));
#43421=CARTESIAN_POINT('Ctrl Pts',(-0.000684191800726341,-0.0348723039615588,
-0.0102921123733125));
#43422=CARTESIAN_POINT('Ctrl Pts',(-0.000893472808505717,-0.0348917542728829,
-0.010383750454362));
#43423=CARTESIAN_POINT('Ctrl Pts',(-0.000981632432394317,-0.0349002397578543,
-0.0104304800640631));
#43424=CARTESIAN_POINT('Ctrl Pts',(-0.00108875635346201,-0.0349106863121,
-0.010497956926511));
#43425=CARTESIAN_POINT('Ctrl Pts',(-0.00111127305248858,-0.0349128897294522,
-0.0105127841343851));
#43426=CARTESIAN_POINT('Ctrl Pts',(-0.00114985736006802,-0.034916670317033,
-0.0105393255720873));
#43427=CARTESIAN_POINT('Ctrl Pts',(-0.00116606079257463,-0.034918258806829,
-0.0105508310641559));
#43428=CARTESIAN_POINT('Ctrl Pts',(-0.00120531444845609,-0.0349221110952953,
-0.0105795933214726));
#43429=CARTESIAN_POINT('Ctrl Pts',(-0.00122816824723893,-0.0349243586670241,
-0.0105971095450949));
#43430=CARTESIAN_POINT('Ctrl Pts',(-0.00131300200722041,-0.0349327541595328,
-0.0106650877875477));
#43431=CARTESIAN_POINT('Ctrl Pts',(-0.00137232240937095,-0.0349387352068917,
-0.0107187600380388));
#43432=CARTESIAN_POINT('Ctrl Pts',(-0.00149853119746944,-0.0349521372694498,
-0.0108475171474998));
#43433=CARTESIAN_POINT('Ctrl Pts',(-0.00156328883612012,-0.0349595204109482,
-0.0109243741651363));
#43434=CARTESIAN_POINT('Ctrl Pts',(-0.00166076931043963,-0.0349720322915117,
-0.0110595039264108));
#43435=CARTESIAN_POINT('Ctrl Pts',(-0.00169683695489829,-0.0349770647267152,
-0.0111151302090635));
#43436=CARTESIAN_POINT('Ctrl Pts',(-0.00174870684972281,-0.034985067715539,
-0.0112045636919352));
#43437=CARTESIAN_POINT('Ctrl Pts',(-0.00176643891152485,-0.034987970477539,
-0.0112371987444787));
#43438=CARTESIAN_POINT('Ctrl Pts',(-0.00179918394341318,-0.034993685646959,
-0.0113016820149685));
#43439=CARTESIAN_POINT('Ctrl Pts',(-0.00181428474557568,-0.0349964937921137,
-0.0113334704610511));
#43440=CARTESIAN_POINT('Ctrl Pts',(-0.00185067358125213,-0.0350037348267818,
-0.0114155948575722));
#43441=CARTESIAN_POINT('Ctrl Pts',(-0.00187075009031881,-0.0350082049994866,
-0.0114664319964782));
#43442=CARTESIAN_POINT('Ctrl Pts',(-0.00193419812995889,-0.0350241963055464,
-0.011648599706018));
#43443=CARTESIAN_POINT('Ctrl Pts',(-0.00196600887230118,-0.0350360251620521,
-0.0117835285781764));
#43444=CARTESIAN_POINT('Ctrl Pts',(-0.00198996515492455,-0.0350519731611638,
-0.0119697260665178));
#43445=CARTESIAN_POINT('Ctrl Pts',(-0.00199445707108768,-0.035056157491469,
-0.0120190370210945));
#43446=CARTESIAN_POINT('Ctrl Pts',(-0.00199903654565857,-0.0350632737818721,
-0.0121042034331366));
#43447=CARTESIAN_POINT('Ctrl Pts',(-0.00199999873973495,-0.0350662302741379,
-0.012139988480039));
#43448=CARTESIAN_POINT('Ctrl Pts',(-0.00200000065241236,-0.0350706548672094,
-0.012194366349962));
#43449=CARTESIAN_POINT('Ctrl Pts',(-0.00199974229911636,-0.0350721548928912,
-0.0122129502063218));
#43450=CARTESIAN_POINT('Ctrl Pts',(-0.00199860808936163,-0.0350754121797412,
-0.0122536777462656));
#43451=CARTESIAN_POINT('Ctrl Pts',(-0.00199762321779275,-0.0350771635311815,
-0.0122758160272709));
#43452=CARTESIAN_POINT('Ctrl Pts',(-0.0019934803562801,-0.0350824765634891,
-0.0123435598832444));
#43453=CARTESIAN_POINT('Ctrl Pts',(-0.00198912655141246,-0.0350859825684029,
-0.0123890804093612));
#43454=CARTESIAN_POINT('Ctrl Pts',(-0.0019736725436104,-0.0350950380550717,
-0.0125076150744442));
#43455=CARTESIAN_POINT('Ctrl Pts',(-0.00196008325081081,-0.0351005129899465,
-0.0125802346121602));
#43456=CARTESIAN_POINT('Ctrl Pts',(-0.0019137695678505,-0.035114931685053,
-0.0127692015068076));
#43457=CARTESIAN_POINT('Ctrl Pts',(-0.00187447486150728,-0.0351238520759617,
-0.0128836074782262));
#43458=CARTESIAN_POINT('Ctrl Pts',(-0.00180723040578281,-0.0351364284662211,
-0.0130336581885925));
#43459=CARTESIAN_POINT('Ctrl Pts',(-0.00178805117458491,-0.0351398071943819,
-0.0130729505283266));
#43460=CARTESIAN_POINT('Ctrl Pts',(-0.00175149615408346,-0.0351459238130408,
-0.0131420034616443));
#43461=CARTESIAN_POINT('Ctrl Pts',(-0.00173460920616686,-0.0351486442047253,
-0.0131720036533968));
#43462=CARTESIAN_POINT('Ctrl Pts',(-0.00169568658560429,-0.0351547029606944,
-0.013237157800672));
#43463=CARTESIAN_POINT('Ctrl Pts',(-0.00167331483111333,-0.0351580522666305,
-0.0132720910509075));
#43464=CARTESIAN_POINT('Ctrl Pts',(-0.00158051715943771,-0.0351714607924919,
-0.0134075281256136));
#43465=CARTESIAN_POINT('Ctrl Pts',(-0.00150200227905443,-0.0351818052950829,
-0.0135021401457446));
#43466=CARTESIAN_POINT('Ctrl Pts',(-0.00133778802172592,-0.0352015913119727,
-0.0136666141690022));
#43467=CARTESIAN_POINT('Ctrl Pts',(-0.00125397812454458,-0.0352109749229107,
-0.0137377711810139));
#43468=CARTESIAN_POINT('Ctrl Pts',(-0.00114182175525152,-0.035222384656903,
-0.0138181195134375));
#43469=CARTESIAN_POINT('Ctrl Pts',(-0.00111855024356905,-0.0352246947194777,
-0.0138340573963449));
#43470=CARTESIAN_POINT('Ctrl Pts',(-0.00107838833744979,-0.0352285756230006,
-0.0138603324864408));
#43471=CARTESIAN_POINT('Ctrl Pts',(-0.00106166919308336,-0.0352301604434166,
-0.0138709197193575));
#43472=CARTESIAN_POINT('Ctrl Pts',(-0.00102158310188005,-0.0352338884136959,
-0.0138954779170239));
#43473=CARTESIAN_POINT('Ctrl Pts',(-0.000998083357425043,-0.0352360184463566,
-0.0139092230484048));
#43474=CARTESIAN_POINT('Ctrl Pts',(-0.000889279314656027,-0.0352456650693163,
-0.0139699162735517));
#43475=CARTESIAN_POINT('Ctrl Pts',(-0.000800888487752885,-0.0352529103857152,
-0.0140110813988215));
#43476=CARTESIAN_POINT('Ctrl Pts',(-0.000586615777225301,-0.0352699090418459,
-0.0140924269270901));
#43477=CARTESIAN_POINT('Ctrl Pts',(-0.000459081788695746,-0.0352796175782822,
-0.0141269073572777));
#43478=CARTESIAN_POINT('Ctrl Pts',(-0.000286248237428606,-0.0352930338543174,
-0.0141557392557054));
#43479=CARTESIAN_POINT('Ctrl Pts',(-0.000243188114020568,-0.0352963945638124,
-0.0141614880783893));
#43480=CARTESIAN_POINT('Ctrl Pts',(-0.000165713831305937,-0.0353024965358647,
-0.0141692736644648));
#43481=CARTESIAN_POINT('Ctrl Pts',(-0.000131368843978521,-0.0353052208480643,
-0.0141718311962366));
#43482=CARTESIAN_POINT('Ctrl Pts',(-5.45483947135336E-5,-0.0353113669895284,
-0.0141755604897042));
#43483=CARTESIAN_POINT('Ctrl Pts',(-1.20684192265568E-5,-0.0353148015805928,
-0.014176267802333));
#43484=CARTESIAN_POINT('Ctrl Pts',(7.83048016157863E-5,-0.0353221937572267,
-0.0141748940247873));
#43485=CARTESIAN_POINT('Ctrl Pts',(0.000126165274681745,-0.0353261597189562,
-0.0141724446682545));
#43486=CARTESIAN_POINT('Ctrl Pts',(0.00027393749543109,-0.0353385616109294,
-0.0141595479101425));
#43487=CARTESIAN_POINT('Ctrl Pts',(0.000373179803022596,-0.0353471219346769,
-0.0141432932043279));
#43488=CARTESIAN_POINT('Ctrl Pts',(0.000548378756239798,-0.035362467552961,
-0.0141008615326838));
#43489=CARTESIAN_POINT('Ctrl Pts',(0.000624797031384798,-0.0353692413967702,
-0.0140774334156359));
#43490=CARTESIAN_POINT('Ctrl Pts',(0.000726573730253065,-0.0353782323347577,
-0.014039430136805));
#43491=CARTESIAN_POINT('Ctrl Pts',(0.000753313452461783,-0.0353805911473329,
-0.0140287826303499));
#43492=CARTESIAN_POINT('Ctrl Pts',(0.000798070260597117,-0.0353845234895327,
-0.0140098316993986));
#43493=CARTESIAN_POINT('Ctrl Pts',(0.00081620873945973,-0.0353861120986209,
-0.0140018314816055));
#43494=CARTESIAN_POINT('Ctrl Pts',(0.000858565343023737,-0.0353898098612445,
-0.0139823921396538));
#43495=CARTESIAN_POINT('Ctrl Pts',(0.000882677875008957,-0.0353919068556627,
-0.0139707340770382));
#43496=CARTESIAN_POINT('Ctrl Pts',(0.000994736329718761,-0.0354016484619153,
-0.0139137506661006));
#43497=CARTESIAN_POINT('Ctrl Pts',(0.001079485148541,-0.0354090088379031,
-0.0138624192183537));
#43498=CARTESIAN_POINT('Ctrl Pts',(0.00126680944704866,-0.0354260636087769,
-0.013729029416039));
#43499=CARTESIAN_POINT('Ctrl Pts',(0.00136578886684921,-0.0354357153013449,
-0.0136427474726699));
#43500=CARTESIAN_POINT('Ctrl Pts',(0.00148544052246622,-0.0354490731896195,
-0.0135157628432833));
#43501=CARTESIAN_POINT('Ctrl Pts',(0.00151422094899876,-0.0354524377619177,
-0.0134831503312042));
#43502=CARTESIAN_POINT('Ctrl Pts',(0.00156383602610512,-0.0354585423023707,
-0.0134230909067011));
#43503=CARTESIAN_POINT('Ctrl Pts',(0.0015850681169543,-0.0354612651874825,
-0.0133959940877483));
#43504=CARTESIAN_POINT('Ctrl Pts',(0.00163086033395229,-0.0354674020236707,
-0.0133343397489836));
#43505=CARTESIAN_POINT('Ctrl Pts',(0.00165504141611922,-0.035470828589713,
-0.0132995230256753));
#43506=CARTESIAN_POINT('Ctrl Pts',(0.00170407702405112,-0.0354781992810384,
-0.0132238999679976));
#43507=CARTESIAN_POINT('Ctrl Pts',(0.00172861195724907,-0.0354821516636666,
-0.0131829185097587));
#43508=CARTESIAN_POINT('Ctrl Pts',(0.00179973977550545,-0.0354944722425904,
-0.0130538414235223));
#43509=CARTESIAN_POINT('Ctrl Pts',(0.00184123316714173,-0.0355029629885641,
-0.0129631167484504));
#43510=CARTESIAN_POINT('Ctrl Pts',(0.00190616342975048,-0.0355188990899091,
-0.0127875767393077));
#43511=CARTESIAN_POINT('Ctrl Pts',(0.00193111423094824,-0.0355263276072942,
-0.0127035516828114));
#43512=CARTESIAN_POINT('Ctrl Pts',(0.00195615753835482,-0.03553565914942,
-0.0125931144816554));
#43513=CARTESIAN_POINT('Ctrl Pts',(0.00196135334137623,-0.0355377554687445,
-0.0125679661213739));
#43514=CARTESIAN_POINT('Ctrl Pts',(0.00196970595692743,-0.0355414285559199,
-0.0125232042463192));
#43515=CARTESIAN_POINT('Ctrl Pts',(0.001973057165011,-0.0355430142357201,
-0.0125036333072206));
#43516=CARTESIAN_POINT('Ctrl Pts',(0.00197923994578229,-0.0355461881986183,
-0.0124639853683421));
#43517=CARTESIAN_POINT('Ctrl Pts',(0.00198205861943998,-0.0355477760296057,
-0.0124439103299233));
#43518=CARTESIAN_POINT('Ctrl Pts',(0.00198821423343565,-0.0355516338130169,
-0.0123946396116975));
#43519=CARTESIAN_POINT('Ctrl Pts',(0.00199121403430999,-0.0355538891471154,
-0.0123654058551468));
#43520=CARTESIAN_POINT('Ctrl Pts',(0.00199783185008784,-0.0355601727511544,
-0.0122830837495095));
#43521=CARTESIAN_POINT('Ctrl Pts',(0.00199997753046282,-0.0355641540731492,
-0.0122299001841672));
#43522=CARTESIAN_POINT('Ctrl Pts',(0.00199999982444772,-0.0355681130672164,
-0.0121766912657388));
#43523=CARTESIAN_POINT('Ctrl Pts',(0.00191,-0.0443987743898723,-0.0121758532865581));
#43524=CARTESIAN_POINT('Ctrl Pts',(0.00191,-0.0443987743898723,-0.0116043826229051));
#43525=CARTESIAN_POINT('Ctrl Pts',(0.00136396443998201,-0.0443987743898723,
-0.0104664461719892));
#43526=CARTESIAN_POINT('Ctrl Pts',(-0.000486154511932736,-0.0443987743898723,
-0.0100448167983067));
#43527=CARTESIAN_POINT('Ctrl Pts',(-0.00197136971063077,-0.0443987743898723,
-0.0112269996519921));
#43528=CARTESIAN_POINT('Ctrl Pts',(-0.00196863290544544,-0.0443987743898723,
-0.0131236113412357));
#43529=CARTESIAN_POINT('Ctrl Pts',(-0.00048737056446968,-0.0443987743898723,
-0.014309575135295));
#43530=CARTESIAN_POINT('Ctrl Pts',(0.00136372235516645,-0.0443987743898723,
-0.0138834315669214));
#43531=CARTESIAN_POINT('Ctrl Pts',(0.00191,-0.0443987743898723,-0.0127473239502111));
#43532=CARTESIAN_POINT('Ctrl Pts',(0.00191,-0.0443987743898723,-0.0121758532865581));
#43533=CARTESIAN_POINT('Ctrl Pts',(0.00192589648945146,-0.0443775790706037,
-0.0121758532865581));
#43534=CARTESIAN_POINT('Ctrl Pts',(0.00192589648945146,-0.0443775790706037,
-0.0115996618695963));
#43535=CARTESIAN_POINT('Ctrl Pts',(0.00137530035187607,-0.0443775790706037,
-0.0104522100376602));
#43536=CARTESIAN_POINT('Ctrl Pts',(-0.00049019929686441,-0.0443775790706037,
-0.0100270915893122));
#43537=CARTESIAN_POINT('Ctrl Pts',(-0.001987759617862,-0.0443775790706037,
-0.0112191030790215));
#43538=CARTESIAN_POINT('Ctrl Pts',(-0.00198501905754235,-0.0443775790706037,
-0.0131315055658264));
#43539=CARTESIAN_POINT('Ctrl Pts',(-0.000491417921724576,-0.0443775790706037,
-0.0143273048600502));
#43540=CARTESIAN_POINT('Ctrl Pts',(0.00137506056245648,-0.0443775790706037,
-0.0138976640310167));
#43541=CARTESIAN_POINT('Ctrl Pts',(0.00192589648945146,-0.0443775790706037,
-0.0127520447035199));
#43542=CARTESIAN_POINT('Ctrl Pts',(0.00192589648945146,-0.0443775790706037,
-0.0121758532865581));
#43543=CARTESIAN_POINT('Ctrl Pts',(0.00195438855983192,-0.0443409009516712,
-0.0121758532865581));
#43544=CARTESIAN_POINT('Ctrl Pts',(0.00195438855983192,-0.0443409009516712,
-0.0115910921262162));
#43545=CARTESIAN_POINT('Ctrl Pts',(0.00139566737358033,-0.0443409009516712,
-0.0104267218465327));
#43546=CARTESIAN_POINT('Ctrl Pts',(-0.000497453148499854,-0.0443409009516712,
-0.00999528841693408));
#43547=CARTESIAN_POINT('Ctrl Pts',(-0.00201718914033432,-0.0443409009516712,
-0.0112049480760704));
#43548=CARTESIAN_POINT('Ctrl Pts',(-0.00201438365174801,-0.0443409009516711,
-0.0131456356479581));
#43549=CARTESIAN_POINT('Ctrl Pts',(-0.000498699477980959,-0.0443409009516712,
-0.0143591706870349));
#43550=CARTESIAN_POINT('Ctrl Pts',(0.00139541851169272,-0.0443409009516711,
-0.0139231103056061));
#43551=CARTESIAN_POINT('Ctrl Pts',(0.00195438855983192,-0.0443409009516712,
-0.0127606144469));
#43552=CARTESIAN_POINT('Ctrl Pts',(0.00195438855983192,-0.0443409009516712,
-0.0121758532865581));
#43553=CARTESIAN_POINT('Ctrl Pts',(0.00201714899795489,-0.0442974094567112,
-0.0121758532865581));
#43554=CARTESIAN_POINT('Ctrl Pts',(0.00201714899795489,-0.0442974094567112,
-0.0115723431648622));
#43555=CARTESIAN_POINT('Ctrl Pts',(0.00144047261468403,-0.0442974094567112,
-0.0103705452165039));
#43556=CARTESIAN_POINT('Ctrl Pts',(-0.000513426520915583,-0.0442974094567112,
-0.00992527387087597));
#43557=CARTESIAN_POINT('Ctrl Pts',(-0.00208195197224179,-0.0442974094567112,
-0.0111737702411527));
#43558=CARTESIAN_POINT('Ctrl Pts',(-0.00207907206613982,-0.0442974094567112,
-0.0131767830034219));
#43559=CARTESIAN_POINT('Ctrl Pts',(-0.000514706653486131,-0.0442974094567112,
-0.0144292589295152));
#43560=CARTESIAN_POINT('Ctrl Pts',(0.00144021931264795,-0.0442974094567112,
-0.0139792362605124));
#43561=CARTESIAN_POINT('Ctrl Pts',(0.00201714899795489,-0.0442974094567112,
-0.0127793634082539));
#43562=CARTESIAN_POINT('Ctrl Pts',(0.00201714899795489,-0.0442974094567112,
-0.0121758532865581));
#43563=CARTESIAN_POINT('Ctrl Pts',(0.00208712894978359,-0.0442779545242776,
-0.0121758532865581));
#43564=CARTESIAN_POINT('Ctrl Pts',(0.00208712894978359,-0.0442779545242776,
-0.0115513687696672));
#43565=CARTESIAN_POINT('Ctrl Pts',(0.00149046301531559,-0.0442779545242776,
-0.0103079241157742));
#43566=CARTESIAN_POINT('Ctrl Pts',(-0.000531240003705059,-0.0442779545242776,
-0.00984718420843915));
#43567=CARTESIAN_POINT('Ctrl Pts',(-0.00215419825785711,-0.0442779545242776,
-0.0111390049289695));
#43568=CARTESIAN_POINT('Ctrl Pts',(-0.00215119853182699,-0.0442779545242776,
-0.0132115012185179));
#43569=CARTESIAN_POINT('Ctrl Pts',(-0.000532572447509192,-0.0442779545242776,
-0.0145074653054627));
#43570=CARTESIAN_POINT('Ctrl Pts',(0.00149019641460847,-0.0442779545242776,
-0.0140417784860521));
#43571=CARTESIAN_POINT('Ctrl Pts',(0.00208712894978359,-0.0442779545242776,
-0.012800337803449));
#43572=CARTESIAN_POINT('Ctrl Pts',(0.00208712894978359,-0.0442779545242776,
-0.0121758532865581));
#43573=CARTESIAN_POINT('Ctrl Pts',(0.00213650829037307,-0.0442788253127506,
-0.0121758532865581));
#43574=CARTESIAN_POINT('Ctrl Pts',(0.00213650829037307,-0.0442788253127506,
-0.0115366660068379));
#43575=CARTESIAN_POINT('Ctrl Pts',(0.00152569330952636,-0.0442788253127506,
-0.0102637123012538));
#43576=CARTESIAN_POINT('Ctrl Pts',(-0.000543805828570658,-0.0442788253127506,
-0.00979211240677498));
#43577=CARTESIAN_POINT('Ctrl Pts',(-0.00220512921753389,-0.0442788253127506,
-0.0111144752032848));
#43578=CARTESIAN_POINT('Ctrl Pts',(-0.00220209708826565,-0.0442788253127506,
-0.0132360162688478));
#43579=CARTESIAN_POINT('Ctrl Pts',(-0.000545154492334908,-0.0442788253127506,
-0.0145625705770762));
#43580=CARTESIAN_POINT('Ctrl Pts',(0.00152542913999413,-0.0442788253127506,
-0.0140859663070167));
#43581=CARTESIAN_POINT('Ctrl Pts',(0.00213650829037307,-0.0442788253127506,
-0.0128150405662783));
#43582=CARTESIAN_POINT('Ctrl Pts',(0.00213650829037307,-0.0442788253127506,
-0.0121758532865581));
#43583=CARTESIAN_POINT('Ctrl Pts',(0.00215960599488205,-0.0442787671797737,
-0.0121758532865581));
#43584=CARTESIAN_POINT('Ctrl Pts',(0.00215960599488205,-0.0442787671797737,
-0.0115296726592007));
#43585=CARTESIAN_POINT('Ctrl Pts',(0.00154222513336241,-0.0442787671797737,
-0.0102430616280669));
#43586=CARTESIAN_POINT('Ctrl Pts',(-0.000549688095030464,-0.0442787671797737,
-0.00976631629653212));
#43587=CARTESIAN_POINT('Ctrl Pts',(-0.0022290094390271,-0.0442787671797737,
-0.0111029994762258));
#43588=CARTESIAN_POINT('Ctrl Pts',(-0.00222589994608779,-0.0442787671797737,
-0.0132474629929249));
#43589=CARTESIAN_POINT('Ctrl Pts',(-0.000551069030812133,-0.0442787671797737,
-0.0145884406624534));
#43590=CARTESIAN_POINT('Ctrl Pts',(0.00154194800605399,-0.0442787671797737,
-0.0141065679844921));
#43591=CARTESIAN_POINT('Ctrl Pts',(0.00215960599488205,-0.0442787671797737,
-0.0128220339139153));
#43592=CARTESIAN_POINT('Ctrl Pts',(0.00215960599488205,-0.0442787671797737,
-0.0121758532865581));
#43593=CARTESIAN_POINT('Ctrl Pts',(-0.00190884695647825,-0.0443979099380992,
-0.0121758537542897));
#43594=CARTESIAN_POINT('Ctrl Pts',(-0.0019086387602771,-0.0443977537577689,
-0.0124605928222598));
#43595=CARTESIAN_POINT('Ctrl Pts',(-0.00184659890197118,-0.0443980578198581,
-0.0127480326817812));
#43596=CARTESIAN_POINT('Ctrl Pts',(-0.00162944389721798,-0.0443983362855908,
-0.0131986267652795));
#43597=CARTESIAN_POINT('Ctrl Pts',(-0.00150149968284053,-0.0443983738682118,
-0.0133748516475149));
#43598=CARTESIAN_POINT('Ctrl Pts',(-0.00109784916003133,-0.0443975727756485,
-0.0137769070334325));
#43599=CARTESIAN_POINT('Ctrl Pts',(-0.00077347669762607,-0.0443981434538313,
-0.0139620860896191));
#43600=CARTESIAN_POINT('Ctrl Pts',(-0.000286256574005507,-0.0443982288725065,
-0.0140731128679073));
#43601=CARTESIAN_POINT('Ctrl Pts',(-0.000142992270597617,-0.0443981711685123,
-0.0140879545366855));
#43602=CARTESIAN_POINT('Ctrl Pts',(0.000427615134630929,-0.0443972050126916,
-0.0140840813965754));
#43603=CARTESIAN_POINT('Ctrl Pts',(0.000857946456805267,-0.0443983417280292,
-0.0139371451114233));
#43604=CARTESIAN_POINT('Ctrl Pts',(0.00124787970615935,-0.044398339904063,
-0.0136260912098367));
#43605=CARTESIAN_POINT('Ctrl Pts',(0.00130109284701091,-0.0443983077589567,
-0.0135781506662894));
#43606=CARTESIAN_POINT('Ctrl Pts',(0.00170253954223259,-0.0443976850210757,
-0.0131724039571971));
#43607=CARTESIAN_POINT('Ctrl Pts',(0.00191,-0.0443987743898723,-0.0126747526877388));
#43608=CARTESIAN_POINT('Ctrl Pts',(0.00191,-0.0443987743898723,-0.0121758532865581));
#43609=CARTESIAN_POINT('Origin',(0.,-0.0442787743898823,-0.0121758532865581));
#43610=CARTESIAN_POINT('Origin',(0.,-0.0442787743898723,-0.0121758532865581));
#43611=CARTESIAN_POINT('',(0.00379145188432738,-0.0442787743898723,-0.0117428405846659));
#43612=CARTESIAN_POINT('',(0.00379145188432738,-0.0442787743898723,-0.0126088659884503));
#43613=CARTESIAN_POINT('',(0.00379145188433738,-0.0442787743898823,-0.0121758532865681));
#43614=CARTESIAN_POINT('',(0.00227072594216369,-0.0442787743898723,-0.00910886598845032));
#43615=CARTESIAN_POINT('',(0.00404145188433738,-0.0442787743898823,-0.0121758532865681));
#43616=CARTESIAN_POINT('',(0.00152072594216369,-0.0442787743898723,-0.0086758532865581));
#43617=CARTESIAN_POINT('',(0.00189572594217369,-0.0442787743898823,-0.00889235963749421));
#43618=CARTESIAN_POINT('',(-0.00152072594216369,-0.0442787743898723,-0.0086758532865581));
#43619=CARTESIAN_POINT('',(0.00202072594217369,-0.0442787743898823,-0.0086758532865481));
#43620=CARTESIAN_POINT('',(-0.00227072594216369,-0.0442787743898723,-0.00910886598845032));
#43621=CARTESIAN_POINT('',(-0.00189572594217369,-0.0442787743898823,-0.00889235963749421));
#43622=CARTESIAN_POINT('',(-0.00379145188432738,-0.0442787743898723,-0.0117428405846659));
#43623=CARTESIAN_POINT('',(-0.00202072594217369,-0.0442787743898823,-0.0086758532865481));
#43624=CARTESIAN_POINT('',(-0.00379145188432738,-0.0442787743898723,-0.0126088659884503));
#43625=CARTESIAN_POINT('',(-0.00379145188433738,-0.0442787743898823,-0.0121758532865481));
#43626=CARTESIAN_POINT('',(-0.00227072594216369,-0.0442787743898723,-0.0152428405846659));
#43627=CARTESIAN_POINT('',(-0.00404145188433738,-0.0442787743898823,-0.0121758532865481));
#43628=CARTESIAN_POINT('',(-0.0015207259421637,-0.0442787743898723,-0.0156758532865581));
#43629=CARTESIAN_POINT('',(-0.0018957259421737,-0.0442787743898823,-0.015459346935622));
#43630=CARTESIAN_POINT('',(0.00152072594216369,-0.0442787743898723,-0.0156758532865581));
#43631=CARTESIAN_POINT('',(-0.00202072594217369,-0.0442787743898823,-0.0156758532865681));
#43632=CARTESIAN_POINT('',(0.00227072594216369,-0.0442787743898723,-0.0152428405846659));
#43633=CARTESIAN_POINT('',(0.0018957259421737,-0.0442787743898823,-0.015459346935622));
#43634=CARTESIAN_POINT('',(0.00202072594217369,-0.0442787743898823,-0.0156758532865681));
#43635=CARTESIAN_POINT('Origin',(0.,-0.0452787743898723,-0.0121758532865581));
#43636=CARTESIAN_POINT('',(0.000499999999998797,-0.0462787743898739,-0.0121758532865581));
#43637=CARTESIAN_POINT('',(0.00125,-0.0452787743898723,-0.0121758532865581));
#43638=CARTESIAN_POINT('Origin',(0.,-0.0462787743898823,-0.0121758532865581));
#43639=CARTESIAN_POINT('Origin',(0.00389145188432738,-0.0441787743898723,
-0.0121758532865581));
#43640=CARTESIAN_POINT('',(0.00399145188432738,-0.0440787743898723,-0.0122624558269365));
#43641=CARTESIAN_POINT('',(0.00347816150747191,-0.0445920647667478,-0.0131515008387137));
#43642=CARTESIAN_POINT('',(0.00399145188432738,-0.0440787743898723,-0.0120892507461797));
#43643=CARTESIAN_POINT('',(0.00399145188433738,-0.0440787743898823,-0.0121758532865681));
#43644=CARTESIAN_POINT('',(0.00428645188433738,-0.0437837743898823,-0.0126002057344225));
#43645=CARTESIAN_POINT('Origin',(0.00202072594216369,-0.0412787743898723,
-0.0156758532865581));
#43646=CARTESIAN_POINT('',(0.00207072594216369,-0.0440787743898723,-0.0155892507461796));
#43647=CARTESIAN_POINT('',(0.00177572594217369,-0.0437837743898823,-0.0161002057344224));
#43648=CARTESIAN_POINT('',(0.00207072594216369,-0.0414787743898723,-0.0155892507461796));
#43649=CARTESIAN_POINT('',(0.00207072594217369,-0.0412787743898823,-0.0155892507461896));
#43650=CARTESIAN_POINT('',(0.00227072594216369,-0.0412787743898723,-0.0152428405846659));
#43651=CARTESIAN_POINT('',(0.00207572594217369,-0.0414737743898823,-0.0155805904921518));
#43652=CARTESIAN_POINT('',(0.00379145188432738,-0.0412787743898723,-0.0126088659884503));
#43653=CARTESIAN_POINT('',(0.00202072594217369,-0.0412787743898823,-0.0156758532865681));
#43654=CARTESIAN_POINT('',(0.00399145188432738,-0.0414787743898723,-0.0122624558269365));
#43655=CARTESIAN_POINT('',(0.0031781615074719,-0.0406654840130169,-0.0136711160809844));
#43656=CARTESIAN_POINT('',(0.00399145188433738,-0.0412787743898823,-0.0122624558269465));
#43657=CARTESIAN_POINT('',(0.00265608891323529,-0.0427787743898723,-0.0145753723394213));
#43658=CARTESIAN_POINT('Origin',(0.00303108891325554,-0.0427787743898823,
-0.0139258532865681));
#43659=CARTESIAN_POINT('Origin',(0.00194572594216369,-0.0441787743898723,
-0.00880575709712576));
#43660=CARTESIAN_POINT('',(0.00207072594216369,-0.0440787743898723,-0.00876245582693654));
#43661=CARTESIAN_POINT('',(0.00258401631903916,-0.0445920647667478,-0.00965150083869371));
#43662=CARTESIAN_POINT('',(0.00192072594216369,-0.0440787743898723,-0.0086758532865581));
#43663=CARTESIAN_POINT('',(0.00199572594217369,-0.0440787743898823,-0.00871915455673732));
#43664=CARTESIAN_POINT('',(0.00251072594217369,-0.0437837743898823,-0.0086758532865481));
#43665=CARTESIAN_POINT('Origin',(0.00202072594216369,-0.0412787743898723,
-0.0086758532865581));
#43666=CARTESIAN_POINT('',(0.00192072594216369,-0.0414787743898723,-0.0086758532865581));
#43667=CARTESIAN_POINT('',(0.00192072594217369,-0.0412787743898823,-0.0086758532865481));
#43668=CARTESIAN_POINT('',(0.00152072594216369,-0.0412787743898723,-0.0086758532865581));
#43669=CARTESIAN_POINT('',(0.00191072594217369,-0.0414737743898823,-0.0086758532865481));
#43670=CARTESIAN_POINT('',(-0.00152072594216369,-0.0412787743898723,-0.0086758532865581));
#43671=CARTESIAN_POINT('',(0.00202072594217369,-0.0412787743898823,-0.0086758532865481));
#43672=CARTESIAN_POINT('',(-0.00192072594216369,-0.0414787743898723,-0.0086758532865581));
#43673=CARTESIAN_POINT('',(-0.000294145188442734,-0.0406654840130169,-0.0086758532865481));
#43674=CARTESIAN_POINT('',(-0.00192072594216369,-0.0440787743898723,-0.0086758532865581));
#43675=CARTESIAN_POINT('',(-0.00192072594217369,-0.0412787743898823,-0.0086758532865481));
#43676=CARTESIAN_POINT('',(-0.000894145188442733,-0.0445920647667478,-0.0086758532865481));
#43677=CARTESIAN_POINT('',(0.000750000000026109,-0.0427787743898723,-0.00867585328655462));
#43678=CARTESIAN_POINT('Origin',(1.00022748892833E-14,-0.0427787743898823,
-0.0086758532865481));
#43679=CARTESIAN_POINT('Origin',(-0.00194572594216369,-0.0441787743898723,
-0.00880575709712576));
#43680=CARTESIAN_POINT('',(-0.00207072594216369,-0.0440787743898723,-0.00876245582693654));
#43681=CARTESIAN_POINT('',(-0.00199572594217369,-0.0440787743898823,-0.00871915455673732));
#43682=CARTESIAN_POINT('',(-0.00177572594217369,-0.0437837743898823,-0.00825150083869372));
#43683=CARTESIAN_POINT('Origin',(-0.00389145188432738,-0.0441787743898723,
-0.0121758532865581));
#43684=CARTESIAN_POINT('',(-0.00399145188432738,-0.0440787743898723,-0.0120892507461797));
#43685=CARTESIAN_POINT('',(-0.00347816150747191,-0.0445920647667478,-0.0112002057344025));
#43686=CARTESIAN_POINT('',(-0.00399145188432738,-0.0440787743898723,-0.0122624558269365));
#43687=CARTESIAN_POINT('',(-0.00399145188433738,-0.0440787743898823,-0.0121758532865481));
#43688=CARTESIAN_POINT('',(-0.00428645188433738,-0.0437837743898823,-0.0117515008386937));
#43689=CARTESIAN_POINT('Origin',(-0.00404145188432738,-0.0412787743898723,
-0.0121758532865581));
#43690=CARTESIAN_POINT('',(-0.00399145188432738,-0.0414787743898723,-0.0122624558269365));
#43691=CARTESIAN_POINT('',(-0.00399145188433738,-0.0412787743898823,-0.0122624558269465));
#43692=CARTESIAN_POINT('',(-0.00379145188432738,-0.0412787743898723,-0.0126088659884503));
#43693=CARTESIAN_POINT('',(-0.00398645188433738,-0.0414737743898823,-0.0122711160809844));
#43694=CARTESIAN_POINT('',(-0.00227072594216369,-0.0412787743898723,-0.0152428405846659));
#43695=CARTESIAN_POINT('',(-0.00404145188433738,-0.0412787743898823,-0.0121758532865481));
#43696=CARTESIAN_POINT('',(-0.00207072594216369,-0.0414787743898723,-0.0155892507461796));
#43697=CARTESIAN_POINT('',(-0.00288401631903917,-0.0406654840130169,-0.0141805904921518));
#43698=CARTESIAN_POINT('',(-0.00207072594216369,-0.0440787743898723,-0.0155892507461796));
#43699=CARTESIAN_POINT('',(-0.00207072594217369,-0.0412787743898823,-0.0155892507461896));
#43700=CARTESIAN_POINT('',(-0.00258401631903917,-0.0445920647667478,-0.0147002057344225));
#43701=CARTESIAN_POINT('Origin',(-0.0019457259421637,-0.0441787743898723,
-0.0155459494759905));
#43702=CARTESIAN_POINT('',(-0.00192072594216369,-0.0440787743898723,-0.0156758532865581));
#43703=CARTESIAN_POINT('',(-0.0019957259421737,-0.0440787743898823,-0.0156325520163788));
#43704=CARTESIAN_POINT('',(-0.0025107259421737,-0.0437837743898823,-0.0156758532865681));
#43705=CARTESIAN_POINT('Origin',(0.0019457259421637,-0.0441787743898723,
-0.0155459494759905));
#43706=CARTESIAN_POINT('',(0.00192072594216369,-0.0440787743898723,-0.0156758532865581));
#43707=CARTESIAN_POINT('',(0.00089414518844275,-0.0445920647667478,-0.0156758532865681));
#43708=CARTESIAN_POINT('',(0.0019957259421737,-0.0440787743898823,-0.0156325520163788));
#43709=CARTESIAN_POINT('Origin',(0.0019457259421637,-0.0413787743898723,
-0.0155459494759905));
#43710=CARTESIAN_POINT('',(0.00192072594216369,-0.0414787743898723,-0.0156758532865581));
#43711=CARTESIAN_POINT('',(0.0019957259421737,-0.0414787743898823,-0.0156325520163788));
#43712=CARTESIAN_POINT('',(0.00152072594216369,-0.0412787743898723,-0.0156758532865581));
#43713=CARTESIAN_POINT('',(0.000294145188442746,-0.0406654840130168,-0.0156758532865681));
#43714=CARTESIAN_POINT('',(0.0018957259421737,-0.0412787743898823,-0.015459346935622));
#43715=CARTESIAN_POINT('Origin',(0.,-0.0412787743898723,-0.0121758532865581));
#43716=CARTESIAN_POINT('',(-0.0015207259421637,-0.0412787743898723,-0.0156758532865581));
#43717=CARTESIAN_POINT('',(-0.00202072594217369,-0.0412787743898823,-0.0156758532865681));
#43718=CARTESIAN_POINT('',(-0.0018957259421737,-0.0412787743898823,-0.015459346935622));
#43719=CARTESIAN_POINT('',(-0.00379145188432738,-0.0412787743898723,-0.0117428405846659));
#43720=CARTESIAN_POINT('',(-0.00379145188433738,-0.0412787743898823,-0.0121758532865481));
#43721=CARTESIAN_POINT('',(-0.00227072594216369,-0.0412787743898723,-0.00910886598845032));
#43722=CARTESIAN_POINT('',(-0.00202072594217369,-0.0412787743898823,-0.0086758532865481));
#43723=CARTESIAN_POINT('',(-0.00189572594217369,-0.0412787743898823,-0.00889235963749421));
#43724=CARTESIAN_POINT('',(0.00227072594216369,-0.0412787743898723,-0.00910886598845032));
#43725=CARTESIAN_POINT('',(0.00189572594217369,-0.0412787743898823,-0.00889235963749421));
#43726=CARTESIAN_POINT('',(0.00379145188432738,-0.0412787743898723,-0.0117428405846659));
#43727=CARTESIAN_POINT('',(0.00404145188433738,-0.0412787743898823,-0.0121758532865681));
#43728=CARTESIAN_POINT('',(0.00379145188433738,-0.0412787743898823,-0.0121758532865681));
#43729=CARTESIAN_POINT('',(0.00270000000001,-0.0412787743898823,-0.0121758532865581));
#43730=CARTESIAN_POINT('Origin',(5.55111512312578E-19,-0.0412787743898823,
-0.0121758532865581));
#43731=CARTESIAN_POINT('Origin',(-0.0019457259421637,-0.0413787743898723,
-0.0155459494759905));
#43732=CARTESIAN_POINT('',(-0.00192072594216369,-0.0414787743898723,-0.0156758532865581));
#43733=CARTESIAN_POINT('',(-0.00191072594217369,-0.0414737743898823,-0.0156758532865681));
#43734=CARTESIAN_POINT('',(-0.0019957259421737,-0.0414787743898823,-0.0156325520163788));
#43735=CARTESIAN_POINT('Origin',(-0.00389145188432738,-0.0413787743898723,
-0.0121758532865581));
#43736=CARTESIAN_POINT('',(-0.00399145188432738,-0.0414787743898723,-0.0120892507461797));
#43737=CARTESIAN_POINT('',(-0.00399145188433738,-0.0414787743898823,-0.0121758532865481));
#43738=CARTESIAN_POINT('',(-0.0031781615074719,-0.0406654840130169,-0.0106805904921318));
#43739=CARTESIAN_POINT('Origin',(-0.00194572594216369,-0.0413787743898723,
-0.00880575709712576));
#43740=CARTESIAN_POINT('',(-0.00207072594216369,-0.0414787743898723,-0.00876245582693654));
#43741=CARTESIAN_POINT('',(-0.00207572594217369,-0.0414737743898823,-0.00877111608096439));
#43742=CARTESIAN_POINT('',(-0.00199572594217369,-0.0414787743898823,-0.00871915455673732));
#43743=CARTESIAN_POINT('Origin',(0.00194572594216369,-0.0413787743898723,
-0.00880575709712576));
#43744=CARTESIAN_POINT('',(0.00207072594216369,-0.0414787743898723,-0.00876245582693654));
#43745=CARTESIAN_POINT('',(0.00199572594217369,-0.0414787743898823,-0.00871915455673732));
#43746=CARTESIAN_POINT('',(0.00288401631903916,-0.0406654840130168,-0.0101711160809644));
#43747=CARTESIAN_POINT('Origin',(0.00404145188432738,-0.0412787743898723,
-0.0121758532865581));
#43748=CARTESIAN_POINT('',(0.00399145188432738,-0.0414787743898723,-0.0120892507461797));
#43749=CARTESIAN_POINT('',(0.00399145188433738,-0.0412787743898823,-0.0120892507461697));
#43750=CARTESIAN_POINT('',(0.00398645188433738,-0.0414737743898823,-0.0120805904921318));
#43751=CARTESIAN_POINT('',(0.00207072594217369,-0.0412787743898823,-0.00876245582692654));
#43752=CARTESIAN_POINT('',(0.00340608891326195,-0.0427787743898723,-0.0110753723394177));
#43753=CARTESIAN_POINT('Origin',(0.00303108891325554,-0.0427787743898823,
-0.0104258532865481));
#43754=CARTESIAN_POINT('Origin',(0.00199572594216369,-0.0412787743898723,
-0.00871915455674732));
#43755=CARTESIAN_POINT('Origin',(-0.00199572594216369,-0.0412787743898723,
-0.00871915455674732));
#43756=CARTESIAN_POINT('',(-0.00207072594217369,-0.0412787743898823,-0.00876245582692654));
#43757=CARTESIAN_POINT('Origin',(-0.00202072594216369,-0.0412787743898723,
-0.0086758532865581));
#43758=CARTESIAN_POINT('',(-0.00399145188433738,-0.0412787743898823,-0.0120892507461696));
#43759=CARTESIAN_POINT('Origin',(-0.00399145188432738,-0.0412787743898723,
-0.0121758532865581));
#43760=CARTESIAN_POINT('Origin',(-0.00199572594216369,-0.0412787743898723,
-0.0156325520163689));
#43761=CARTESIAN_POINT('',(-0.00192072594217369,-0.0412787743898823,-0.0156758532865681));
#43762=CARTESIAN_POINT('Origin',(-0.00202072594216369,-0.0412787743898723,
-0.0156758532865581));
#43763=CARTESIAN_POINT('',(0.00192072594217369,-0.0412787743898823,-0.0156758532865681));
#43764=CARTESIAN_POINT('Origin',(0.00199572594216369,-0.0412787743898723,
-0.0156325520163689));
#43765=CARTESIAN_POINT('Origin',(0.00389145188432738,-0.0413787743898723,
-0.0121758532865581));
#43766=CARTESIAN_POINT('',(0.00399145188433738,-0.0414787743898823,-0.0121758532865681));
#43767=CARTESIAN_POINT('Origin',(0.00399145188432738,-0.0412787743898723,
-0.0121758532865581));
#43768=CARTESIAN_POINT('Ctrl Pts',(0.00270918054975648,-0.0412787503570556,
-0.0121758532865581));
#43769=CARTESIAN_POINT('Ctrl Pts',(0.00270918054975648,-0.0412787503570556,
-0.0113652728041599));
#43770=CARTESIAN_POINT('Ctrl Pts',(0.00193513294480066,-0.0412787503570556,
-0.00975168114383156));
#43771=CARTESIAN_POINT('Ctrl Pts',(-0.00069000520119527,-0.0412787503570556,
-0.00915299470268466));
#43772=CARTESIAN_POINT('Ctrl Pts',(-0.00279540565516726,-0.0412787503570556,
-0.0108302679555478));
#43773=CARTESIAN_POINT('Ctrl Pts',(-0.00279272352454856,-0.0412787503570556,
-0.0135201078666651));
#43774=CARTESIAN_POINT('Ctrl Pts',(-0.000690883461576721,-0.0412787503570556,
-0.0152020993353227));
#43775=CARTESIAN_POINT('Ctrl Pts',(0.00193418739257031,-0.0412787503570556,
-0.01459810269407));
#43776=CARTESIAN_POINT('Ctrl Pts',(0.00270918054975648,-0.0412787503570556,
-0.0129864337689563));
#43777=CARTESIAN_POINT('Ctrl Pts',(0.00270918054975648,-0.0412787503570556,
-0.0121758532865581));
#43778=CARTESIAN_POINT('Ctrl Pts',(0.00267614195234609,-0.0412788886794323,
-0.0121758532865581));
#43779=CARTESIAN_POINT('Ctrl Pts',(0.00267614195234609,-0.0412788886794323,
-0.0113751391161252));
#43780=CARTESIAN_POINT('Ctrl Pts',(0.00191154067064816,-0.0412788886794323,
-0.00978125017196854));
#43781=CARTESIAN_POINT('Ctrl Pts',(-0.000681589977327022,-0.0412788886794323,
-0.00918985318007107));
#43782=CARTESIAN_POINT('Ctrl Pts',(-0.00276132283802881,-0.0412788886794323,
-0.0108466776255854));
#43783=CARTESIAN_POINT('Ctrl Pts',(-0.00275866480260235,-0.0412788886794323,
-0.013503712356313));
#43784=CARTESIAN_POINT('Ctrl Pts',(-0.000682462010447489,-0.0412788886794323,
-0.0151652074941981));
#43785=CARTESIAN_POINT('Ctrl Pts',(0.00191060490329316,-0.0412788886794323,
-0.014568552060673));
#43786=CARTESIAN_POINT('Ctrl Pts',(0.00267614195234609,-0.0412788886794323,
-0.012976567456991));
#43787=CARTESIAN_POINT('Ctrl Pts',(0.00267614195234609,-0.0412788886794323,
-0.0121758532865581));
#43788=CARTESIAN_POINT('Ctrl Pts',(0.00261368928777976,-0.0412787942793926,
-0.0121758532865581));
#43789=CARTESIAN_POINT('Ctrl Pts',(0.00261368928777976,-0.0412787942793926,
-0.0113938502436242));
#43790=CARTESIAN_POINT('Ctrl Pts',(0.00186692234954223,-0.0412787942793926,
-0.00983712445344849));
#43791=CARTESIAN_POINT('Ctrl Pts',(-0.000665684594985857,-0.0412787942793926,
-0.00925954420041668));
#43792=CARTESIAN_POINT('Ctrl Pts',(-0.00269687259383373,-0.0412787942793926,
-0.0108776961201086));
#43793=CARTESIAN_POINT('Ctrl Pts',(-0.00269428806701916,-0.0412787942793926,
-0.0134727273438823));
#43794=CARTESIAN_POINT('Ctrl Pts',(-0.000666530303291745,-0.0412787942793926,
-0.0150954276100709));
#43795=CARTESIAN_POINT('Ctrl Pts',(0.00186601074701434,-0.0412787942793926,
-0.0145127289543036));
#43796=CARTESIAN_POINT('Ctrl Pts',(0.00261368928777976,-0.0412787942793926,
-0.012957856329492));
#43797=CARTESIAN_POINT('Ctrl Pts',(0.00261368928777976,-0.0412787942793926,
-0.0121758532865581));
#43798=CARTESIAN_POINT('Ctrl Pts',(0.00253433766292927,-0.0412183037740197,
-0.0121758532865581));
#43799=CARTESIAN_POINT('Ctrl Pts',(0.00253433766292927,-0.0412183037740197,
-0.0114175510782768));
#43800=CARTESIAN_POINT('Ctrl Pts',(0.00181025729792705,-0.0412183037740197,
-0.00990814158877628));
#43801=CARTESIAN_POINT('Ctrl Pts',(-0.000645473156809493,-0.0412183037740197,
-0.00934807153777405));
#43802=CARTESIAN_POINT('Ctrl Pts',(-0.00261501139357923,-0.0412183037740197,
-0.0109171085874015));
#43803=CARTESIAN_POINT('Ctrl Pts',(-0.00261248660679668,-0.0412183037740197,
-0.0134333493339249));
#43804=CARTESIAN_POINT('Ctrl Pts',(-0.000646302936028143,-0.0412183037740197,
-0.0150068184163061));
#43805=CARTESIAN_POINT('Ctrl Pts',(0.00180936957537367,-0.0412183037740197,
-0.0144417570953774));
#43806=CARTESIAN_POINT('Ctrl Pts',(0.00253433766292927,-0.0412183037740197,
-0.0129341554948394));
#43807=CARTESIAN_POINT('Ctrl Pts',(0.00253433766292927,-0.0412183037740197,
-0.0121758532865581));
#43808=CARTESIAN_POINT('Ctrl Pts',(0.00250057355266071,-0.0411453162532137,
-0.0121758532865581));
#43809=CARTESIAN_POINT('Ctrl Pts',(0.00250057355266071,-0.0411453162532137,
-0.011427734754967));
#43810=CARTESIAN_POINT('Ctrl Pts',(0.00178611059073584,-0.0411453162532137,
-0.00993832706908355));
#43811=CARTESIAN_POINT('Ctrl Pts',(-0.000636876223173571,-0.0411453162532137,
-0.00938576861420257));
#43812=CARTESIAN_POINT('Ctrl Pts',(-0.00258014094469067,-0.0411453162532137,
-0.0109338776021103));
#43813=CARTESIAN_POINT('Ctrl Pts',(-0.00257768702246746,-0.0411453162532137,
-0.0134166058963254));
#43814=CARTESIAN_POINT('Ctrl Pts',(-0.00063767557125981,-0.0411453162532137,
-0.014969044583688));
#43815=CARTESIAN_POINT('Ctrl Pts',(0.00178524224201209,-0.0411453162532137,
-0.0144116175405293));
#43816=CARTESIAN_POINT('Ctrl Pts',(0.00250057355266071,-0.0411453162532137,
-0.0129239718181492));
#43817=CARTESIAN_POINT('Ctrl Pts',(0.00250057355266071,-0.0411453162532137,
-0.0121758532865581));
#43818=CARTESIAN_POINT('Ctrl Pts',(0.0025,-0.041101214337398,-0.0121758532865581));
#43819=CARTESIAN_POINT('Ctrl Pts',(0.0025,-0.041101214337398,-0.0114277797728648));
#43820=CARTESIAN_POINT('Ctrl Pts',(0.00178574661104337,-0.041101214337398,
-0.00993888160219718));
#43821=CARTESIAN_POINT('Ctrl Pts',(-0.000636726266562143,-0.041101214337398,
-0.00938637186566609));
#43822=CARTESIAN_POINT('Ctrl Pts',(-0.0025795983978868,-0.041101214337398,
-0.0109341637345287));
#43823=CARTESIAN_POINT('Ctrl Pts',(-0.00257708691874699,-0.041101214337398,
-0.0134163060846059));
#43824=CARTESIAN_POINT('Ctrl Pts',(-0.000637555681479932,-0.041101214337398,
-0.0149684942391342));
#43825=CARTESIAN_POINT('Ctrl Pts',(0.00178486667912529,-0.041101214337398,
-0.0144110293156704));
#43826=CARTESIAN_POINT('Ctrl Pts',(0.0025,-0.041101214337398,-0.0129239268002514));
#43827=CARTESIAN_POINT('Ctrl Pts',(0.0025,-0.041101214337398,-0.0121758532865581));
#43828=CARTESIAN_POINT('Ctrl Pts',(0.0025,-0.0410787743898723,-0.0121758532865581));
#43829=CARTESIAN_POINT('Ctrl Pts',(0.0025,-0.0410787743898723,-0.0114278550357034));
#43830=CARTESIAN_POINT('Ctrl Pts',(0.00178571943910354,-0.0410787743898723,
-0.00993885703610024));
#43831=CARTESIAN_POINT('Ctrl Pts',(-0.000636728572014028,-0.0410787743898723,
-0.00938639369106591));
#43832=CARTESIAN_POINT('Ctrl Pts',(-0.0025795691101196,-0.0410787743898723,
-0.0109341629839093));
#43833=CARTESIAN_POINT('Ctrl Pts',(-0.00257709218909681,-0.0410787743898723,
-0.0134163151357684));
#43834=CARTESIAN_POINT('Ctrl Pts',(-0.000637540000123396,-0.0410787743898723,
-0.0149684405315022));
#43835=CARTESIAN_POINT('Ctrl Pts',(0.00178484651300112,-0.0410787743898723,
-0.0144110741552401));
#43836=CARTESIAN_POINT('Ctrl Pts',(0.0025,-0.0410787743898723,-0.0129238515374128));
#43837=CARTESIAN_POINT('Ctrl Pts',(0.0025,-0.0410787743898723,-0.0121758532865581));
#43838=CARTESIAN_POINT('Ctrl Pts',(0.0025,-0.0410787743898723,-0.0121758532865581));
#43839=CARTESIAN_POINT('Ctrl Pts',(0.0025,-0.041101214337398,-0.0121758532865581));
#43840=CARTESIAN_POINT('Ctrl Pts',(0.00250057355266071,-0.0411453162532137,
-0.0121758532865581));
#43841=CARTESIAN_POINT('Ctrl Pts',(0.00253433766292927,-0.0412183037740197,
-0.0121758532865581));
#43842=CARTESIAN_POINT('Ctrl Pts',(0.00261084648764158,-0.0412766271855573,
-0.0121758532865581));
#43843=CARTESIAN_POINT('Ctrl Pts',(0.00267008006997241,-0.0412787743898725,
-0.0121758532865581));
#43844=CARTESIAN_POINT('Ctrl Pts',(0.00270000000001,-0.0412787743898723,
-0.0121758532865581));
#43845=CARTESIAN_POINT('Origin',(2.27488928325654E-18,-0.0427787743898723,
-0.0086758532865581));
#43846=CARTESIAN_POINT('',(2.23368293997689E-18,-0.0427787743898723,-0.0087758532865581));
#43847=CARTESIAN_POINT('',(0.000750000000000002,-0.0427787743898723,-0.0086758532865581));
#43848=CARTESIAN_POINT('Origin',(0.00303108891324554,-0.0427787743898723,
-0.0104258532865581));
#43849=CARTESIAN_POINT('',(0.00294448637286709,-0.0427787743898723,-0.0104758532865581));
#43850=CARTESIAN_POINT('',(0.00340608891324554,-0.0427787743898723,-0.0110753723393964));
#43851=CARTESIAN_POINT('Origin',(0.00303108891324554,-0.0427787743898723,
-0.0139258532865581));
#43852=CARTESIAN_POINT('',(0.00294448637286709,-0.0427787743898723,-0.0138758532865581));
#43853=CARTESIAN_POINT('',(0.00265608891324554,-0.0427787743898723,-0.0145753723393964));
#43854=CARTESIAN_POINT('Origin',(0.,-0.0444787743898723,-0.0121758532865581));
#43855=CARTESIAN_POINT('',(0.000199999999998,-0.0456787743898783,-0.0121758532865581));
#43856=CARTESIAN_POINT('Origin',(0.,-0.0456787743898823,-0.0121758532865581));
#43857=CARTESIAN_POINT('',(0.000999999999998,-0.0432787743898783,-0.0121758532865581));
#43858=CARTESIAN_POINT('',(0.0006,-0.0444787743898723,-0.0121758532865581));
#43859=CARTESIAN_POINT('',(-0.001,-0.0432787743898823,-0.0121758532865581));
#43860=CARTESIAN_POINT('Origin',(0.,-0.0432787743898823,-0.0121758532865581));
#43861=CARTESIAN_POINT('Origin',(0.,-0.0432787743898823,-0.0121758532865581));
#43862=CARTESIAN_POINT('Origin',(0.,-0.0462787743898723,-0.0121758532865581));
#43863=CARTESIAN_POINT('',(0.0002,-0.0462787743898823,-0.0121758532865581));
#43864=CARTESIAN_POINT('Origin',(0.,-0.0462787743898823,-0.0121758532865581));
#43865=CARTESIAN_POINT('',(0.0002,-0.0462787743898723,-0.0121758532865581));
#43866=CARTESIAN_POINT('Origin',(0.,-0.0340287743898723,-0.0121758532865581));
#43867=CARTESIAN_POINT('',(-0.000999999999999024,-0.0342787743898735,-0.0121758532865581));
#43868=CARTESIAN_POINT('Origin',(0.,-0.0342787743898823,-0.0121758532865581));
#43869=CARTESIAN_POINT('',(-0.0014000000000039,-0.0337787743898674,-0.0121758532865581));
#43870=CARTESIAN_POINT('',(-0.0012,-0.0340287743898723,-0.0121758532865581));
#43871=CARTESIAN_POINT('Origin',(0.,-0.0337787743898723,-0.0121758532865581));
#43872=CARTESIAN_POINT('Origin',(0.,-0.0337787743898723,-0.0121758532865581));
#43873=CARTESIAN_POINT('',(-0.002300000000005,-0.0337787743898773,-0.0121758532865581));
#43874=CARTESIAN_POINT('Origin',(0.,-0.0337787743898723,-0.0121758532865581));
#43875=CARTESIAN_POINT('Origin',(0.,-0.0337787743898723,-0.0121758532865581));
#43876=CARTESIAN_POINT('',(-0.001,-0.0337787743898723,-0.0121758532865581));
#43877=CARTESIAN_POINT('Origin',(0.,-0.0338787743898723,-0.0121758532865581));
#43878=CARTESIAN_POINT('',(-0.000786711117161713,-0.0339787743898823,-0.0145488441458292));
#43879=CARTESIAN_POINT('',(-0.00250000000001,-0.0339787743898823,-0.0121758532865581));
#43880=CARTESIAN_POINT('Origin',(0.,-0.0339787743898823,-0.0121758532865581));
#43881=CARTESIAN_POINT('',(-0.0024,-0.0338787743898723,-0.0121758532865581));
#43882=CARTESIAN_POINT('Origin',(0.,-0.0339787743898823,-0.0121758532865581));
#43883=CARTESIAN_POINT('Ctrl Pts',(-0.000771496087389042,-0.0339794895371937,
-0.014554586149909));
#43884=CARTESIAN_POINT('Ctrl Pts',(-0.000773967688123329,-0.0339793735894346,
-0.0145536626403178));
#43885=CARTESIAN_POINT('Ctrl Pts',(-0.000776437811893427,-0.0339792576009297,
-0.0145527351854424));
#43886=CARTESIAN_POINT('Ctrl Pts',(-0.000781509664634019,-0.0339790192212365,
-0.0145508216205089));
#43887=CARTESIAN_POINT('Ctrl Pts',(-0.000784111224758069,-0.0339788968258219,
-0.014549835070045));
#43888=CARTESIAN_POINT('Ctrl Pts',(-0.000786711117158984,-0.0339787743898754,
-0.0145488441458229));
#43889=CARTESIAN_POINT('Origin',(-2.24345254752611E-19,-0.0397787743898723,
-0.0121758532865581));
#43890=CARTESIAN_POINT('Ctrl Pts',(-0.00175719004339857,-0.0397787743898739,
-0.0139541342405783));
#43891=CARTESIAN_POINT('Ctrl Pts',(-0.00169307291765995,-0.0397787746017101,
-0.0140038566338397));
#43892=CARTESIAN_POINT('Ctrl Pts',(-0.00162653221361426,-0.0397787743898809,
-0.0140503442714278));
#43893=CARTESIAN_POINT('Ctrl Pts',(-0.00155787560922398,-0.0397787743898809,
-0.0140935098107271));
#43894=CARTESIAN_POINT('Ctrl Pts',(-0.00143215670016973,-0.0397787743898808,
-0.0141725513619027));
#43895=CARTESIAN_POINT('Ctrl Pts',(-0.00129934194595018,-0.0397787743898807,
-0.0142404794281288));
#43896=CARTESIAN_POINT('Ctrl Pts',(-0.00116123097203325,-0.0397787743898805,
-0.0142964185823052));
#43897=CARTESIAN_POINT('Ctrl Pts',(-0.00113108173522323,-0.0397787743898805,
-0.0143086299421876));
#43898=CARTESIAN_POINT('Ctrl Pts',(-0.00110068007533138,-0.0397787743898804,
-0.0143202682758157));
#43899=CARTESIAN_POINT('Ctrl Pts',(-0.00107004492089912,-0.0397787743898804,
-0.0143313215520188));
#43900=CARTESIAN_POINT('Ctrl Pts',(-0.00105495584662179,-0.0397787743898804,
-0.014336765745421));
#43901=CARTESIAN_POINT('Ctrl Pts',(-0.00103980846841194,-0.0397787743898804,
-0.0143420684573587));
#43902=CARTESIAN_POINT('Ctrl Pts',(-0.00102462359856661,-0.0397787743898804,
-0.014347222153839));
#43903=CARTESIAN_POINT('Ctrl Pts',(-0.000814784928526715,-0.0397787743898801,
-0.0144184407303709));
#43904=CARTESIAN_POINT('Ctrl Pts',(-0.000596993519393736,-0.0397787743898798,
-0.0144616995548158));
#43905=CARTESIAN_POINT('Ctrl Pts',(-0.000377446859808482,-0.0397787743898794,
-0.0144737272746223));
#43906=CARTESIAN_POINT('Ctrl Pts',(-0.000348131916821991,-0.0397787743898793,
-0.0144753332745544));
#43907=CARTESIAN_POINT('Ctrl Pts',(-0.000318786529917582,-0.0397787743898793,
-0.0144763786947731));
#43908=CARTESIAN_POINT('Ctrl Pts',(-0.000289426596251435,-0.0397787743898792,
-0.0144768522077377));
#43909=CARTESIAN_POINT('Ctrl Pts',(-0.000275910077730923,-0.0397787743898792,
-0.0144770702002859));
#43910=CARTESIAN_POINT('Ctrl Pts',(-0.000262390406744024,-0.0397787743898792,
-0.0144771668815114));
#43911=CARTESIAN_POINT('Ctrl Pts',(-0.000248883867653849,-0.0397787743898792,
-0.0144771413739509));
#43912=CARTESIAN_POINT('Ctrl Pts',(-0.000169711581607006,-0.039778774389879,
-0.0144769918543837));
#43913=CARTESIAN_POINT('Ctrl Pts',(-9.08628147936332E-5,-0.0397787743898786,
-0.0144726507129251));
#43914=CARTESIAN_POINT('Ctrl Pts',(-1.26284316727756E-5,-0.0397787743898793,
-0.0144639743441833));
#43915=CARTESIAN_POINT('Ctrl Pts',(2.79176950103316E-5,-0.0397787743898796,
-0.014459477687699));
#43916=CARTESIAN_POINT('Ctrl Pts',(6.82986355817335E-5,-0.0397787743898797,
-0.0144538157856816));
#43917=CARTESIAN_POINT('Ctrl Pts',(0.000108472229486668,-0.0397787743898798,
-0.0144469633457009));
#43918=CARTESIAN_POINT('Ctrl Pts',(0.000264185840183674,-0.0397787743898801,
-0.014420403158579));
#43919=CARTESIAN_POINT('Ctrl Pts',(0.000416825422655187,-0.0397787743898803,
-0.0143759995156889));
#43920=CARTESIAN_POINT('Ctrl Pts',(0.000563929584611809,-0.0397787743898805,
-0.0143151782020699));
#43921=CARTESIAN_POINT('Ctrl Pts',(0.00057535801717517,-0.0397787743898805,
-0.0143104530313347));
#43922=CARTESIAN_POINT('Ctrl Pts',(0.000586751212388327,-0.0397787743898805,
-0.0143056290827273));
#43923=CARTESIAN_POINT('Ctrl Pts',(0.000598097161382955,-0.0397787743898805,
-0.0143007118517534));
#43924=CARTESIAN_POINT('Ctrl Pts',(0.00084134323732603,-0.0397787743898808,
-0.0141952912175276));
#43925=CARTESIAN_POINT('Ctrl Pts',(0.00106470216535388,-0.0397787743898811,
-0.0140467805829466));
#43926=CARTESIAN_POINT('Ctrl Pts',(0.00125595755705645,-0.039778774389881,
-0.0138622743458417));
#43927=CARTESIAN_POINT('Ctrl Pts',(0.00126478613523544,-0.039778774389881,
-0.0138537573167305));
#43928=CARTESIAN_POINT('Ctrl Pts',(0.00127354488019596,-0.039778774389881,
-0.0138451632153568));
#43929=CARTESIAN_POINT('Ctrl Pts',(0.00128222281185596,-0.039778774389881,
-0.0138365023680465));
#43930=CARTESIAN_POINT('Ctrl Pts',(0.00143780054712722,-0.0397787743898809,
-0.0136812309205574));
#43931=CARTESIAN_POINT('Ctrl Pts',(0.00156853257307188,-0.0397787743898809,
-0.013503836767471));
#43932=CARTESIAN_POINT('Ctrl Pts',(0.00166648651957269,-0.0397787743898807,
-0.013308227265951));
#43933=CARTESIAN_POINT('Ctrl Pts',(0.00168292296901946,-0.0397787743898806,
-0.0132754044364695));
#43934=CARTESIAN_POINT('Ctrl Pts',(0.00169842718748885,-0.0397787743898806,
-0.0132420666686444));
#43935=CARTESIAN_POINT('Ctrl Pts',(0.00171294960382052,-0.0397787743898806,
-0.0132082309571952));
#43936=CARTESIAN_POINT('Ctrl Pts',(0.000483041833372184,-0.0397787743898692,
-0.0102334017947949));
#43937=CARTESIAN_POINT('Ctrl Pts',(0.000414177013520476,-0.0397787743898693,
-0.0102065664006364));
#43938=CARTESIAN_POINT('Ctrl Pts',(0.000343834095042283,-0.0397787743898694,
-0.0101837221474513));
#43939=CARTESIAN_POINT('Ctrl Pts',(0.000272408372401186,-0.0397787743898695,
-0.0101647601900402));
#43940=CARTESIAN_POINT('Ctrl Pts',(0.000200790353882954,-0.0397787743898696,
-0.0101457471823058));
#43941=CARTESIAN_POINT('Ctrl Pts',(0.000128082810507698,-0.0397787743898699,
-0.0101306371703763));
#43942=CARTESIAN_POINT('Ctrl Pts',(5.4645348325696E-5,-0.0397787743898706,
-0.0101193622655315));
#43943=CARTESIAN_POINT('Ctrl Pts',(-2.60214829574234E-7,-0.0397787743898712,
-0.0101109325760838));
#43944=CARTESIAN_POINT('Ctrl Pts',(-5.55746772423925E-5,-0.0397787743898709,
-0.0101046474835075));
#43945=CARTESIAN_POINT('Ctrl Pts',(-0.00011115731807598,-0.0397787743898708,
-0.0101004949795128));
#43946=CARTESIAN_POINT('Ctrl Pts',(-0.000133445379702656,-0.0397787743898708,
-0.0100988298685438));
#43947=CARTESIAN_POINT('Ctrl Pts',(-0.000155776632439193,-0.0397787743898707,
-0.0100975078244661));
#43948=CARTESIAN_POINT('Ctrl Pts',(-0.000178142233916201,-0.0397787743898706,
-0.0100965287355665));
#43949=CARTESIAN_POINT('Ctrl Pts',(-0.00019234388482969,-0.0397787743898706,
-0.0100959070362672));
#43950=CARTESIAN_POINT('Ctrl Pts',(-0.000206551772363642,-0.0397787743898706,
-0.0100954240005371));
#43951=CARTESIAN_POINT('Ctrl Pts',(-0.000220756779646141,-0.0397787743898706,
-0.0100950792693289));
#43952=CARTESIAN_POINT('Ctrl Pts',(-0.000425767795136176,-0.0397787743898701,
-0.0100901040029552));
#43953=CARTESIAN_POINT('Ctrl Pts',(-0.000630534063748425,-0.0397787743898698,
-0.0101137246364624));
#43954=CARTESIAN_POINT('Ctrl Pts',(-0.000828216436399461,-0.0397787743898695,
-0.0101651844785696));
#43955=CARTESIAN_POINT('Ctrl Pts',(-0.000847794356858231,-0.0397787743898695,
-0.0101702809203114));
#43956=CARTESIAN_POINT('Ctrl Pts',(-0.00086730325133829,-0.0397787743898694,
-0.010175652348327));
#43957=CARTESIAN_POINT('Ctrl Pts',(-0.00088673662891264,-0.0397787743898694,
-0.0101812993238104));
#43958=CARTESIAN_POINT('Ctrl Pts',(-0.000899127635869771,-0.0397787743898694,
-0.0101848999183151));
#43959=CARTESIAN_POINT('Ctrl Pts',(-0.000911479167813636,-0.0397787743898694,
-0.0101886100052308));
#43960=CARTESIAN_POINT('Ctrl Pts',(-0.000923787881901184,-0.0397787743898694,
-0.0101924287155602));
#43961=CARTESIAN_POINT('Ctrl Pts',(-0.0010006813909627,-0.0397787743898693,
-0.0102162845005941));
#43962=CARTESIAN_POINT('Ctrl Pts',(-0.00107592433438783,-0.0397787743898692,
-0.0102443815824418));
#43963=CARTESIAN_POINT('Ctrl Pts',(-0.001149122989709,-0.0397787743898691,
-0.0102766566890817));
#43964=CARTESIAN_POINT('Ctrl Pts',(-0.00118063222353515,-0.039778774389869,
-0.0102905498935049));
#43965=CARTESIAN_POINT('Ctrl Pts',(-0.00121176282517371,-0.039778774389869,
-0.0103052179143883));
#43966=CARTESIAN_POINT('Ctrl Pts',(-0.00124248380239654,-0.039778774389869,
-0.0103206586458563));
#43967=CARTESIAN_POINT('Ctrl Pts',(-0.00135026660817169,-0.0397787743898688,
-0.0103748315762539));
#43968=CARTESIAN_POINT('Ctrl Pts',(-0.00145301438322215,-0.0397787743898688,
-0.0104384928979925));
#43969=CARTESIAN_POINT('Ctrl Pts',(-0.00155024698053707,-0.0397787743898687,
-0.0105105042446334));
#43970=CARTESIAN_POINT('Ctrl Pts',(-0.00157849804471611,-0.0397787743898687,
-0.0105314272399226));
#43971=CARTESIAN_POINT('Ctrl Pts',(-0.00160628289122325,-0.0397787743898687,
-0.010553056998596));
#43972=CARTESIAN_POINT('Ctrl Pts',(-0.00163358791178077,-0.0397787743898687,
-0.0105753698802968));
#43973=CARTESIAN_POINT('Ctrl Pts',(-0.00164341407028885,-0.0397787743898687,
-0.0105833995359384));
#43974=CARTESIAN_POINT('Ctrl Pts',(-0.00165317745973684,-0.0397787743898687,
-0.0105915172646323));
#43975=CARTESIAN_POINT('Ctrl Pts',(-0.00166286744266842,-0.0397787743898687,
-0.010599713243512));
#43976=CARTESIAN_POINT('Ctrl Pts',(-0.00187591233938246,-0.0397787743898686,
-0.0107799108234484));
#43977=CARTESIAN_POINT('Ctrl Pts',(-0.00205500826442918,-0.0397787743898687,
-0.0109984408165224));
#43978=CARTESIAN_POINT('Ctrl Pts',(-0.00219419613869514,-0.0397787743898689,
-0.011242458169426));
#43979=CARTESIAN_POINT('Ctrl Pts',(-0.00220088488234335,-0.0397787743898689,
-0.0112541845466546));
#43980=CARTESIAN_POINT('Ctrl Pts',(-0.00220748074423558,-0.0397787743898689,
-0.0112659708583141));
#43981=CARTESIAN_POINT('Ctrl Pts',(-0.00221398281530691,-0.0397787743898689,
-0.011277815973893));
#43982=CARTESIAN_POINT('Ctrl Pts',(-0.00222015900819364,-0.0397787743898689,
-0.0112890674225127));
#43983=CARTESIAN_POINT('Ctrl Pts',(-0.0022262457661904,-0.0397787743898689,
-0.0113003631705176));
#43984=CARTESIAN_POINT('Ctrl Pts',(-0.00223224252299715,-0.0397787743898689,
-0.0113117017067491));
#43985=CARTESIAN_POINT('Ctrl Pts',(-0.0023529561855896,-0.0397787743898691,
-0.0115399444521286));
#43986=CARTESIAN_POINT('Ctrl Pts',(-0.00243745467686456,-0.0397787743898694,
-0.0117853097684529));
#43987=CARTESIAN_POINT('Ctrl Pts',(-0.00248078229039228,-0.0397787743898698,
-0.012039045318197));
#43988=CARTESIAN_POINT('Ctrl Pts',(-0.00248852509767497,-0.0397787743898699,
-0.0120843888140066));
#43989=CARTESIAN_POINT('Ctrl Pts',(-0.00249494460435551,-0.0397787743898701,
-0.0121300059194942));
#43990=CARTESIAN_POINT('Ctrl Pts',(-0.00250000000000001,-0.0397787743898723,
-0.0121758532865581));
#43991=CARTESIAN_POINT('Ctrl Pts',(0.000906555879570053,-0.0336884873565647,
-0.0139554885237476));
#43992=CARTESIAN_POINT('Ctrl Pts',(0.00148851471592875,-0.0337405323694969,
-0.0136590408284119));
#43993=CARTESIAN_POINT('Ctrl Pts',(0.00233007966486597,-0.0338446173408443,
-0.0124566928781431));
#43994=CARTESIAN_POINT('Ctrl Pts',(0.00152799326844162,-0.0340007422706073,
-0.0103918577137271));
#43995=CARTESIAN_POINT('Ctrl Pts',(-0.00063191986896287,-0.0341568621458532,
-0.00991565403964754));
#43996=CARTESIAN_POINT('Ctrl Pts',(-0.00223010102783316,-0.0343129820210993,
-0.0114427530396798));
#43997=CARTESIAN_POINT('Ctrl Pts',(-0.00184953643573394,-0.0344691018963453,
-0.0136218346413422));
#43998=CARTESIAN_POINT('Ctrl Pts',(0.000172737121026436,-0.0346252217715913,
-0.0145169013604168));
#43999=CARTESIAN_POINT('Ctrl Pts',(0.00204157869281899,-0.0347813416468374,
-0.013334655467512));
#44000=CARTESIAN_POINT('Ctrl Pts',(0.00209858523606372,-0.0349374615220834,
-0.0111237801770316));
#44001=CARTESIAN_POINT('Ctrl Pts',(0.000293061994614866,-0.0350935813973294,
-0.00984672032610751));
#44002=CARTESIAN_POINT('Ctrl Pts',(-0.00177253570391892,-0.0352497012725754,
-0.0106367143420735));
#44003=CARTESIAN_POINT('Ctrl Pts',(-0.0022650169213336,-0.0354058211478214,
-0.0127927219130861));
#44004=CARTESIAN_POINT('Ctrl Pts',(-0.000747290023119862,-0.0355619410230674,
-0.0144012441562325));
#44005=CARTESIAN_POINT('Ctrl Pts',(0.00143365440835409,-0.0357180608983135,
-0.0140347387897662));
#44006=CARTESIAN_POINT('Ctrl Pts',(0.00234223148318713,-0.0358741807735595,
-0.0120184681222078));
#44007=CARTESIAN_POINT('Ctrl Pts',(0.00117207673424978,-0.0360303006488055,
-0.010141878857636));
#44008=CARTESIAN_POINT('Ctrl Pts',(-0.00103829608658593,-0.0361864205240515,
-0.0100704414314441));
#44009=CARTESIAN_POINT('Ctrl Pts',(-0.0023271810267558,-0.0363425403992976,
-0.0118675581893953));
#44010=CARTESIAN_POINT('Ctrl Pts',(-0.00155069202014295,-0.0364986602745435,
-0.0139382866448643));
#44011=CARTESIAN_POINT('Ctrl Pts',(0.000602036529911888,-0.0366547801497896,
-0.0144448551399557));
#44012=CARTESIAN_POINT('Ctrl Pts',(0.00222045755410605,-0.0368109000250356,
-0.0129376837430793));
#44013=CARTESIAN_POINT('Ctrl Pts',(0.00186822176134942,-0.0369670199002817,
-0.0107543876576293));
#44014=CARTESIAN_POINT('Ctrl Pts',(-0.000142061225288998,-0.0371231397755276,
-0.00983264266723763));
#44015=CARTESIAN_POINT('Ctrl Pts',(-0.00202626513103703,-0.0372792596507737,
-0.0109904978707365));
#44016=CARTESIAN_POINT('Ctrl Pts',(-0.00211215758058384,-0.0374353795260197,
-0.0132003561920008));
#44017=CARTESIAN_POINT('Ctrl Pts',(-0.000323510645583594,-0.0375914994012657,
-0.0145009681811352));
#44018=CARTESIAN_POINT('Ctrl Pts',(0.00175225415004698,-0.0377476192765118,
-0.0137380394695316));
#44019=CARTESIAN_POINT('Ctrl Pts',(0.00227288891551885,-0.0379037391517577,
-0.0115886711349254));
#44020=CARTESIAN_POINT('Ctrl Pts',(0.000776341706463385,-0.0380598590270038,
-0.00996042508615809));
#44021=CARTESIAN_POINT('Ctrl Pts',(-0.00140922355039861,-0.0382159789022498,
-0.0102983761236881));
#44022=CARTESIAN_POINT('Ctrl Pts',(-0.00234407459792171,-0.0383720987774958,
-0.0123025811821577));
#44023=CARTESIAN_POINT('Ctrl Pts',(-0.00119861222885379,-0.0385282186527418,
-0.0141943295796207));
#44024=CARTESIAN_POINT('Ctrl Pts',(0.00101072130964566,-0.0386843385279879,
-0.0142946521179208));
#44025=CARTESIAN_POINT('Ctrl Pts',(0.00232284301417837,-0.0388404584032339,
-0.0125145929042303));
#44026=CARTESIAN_POINT('Ctrl Pts',(0.00157381725247728,-0.0389965782784799,
-0.0104338009448371));
#44027=CARTESIAN_POINT('Ctrl Pts',(-0.000572693408805765,-0.0391526981537259,
-0.00989927497122912));
#44028=CARTESIAN_POINT('Ctrl Pts',(-0.00220955263118552,-0.039308818028972,
-0.0113848409437049));
#44029=CARTESIAN_POINT('Ctrl Pts',(-0.00188811561699103,-0.0394649379042179,
-0.0135731446123589));
#44030=CARTESIAN_POINT('Ctrl Pts',(0.000114518372946742,-0.0396210666742362,
-0.0145200265170436));
#44031=CARTESIAN_POINT('Ctrl Pts',(0.00137369945946738,-0.039725155485839,
-0.0137659946183006));
#44032=CARTESIAN_POINT('Ctrl Pts',(0.00171075374050644,-0.0397772043390267,
-0.0132065165554317));
#44033=CARTESIAN_POINT('Ctrl Pts',(0.00098385440276809,-0.0337868080702585,
-0.0141072311562383));
#44034=CARTESIAN_POINT('Ctrl Pts',(0.00161543462444493,-0.0338388530831906,
-0.0137855065093421));
#44035=CARTESIAN_POINT('Ctrl Pts',(0.00252875657059996,-0.0339429380545382,
-0.0124806389868986));
#44036=CARTESIAN_POINT('Ctrl Pts',(0.00165827936085888,-0.034099062984301,
-0.0102397432922342));
#44037=CARTESIAN_POINT('Ctrl Pts',(-0.000685801238827782,-0.0342551828595471,
-0.0097229355676187));
#44038=CARTESIAN_POINT('Ctrl Pts',(-0.00242025314081233,-0.0344113027347931,
-0.0113802444092502));
#44039=CARTESIAN_POINT('Ctrl Pts',(-0.00200723927381052,-0.0345674226100391,
-0.0137451278942078));
#44040=CARTESIAN_POINT('Ctrl Pts',(0.000187465749076539,-0.0347235424852852,
-0.0147165135000796));
#44041=CARTESIAN_POINT('Ctrl Pts',(0.00221565623343605,-0.0348796623605312,
-0.0134334620598964));
#44042=CARTESIAN_POINT('Ctrl Pts',(0.00227752350474481,-0.0350357822357772,
-0.0110340739609059));
#44043=CARTESIAN_POINT('Ctrl Pts',(0.000318050260533953,-0.0351919021110232,
-0.00964812414220752));
#44044=CARTESIAN_POINT('Ctrl Pts',(-0.00192367298659113,-0.0353480219862693,
-0.0105054779008497));
#44045=CARTESIAN_POINT('Ctrl Pts',(-0.00245814617787837,-0.0355041418615152,
-0.0128453199215624));
#44046=CARTESIAN_POINT('Ctrl Pts',(-0.000811008561038556,-0.0356602617367613,
-0.0145909946521928));
#44047=CARTESIAN_POINT('Ctrl Pts',(0.00155589659004363,-0.0358163816120073,
-0.0141932387867663));
#44048=CARTESIAN_POINT('Ctrl Pts',(0.00254194452759889,-0.0359725014872533,
-0.0120050484962897));
#44049=CARTESIAN_POINT('Ctrl Pts',(0.00127201519659285,-0.0361286213624993,
-0.00996844970327133));
#44050=CARTESIAN_POINT('Ctrl Pts',(-0.00112682758910452,-0.0362847412377453,
-0.00989092108328737));
#44051=CARTESIAN_POINT('Ctrl Pts',(-0.00252561077679837,-0.0364408611129914,
-0.011841271055577));
#44052=CARTESIAN_POINT('Ctrl Pts',(-0.00168291354756704,-0.0365969809882374,
-0.0140885625394916));
#44053=CARTESIAN_POINT('Ctrl Pts',(0.000653369862718166,-0.0367531008634834,
-0.0146383241762873));
#44054=CARTESIAN_POINT('Ctrl Pts',(0.00240978740527609,-0.0369092207387295,
-0.0130026420876706));
#44055=CARTESIAN_POINT('Ctrl Pts',(0.00202751782507054,-0.0370653406139755,
-0.0106331847661483));
#44056=CARTESIAN_POINT('Ctrl Pts',(-0.000154174238028764,-0.0372214604892215,
-0.00963284613566438));
#44057=CARTESIAN_POINT('Ctrl Pts',(-0.00219903694330649,-0.0373775803644675,
-0.0108894271864326));
#44058=CARTESIAN_POINT('Ctrl Pts',(-0.00229225311073265,-0.0375337002397135,
-0.0132877116031647));
#44059=CARTESIAN_POINT('Ctrl Pts',(-0.000351095150528087,-0.0376898201149596,
-0.0146992217600561));
#44060=CARTESIAN_POINT('Ctrl Pts',(0.00190166210284798,-0.0378459399902055,
-0.0138712410598864));
#44061=CARTESIAN_POINT('Ctrl Pts',(0.00246668938664495,-0.0380020598654516,
-0.0115386043776605));
#44062=CARTESIAN_POINT('Ctrl Pts',(0.000842537369366294,-0.0381581797406976,
-0.00977152406857997));
#44063=CARTESIAN_POINT('Ctrl Pts',(-0.00152938260706192,-0.0383142996159437,
-0.0101382908875782));
#44064=CARTESIAN_POINT('Ctrl Pts',(-0.00254394479761788,-0.0384704194911896,
-0.0123133867810167));
#44065=CARTESIAN_POINT('Ctrl Pts',(-0.00130081327047237,-0.0386265393664357,
-0.0143664372677182));
#44066=CARTESIAN_POINT('Ctrl Pts',(0.00109690161729249,-0.0387826592416817,
-0.0144753139219078));
#44067=CARTESIAN_POINT('Ctrl Pts',(0.00252090287862051,-0.0389387791169277,
-0.0125434759248856));
#44068=CARTESIAN_POINT('Ctrl Pts',(0.00170801057926678,-0.0390948989921738,
-0.010285262860883));
#44069=CARTESIAN_POINT('Ctrl Pts',(-0.000621524766853903,-0.0392510188674198,
-0.00970515991921151));
#44070=CARTESIAN_POINT('Ctrl Pts',(-0.00239795266163922,-0.0394071387426657,
-0.0113173943722227));
#44071=CARTESIAN_POINT('Ctrl Pts',(-0.00204910795305066,-0.0395632586179118,
-0.0136922862542543));
#44072=CARTESIAN_POINT('Ctrl Pts',(0.000124282912902093,-0.03971938738793,
-0.014719905126758));
#44073=CARTESIAN_POINT('Ctrl Pts',(0.00149082951391602,-0.0398234761995329,
-0.0139015798363658));
#44074=CARTESIAN_POINT('Ctrl Pts',(0.00185662311345606,-0.0398755250527205,
-0.0132943972370243));
#44075=CARTESIAN_POINT('Ctrl Pts',(0.00106115292596612,-0.0338851287839525,
-0.0142589737887292));
#44076=CARTESIAN_POINT('Ctrl Pts',(0.00174235453296112,-0.0339371737968846,
-0.0139119721902721));
#44077=CARTESIAN_POINT('Ctrl Pts',(0.00272743347633392,-0.0340412587682322,
-0.012504585095654));
#44078=CARTESIAN_POINT('Ctrl Pts',(0.00178856545327616,-0.034197383697995,
-0.0100876288707415));
#44079=CARTESIAN_POINT('Ctrl Pts',(-0.000739682608692693,-0.034353503573241,
-0.00953021709558985));
#44080=CARTESIAN_POINT('Ctrl Pts',(-0.00261040525379151,-0.034509623448487,
-0.0113177357788206));
#44081=CARTESIAN_POINT('Ctrl Pts',(-0.00216494211188709,-0.0346657433237329,
-0.0138684211470736));
#44082=CARTESIAN_POINT('Ctrl Pts',(0.00020219437712664,-0.0348218631989791,
-0.0149161256397424));
#44083=CARTESIAN_POINT('Ctrl Pts',(0.00238973377405311,-0.0349779830742251,
-0.0135322686522809));
#44084=CARTESIAN_POINT('Ctrl Pts',(0.00245646177342591,-0.0351341029494712,
-0.0109443677447801));
#44085=CARTESIAN_POINT('Ctrl Pts',(0.000343038526453036,-0.035290222824717,
-0.00944952795830755));
#44086=CARTESIAN_POINT('Ctrl Pts',(-0.00207481026926333,-0.0354463426999631,
-0.010374241459626));
#44087=CARTESIAN_POINT('Ctrl Pts',(-0.00265127543442315,-0.0356024625752092,
-0.0128979179300387));
#44088=CARTESIAN_POINT('Ctrl Pts',(-0.000874727098957249,-0.0357585824504551,
-0.0147807451481533));
#44089=CARTESIAN_POINT('Ctrl Pts',(0.00167813877173317,-0.0359147023257013,
-0.0143517387837662));
#44090=CARTESIAN_POINT('Ctrl Pts',(0.00274165757201066,-0.0360708222009473,
-0.0119916288703718));
#44091=CARTESIAN_POINT('Ctrl Pts',(0.00137195365893592,-0.0362269420761933,
-0.00979502054890656));
#44092=CARTESIAN_POINT('Ctrl Pts',(-0.0012153590916231,-0.0363830619514392,
-0.00971140073513063));
#44093=CARTESIAN_POINT('Ctrl Pts',(-0.00272404052684096,-0.0365391818266853,
-0.0118149839217589));
#44094=CARTESIAN_POINT('Ctrl Pts',(-0.00181513507499112,-0.0366953017019313,
-0.0142388384341189));
#44095=CARTESIAN_POINT('Ctrl Pts',(0.000704703195524443,-0.0368514215771773,
-0.0148317932126191));
#44096=CARTESIAN_POINT('Ctrl Pts',(0.00259911725644613,-0.0370075414524233,
-0.0130676004322619));
#44097=CARTESIAN_POINT('Ctrl Pts',(0.00218681388879167,-0.0371636613276694,
-0.0105119818746673));
#44098=CARTESIAN_POINT('Ctrl Pts',(-0.000166287250768526,-0.0373197812029154,
-0.00943304960409114));
#44099=CARTESIAN_POINT('Ctrl Pts',(-0.00237180875557593,-0.0374759010781614,
-0.0107883565021288));
#44100=CARTESIAN_POINT('Ctrl Pts',(-0.00247234864088144,-0.0376320209534073,
-0.0133750670143283));
#44101=CARTESIAN_POINT('Ctrl Pts',(-0.000378679655472579,-0.0377881408286535,
-0.0148974753389772));
#44102=CARTESIAN_POINT('Ctrl Pts',(0.00205107005564896,-0.0379442607038995,
-0.0140044426502412));
#44103=CARTESIAN_POINT('Ctrl Pts',(0.00266048985777104,-0.0381003805791455,
-0.0114885376203958));
#44104=CARTESIAN_POINT('Ctrl Pts',(0.000908733032269202,-0.0382565004543916,
-0.00958262305100186));
#44105=CARTESIAN_POINT('Ctrl Pts',(-0.00164954166372522,-0.0384126203296376,
-0.00997820565146808));
#44106=CARTESIAN_POINT('Ctrl Pts',(-0.00274381499731402,-0.0385687402048836,
-0.0123241923798756));
#44107=CARTESIAN_POINT('Ctrl Pts',(-0.00140301431209096,-0.0387248600801295,
-0.0145385449558156));
#44108=CARTESIAN_POINT('Ctrl Pts',(0.00118308192493933,-0.0388809799553756,
-0.0146559757258947));
#44109=CARTESIAN_POINT('Ctrl Pts',(0.00271896274306265,-0.0390370998306216,
-0.0125723589455407));
#44110=CARTESIAN_POINT('Ctrl Pts',(0.00184220390605629,-0.0391932197058677,
-0.0101367247769288));
#44111=CARTESIAN_POINT('Ctrl Pts',(-0.000670356124902047,-0.0393493395811137,
-0.00951104486719392));
#44112=CARTESIAN_POINT('Ctrl Pts',(-0.00258635269209294,-0.0395054594563597,
-0.0112499478007406));
#44113=CARTESIAN_POINT('Ctrl Pts',(-0.00221010028911027,-0.0396615793316057,
-0.0138114278961496));
#44114=CARTESIAN_POINT('Ctrl Pts',(0.000134047452857446,-0.0398177081016239,
-0.0149197837364725));
#44115=CARTESIAN_POINT('Ctrl Pts',(0.00160795956836466,-0.039921796913227,
-0.0140371650544312));
#44116=CARTESIAN_POINT('Ctrl Pts',(0.00200249248640567,-0.0399738457664145,
-0.0133822779186168));
#44117=CARTESIAN_POINT('Ctrl Pts',(0.00113845144916417,-0.0339834494976463,
-0.0144107164212199));
#44118=CARTESIAN_POINT('Ctrl Pts',(0.00186927444147729,-0.0340354945105784,
-0.0140384378712023));
#44119=CARTESIAN_POINT('Ctrl Pts',(0.0029261103820679,-0.0341395794819259,
-0.0125285312044095));
#44120=CARTESIAN_POINT('Ctrl Pts',(0.00191885154569343,-0.0342957044116889,
-0.00993551444924871));
#44121=CARTESIAN_POINT('Ctrl Pts',(-0.000793563978557607,-0.0344518242869349,
-0.009337498623561));
#44122=CARTESIAN_POINT('Ctrl Pts',(-0.00280055736677067,-0.0346079441621809,
-0.011255227148391));
#44123=CARTESIAN_POINT('Ctrl Pts',(-0.00232264494996366,-0.0347640640374269,
-0.0139917143999392));
#44124=CARTESIAN_POINT('Ctrl Pts',(0.000216923005176743,-0.034920183912673,
-0.0151157377794053));
#44125=CARTESIAN_POINT('Ctrl Pts',(0.00256381131467016,-0.0350763037879189,
-0.0136310752446654));
#44126=CARTESIAN_POINT('Ctrl Pts',(0.00263540004210701,-0.035232423663165,
-0.0108546615286545));
#44127=CARTESIAN_POINT('Ctrl Pts',(0.00036802679237212,-0.035388543538411,
-0.00925093177440756));
#44128=CARTESIAN_POINT('Ctrl Pts',(-0.00222594755193554,-0.035544663413657,
-0.0102430050184023));
#44129=CARTESIAN_POINT('Ctrl Pts',(-0.00284440469096792,-0.035700783288903,
-0.0129505159385148));
#44130=CARTESIAN_POINT('Ctrl Pts',(-0.000938445636875939,-0.035856903164149,
-0.0149704956441137));
#44131=CARTESIAN_POINT('Ctrl Pts',(0.00180038095342271,-0.036013023039395,
-0.0145102387807663));
#44132=CARTESIAN_POINT('Ctrl Pts',(0.00294137061642242,-0.0361691429146411,
-0.0119782092444539));
#44133=CARTESIAN_POINT('Ctrl Pts',(0.00147189212127897,-0.0363252627898871,
-0.00962159139454179));
#44134=CARTESIAN_POINT('Ctrl Pts',(-0.00130389059414169,-0.0364813826651332,
-0.00953188038697389));
#44135=CARTESIAN_POINT('Ctrl Pts',(-0.00292247027688355,-0.0366375025403792,
-0.0117886967879408));
#44136=CARTESIAN_POINT('Ctrl Pts',(-0.0019473566024152,-0.0367936224156252,
-0.0143891143287463));
#44137=CARTESIAN_POINT('Ctrl Pts',(0.00075603652833072,-0.0369497422908712,
-0.0150252622489507));
#44138=CARTESIAN_POINT('Ctrl Pts',(0.00278844710761618,-0.0371058621661172,
-0.0131325587768532));
#44139=CARTESIAN_POINT('Ctrl Pts',(0.0023461099525128,-0.0372619820413633,
-0.0103907789831864));
#44140=CARTESIAN_POINT('Ctrl Pts',(-0.00017840026350829,-0.0374181019166092,
-0.00923325307251788));
#44141=CARTESIAN_POINT('Ctrl Pts',(-0.00254458056784538,-0.0375742217918553,
-0.0106872858178249));
#44142=CARTESIAN_POINT('Ctrl Pts',(-0.00265244417103022,-0.0377303416671013,
-0.0134624224254922));
#44143=CARTESIAN_POINT('Ctrl Pts',(-0.000406264160417076,-0.0378864615423473,
-0.0150957289178981));
#44144=CARTESIAN_POINT('Ctrl Pts',(0.00220047800844996,-0.0380425814175933,
-0.014137644240596));
#44145=CARTESIAN_POINT('Ctrl Pts',(0.00285429032889712,-0.0381987012928394,
-0.0114384708631308));
#44146=CARTESIAN_POINT('Ctrl Pts',(0.000974928695172114,-0.0383548211680854,
-0.00939372203342373));
#44147=CARTESIAN_POINT('Ctrl Pts',(-0.00176970072038853,-0.0385109410433314,
-0.00981812041535807));
#44148=CARTESIAN_POINT('Ctrl Pts',(-0.00294368519701017,-0.0386670609185775,
-0.0123349979787346));
#44149=CARTESIAN_POINT('Ctrl Pts',(-0.00150521535370954,-0.0388231807938234,
-0.0147106526439131));
#44150=CARTESIAN_POINT('Ctrl Pts',(0.00126926223258616,-0.0389793006690694,
-0.0148366375298816));
#44151=CARTESIAN_POINT('Ctrl Pts',(0.00291702260750478,-0.0391354205443155,
-0.012601241966196));
#44152=CARTESIAN_POINT('Ctrl Pts',(0.0019763972328458,-0.0392915404195615,
-0.00998818669297467));
#44153=CARTESIAN_POINT('Ctrl Pts',(-0.00071918748295019,-0.0394476602948075,
-0.0093169298151763));
#44154=CARTESIAN_POINT('Ctrl Pts',(-0.00277475272254664,-0.0396037801700536,
-0.0111825012292584));
#44155=CARTESIAN_POINT('Ctrl Pts',(-0.00237109262516989,-0.0397599000452996,
-0.0139305695380448));
#44156=CARTESIAN_POINT('Ctrl Pts',(0.000143811992812799,-0.0399160288153178,
-0.0151196623461868));
#44157=CARTESIAN_POINT('Ctrl Pts',(0.00172508962281328,-0.0400201176269206,
-0.0141727502724965));
#44158=CARTESIAN_POINT('Ctrl Pts',(0.00214836185935528,-0.0400721664801083,
-0.0134701586002094));
#44159=CARTESIAN_POINT('Ctrl Pts',(0.00151144094680255,-0.033978774389881,
-0.0108636057192968));
#44160=CARTESIAN_POINT('Ctrl Pts',(0.00166330063753257,-0.0339787743898811,
-0.0109989552134901));
#44161=CARTESIAN_POINT('Ctrl Pts',(0.00179339272885179,-0.033978774389881,
-0.011157796271544));
#44162=CARTESIAN_POINT('Ctrl Pts',(0.00189962202083712,-0.0339787743898808,
-0.0113327013342186));
#44163=CARTESIAN_POINT('Ctrl Pts',(0.00191122342101952,-0.0339787743898808,
-0.0113518028794524));
#44164=CARTESIAN_POINT('Ctrl Pts',(0.00192253879240254,-0.0339787743898808,
-0.0113710986315245));
#44165=CARTESIAN_POINT('Ctrl Pts',(0.0019335642210336,-0.0339787743898808,
-0.0113905806628577));
#44166=CARTESIAN_POINT('Ctrl Pts',(0.00194056621304015,-0.0339787743898807,
-0.0114029532455691));
#44167=CARTESIAN_POINT('Ctrl Pts',(0.0019474474664082,-0.0339787743898807,
-0.0114153943530156));
#44168=CARTESIAN_POINT('Ctrl Pts',(0.00195420415872564,-0.0339787743898807,
-0.011427895692725));
#44169=CARTESIAN_POINT('Ctrl Pts',(0.00205171004550552,-0.0339787743898806,
-0.0116083026369859));
#44170=CARTESIAN_POINT('Ctrl Pts',(0.00212362567593681,-0.0339787743898803,
-0.0118014738101103));
#44171=CARTESIAN_POINT('Ctrl Pts',(0.00216752041363818,-0.03397877438988,
-0.0120009720848389));
#44172=CARTESIAN_POINT('Ctrl Pts',(0.0021718675886441,-0.03397877438988,
-0.0120207296676162));
#44173=CARTESIAN_POINT('Ctrl Pts',(0.00217593841741397,-0.03397877438988,
-0.0120405505893999));
#44174=CARTESIAN_POINT('Ctrl Pts',(0.00217972945324975,-0.0339787743898799,
-0.0120604293217883));
#44175=CARTESIAN_POINT('Ctrl Pts',(0.00218214673490848,-0.0339787743898799,
-0.0120731046161624));
#44176=CARTESIAN_POINT('Ctrl Pts',(0.00218444853340343,-0.0339787743898799,
-0.0120857944484929));
#44177=CARTESIAN_POINT('Ctrl Pts',(0.00218663410517573,-0.0339787743898797,
-0.012098495444595));
#44178=CARTESIAN_POINT('Ctrl Pts',(0.00220028731583387,-0.0339787743898783,
-0.0121778382406302));
#44179=CARTESIAN_POINT('Ctrl Pts',(0.00220941217430585,-0.0339787743898788,
-0.0122576359088878));
#44180=CARTESIAN_POINT('Ctrl Pts',(0.00221388631338771,-0.0339787743898789,
-0.0123375089230316));
#44181=CARTESIAN_POINT('Ctrl Pts',(0.00221581226193364,-0.033978774389879,
-0.0123718912505887));
#44182=CARTESIAN_POINT('Ctrl Pts',(0.00221687594955819,-0.0339787743898791,
-0.0124062879804758));
#44183=CARTESIAN_POINT('Ctrl Pts',(0.00221706518265614,-0.0339787743898792,
-0.0124406705429053));
#44184=CARTESIAN_POINT('Ctrl Pts',(0.00221792199649984,-0.0339787743898795,
-0.0125963486763256));
#44185=CARTESIAN_POINT('Ctrl Pts',(0.00220091840700706,-0.0339787743898797,
-0.0127517267421406));
#44186=CARTESIAN_POINT('Ctrl Pts',(0.00216767342000132,-0.03397877438988,
-0.0129047836695825));
#44187=CARTESIAN_POINT('Ctrl Pts',(0.00216497993523347,-0.03397877438988,
-0.0129171842309847));
#44188=CARTESIAN_POINT('Ctrl Pts',(0.00216217948073034,-0.03397877438988,
-0.0129295688496655));
#44189=CARTESIAN_POINT('Ctrl Pts',(0.00215927597939003,-0.03397877438988,
-0.0129419235881118));
#44190=CARTESIAN_POINT('Ctrl Pts',(0.00210292817318756,-0.0339787743898804,
-0.0131816901065538));
#44191=CARTESIAN_POINT('Ctrl Pts',(0.00200786407849481,-0.0339787743898806,
-0.0134114392628006));
#44192=CARTESIAN_POINT('Ctrl Pts',(0.00188036716095463,-0.0339787743898808,
-0.0136235328573169));
#44193=CARTESIAN_POINT('Ctrl Pts',(0.00186342196383062,-0.0339787743898808,
-0.0136517215213031));
#44194=CARTESIAN_POINT('Ctrl Pts',(0.00184589784857195,-0.0339787743898808,
-0.0136795980104251));
#44195=CARTESIAN_POINT('Ctrl Pts',(0.00182780425197144,-0.0339787743898809,
-0.0137071434861153));
#44196=CARTESIAN_POINT('Ctrl Pts',(0.00182039269394275,-0.0339787743898809,
-0.013718426753672));
#44197=CARTESIAN_POINT('Ctrl Pts',(0.00181288556877312,-0.0339787743898808,
-0.0137296544738017));
#44198=CARTESIAN_POINT('Ctrl Pts',(0.00180528347101283,-0.0339787743898809,
-0.0137408253232928));
#44199=CARTESIAN_POINT('Ctrl Pts',(0.00179806238775325,-0.0339787743898809,
-0.0137514362936854));
#44200=CARTESIAN_POINT('Ctrl Pts',(0.00179076123317478,-0.0339787743898809,
-0.0137619876892948));
#44201=CARTESIAN_POINT('Ctrl Pts',(0.00178338109605654,-0.0339787743898809,
-0.0137724783202789));
#44202=CARTESIAN_POINT('Ctrl Pts',(0.0016348184319285,-0.033978774389881,
-0.0139836554383211));
#44203=CARTESIAN_POINT('Ctrl Pts',(0.00145455809974202,-0.033978774389881,
-0.0141703380238125));
#44204=CARTESIAN_POINT('Ctrl Pts',(0.00124814854542299,-0.0339787743898809,
-0.0143241368117442));
#44205=CARTESIAN_POINT('Ctrl Pts',(0.0012112623088025,-0.0339787743898809,
-0.0143516212879464));
#44206=CARTESIAN_POINT('Ctrl Pts',(0.00117353151163338,-0.0339787743898809,
-0.0143780508975888));
#44207=CARTESIAN_POINT('Ctrl Pts',(0.00113497624935288,-0.0339787743898726,
-0.014403369597027));
#44208=CARTESIAN_POINT('Origin',(2.24345254752611E-19,-0.0339787743898723,
-0.0121758532865581));
#44209=CARTESIAN_POINT('Ctrl Pts',(-0.000786711117161725,-0.0339787743898715,
-0.0145488441458292));
#44210=CARTESIAN_POINT('Ctrl Pts',(-0.000860123002178482,-0.0339787741780464,
-0.0145142886963759));
#44211=CARTESIAN_POINT('Ctrl Pts',(-0.000931752987587147,-0.033978774389869,
-0.0144761052423907));
#44212=CARTESIAN_POINT('Ctrl Pts',(-0.00100138356020524,-0.0339787743898689,
-0.0144345282803354));
#44213=CARTESIAN_POINT('Ctrl Pts',(-0.00112888556271287,-0.0339787743898688,
-0.0143583958327494));
#44214=CARTESIAN_POINT('Ctrl Pts',(-0.00124970686175793,-0.0339787743898688,
-0.0142708955021727));
#44215=CARTESIAN_POINT('Ctrl Pts',(-0.00136225039894955,-0.0339787743898687,
-0.0141732333563242));
#44216=CARTESIAN_POINT('Ctrl Pts',(-0.00139891908765987,-0.0339787743898687,
-0.0141414132899369));
#44217=CARTESIAN_POINT('Ctrl Pts',(-0.00143473026633101,-0.0339787743898687,
-0.0141084886236575));
#44218=CARTESIAN_POINT('Ctrl Pts',(-0.00146953555976837,-0.0339787743898687,
-0.0140745793427416));
#44219=CARTESIAN_POINT('Ctrl Pts',(-0.00162825693636651,-0.0339787743898687,
-0.0139199440210739));
#44220=CARTESIAN_POINT('Ctrl Pts',(-0.00176567645263645,-0.0339787743898687,
-0.0137455293399189));
#44221=CARTESIAN_POINT('Ctrl Pts',(-0.00187606559832088,-0.0339787743898689,
-0.0135553722231497));
#44222=CARTESIAN_POINT('Ctrl Pts',(-0.00189080530467026,-0.0339787743898689,
-0.0135299815015887));
#44223=CARTESIAN_POINT('Ctrl Pts',(-0.00190505934940457,-0.0339787743898689,
-0.0135043091584398));
#44224=CARTESIAN_POINT('Ctrl Pts',(-0.00191881042213725,-0.0339787743898689,
-0.0134783642158126));
#44225=CARTESIAN_POINT('Ctrl Pts',(-0.00192514106849106,-0.033978774389869,
-0.0134664198199363));
#44226=CARTESIAN_POINT('Ctrl Pts',(-0.00193136505545212,-0.033978774389869,
-0.0134544175408938));
#44227=CARTESIAN_POINT('Ctrl Pts',(-0.00193747420805989,-0.033978774389869,
-0.0134423714900749));
#44228=CARTESIAN_POINT('Ctrl Pts',(-0.00197328449032473,-0.0339787743898691,
-0.0133717606365416));
#44229=CARTESIAN_POINT('Ctrl Pts',(-0.00200521312322471,-0.0339787743898691,
-0.0132995351063943));
#44230=CARTESIAN_POINT('Ctrl Pts',(-0.00203300009904627,-0.0339787743898692,
-0.0132258888697933));
#44231=CARTESIAN_POINT('Ctrl Pts',(-0.00204740119244997,-0.0339787743898693,
-0.013187720400546));
#44232=CARTESIAN_POINT('Ctrl Pts',(-0.00206068903433681,-0.0339787743898693,
-0.0131491701053409));
#44233=CARTESIAN_POINT('Ctrl Pts',(-0.00207282194711271,-0.0339787743898694,
-0.0131102640679554));
#44234=CARTESIAN_POINT('Ctrl Pts',(-0.00211984913524711,-0.0339787743898696,
-0.01295946420864));
#44235=CARTESIAN_POINT('Ctrl Pts',(-0.00214958198481788,-0.0339787743898699,
-0.0128033026699766));
#44236=CARTESIAN_POINT('Ctrl Pts',(-0.00216217348592332,-0.0339787743898701,
-0.0126446198177156));
#44237=CARTESIAN_POINT('Ctrl Pts',(-0.00216315171282087,-0.0339787743898702,
-0.0126322918329138));
#44238=CARTESIAN_POINT('Ctrl Pts',(-0.00216402592998013,-0.0339787743898702,
-0.0126199504008421));
#44239=CARTESIAN_POINT('Ctrl Pts',(-0.00216479558205437,-0.0339787743898702,
-0.0126076087164675));
#44240=CARTESIAN_POINT('Ctrl Pts',(-0.00216967912507767,-0.0339787743898704,
-0.0125292991157523));
#44241=CARTESIAN_POINT('Ctrl Pts',(-0.00217036796979726,-0.0339787743898705,
-0.0124508477717779));
#44242=CARTESIAN_POINT('Ctrl Pts',(-0.00216693899131665,-0.0339787743898707,
-0.0123725957115567));
#44243=CARTESIAN_POINT('Ctrl Pts',(-0.00216352186151759,-0.0339787743898708,
-0.0122946140478242));
#44244=CARTESIAN_POINT('Ctrl Pts',(-0.00215601492434311,-0.0339787743898712,
-0.0122168292977697));
#44245=CARTESIAN_POINT('Ctrl Pts',(-0.00214444540087901,-0.0339787743898705,
-0.0121395948000181));
#44246=CARTESIAN_POINT('Ctrl Pts',(-0.00212839776258705,-0.0339787743898696,
-0.0120324658169251));
#44247=CARTESIAN_POINT('Ctrl Pts',(-0.00210453912761219,-0.0339787743898695,
-0.0119263875876493));
#44248=CARTESIAN_POINT('Ctrl Pts',(-0.00207280590838327,-0.0339787743898694,
-0.0118224055122139));
#44249=CARTESIAN_POINT('Ctrl Pts',(-0.0020692252405201,-0.0339787743898694,
-0.01181067253066));
#44250=CARTESIAN_POINT('Ctrl Pts',(-0.00206554419682896,-0.0339787743898694,
-0.0117989667807872));
#44251=CARTESIAN_POINT('Ctrl Pts',(-0.00206176699337699,-0.0339787743898693,
-0.0117873027340864));
#44252=CARTESIAN_POINT('Ctrl Pts',(-0.00199404940249818,-0.033978774389869,
-0.0115781900525698));
#44253=CARTESIAN_POINT('Ctrl Pts',(-0.00189534055859523,-0.0339787743898688,
-0.0113811715559088));
#44254=CARTESIAN_POINT('Ctrl Pts',(-0.00176552088862998,-0.0339787743898688,
-0.0112050888723163));
#44255=CARTESIAN_POINT('Ctrl Pts',(-0.00174373775123362,-0.0339787743898687,
-0.0111755430162003));
#44256=CARTESIAN_POINT('Ctrl Pts',(-0.00172107260431907,-0.0339787743898687,
-0.0111465939879031));
#44257=CARTESIAN_POINT('Ctrl Pts',(-0.00169751808662202,-0.0339787743898689,
-0.0111182936685626));
#44258=CARTESIAN_POINT('Ctrl Pts',(-0.00212815972946482,-0.0336854482808955,
-0.0108489132294999));
#44259=CARTESIAN_POINT('Ctrl Pts',(-0.00256222339942132,-0.033737507795067,
-0.0115450254415221));
#44260=CARTESIAN_POINT('Ctrl Pts',(-0.00268821701388861,-0.0338416072676536,
-0.0133839745614382));
#44261=CARTESIAN_POINT('Ctrl Pts',(-0.000486973306187236,-0.0339977466986558,
-0.0150849424241983));
#44262=CARTESIAN_POINT('Ctrl Pts',(0.00214464703375922,-0.0341538665739017,
-0.0141970646480211));
#44263=CARTESIAN_POINT('Ctrl Pts',(0.00287363000161765,-0.0343099864491478,
-0.0115187757733854));
#44264=CARTESIAN_POINT('Ctrl Pts',(0.00105188768346137,-0.0344661063243938,
-0.00942187655811136));
#44265=CARTESIAN_POINT('Ctrl Pts',(-0.00170320879371006,-0.0346222261996398,
-0.0097700531871246));
#44266=CARTESIAN_POINT('Ctrl Pts',(-0.00294680945920505,-0.0347783460748859,
-0.012252897597106));
#44267=CARTESIAN_POINT('Ctrl Pts',(-0.0015750623770788,-0.0349344659501319,
-0.0146676160102062));
#44268=CARTESIAN_POINT('Ctrl Pts',(0.00119452509052153,-0.0350905858253779,
-0.0148707633163185));
#44269=CARTESIAN_POINT('Ctrl Pts',(0.00290398577660606,-0.0352467057006239,
-0.0126822455683436));
#44270=CARTESIAN_POINT('Ctrl Pts',(0.00203615063089732,-0.0354028255758699,
-0.0100442688229747));
#44271=CARTESIAN_POINT('Ctrl Pts',(-0.000638764814960264,-0.0355589454511159,
-0.00929809254628702));
#44272=CARTESIAN_POINT('Ctrl Pts',(-0.00274677837741386,-0.035715065326362,
-0.0111059200285361));
#44273=CARTESIAN_POINT('Ctrl Pts',(-0.00241702425108935,-0.035871185201608,
-0.0138633186690574));
#44274=CARTESIAN_POINT('Ctrl Pts',(5.78390342861788E-5,-0.036027305076854,
-0.0151230886392878));
#44275=CARTESIAN_POINT('Ctrl Pts',(0.00248137045250796,-0.0361834249521,
-0.0137671877677982));
#44276=CARTESIAN_POINT('Ctrl Pts',(0.0027026847262315,-0.0363395448273461,
-0.0109989763542873));
#44277=CARTESIAN_POINT('Ctrl Pts',(0.000525365592294934,-0.036495664702592,
-0.00927524394755182));
#44278=CARTESIAN_POINT('Ctrl Pts',(-0.00211821567918175,-0.0366517845778381,
-0.0101258029520302));
#44279=CARTESIAN_POINT('Ctrl Pts',(-0.00288187993770758,-0.0368079044530841,
-0.0127957823649758));
#44280=CARTESIAN_POINT('Ctrl Pts',(-0.00108787485474889,-0.0369640243283302,
-0.0149155744116917));
#44281=CARTESIAN_POINT('Ctrl Pts',(0.00167161934314252,-0.0371201442035761,
-0.0146038633389977));
#44282=CARTESIAN_POINT('Ctrl Pts',(0.00294755115440384,-0.0372762640788222,
-0.0121372923486029));
#44283=CARTESIAN_POINT('Ctrl Pts',(0.00160752995028988,-0.0374323839540682,
-0.00970494474167266));
#44284=CARTESIAN_POINT('Ctrl Pts',(-0.00115917356836235,-0.0375885038293142,
-0.0094655281610616));
#44285=CARTESIAN_POINT('Ctrl Pts',(-0.00289711209160976,-0.0377446237045603,
-0.0116315278692769));
#44286=CARTESIAN_POINT('Ctrl Pts',(-0.0020638591878221,-0.0379007435798062,
-0.0142806128024932));
#44287=CARTESIAN_POINT('Ctrl Pts',(0.000601062435999465,-0.0380568634550523,
-0.0150617302182937));
#44288=CARTESIAN_POINT('Ctrl Pts',(0.00273255420357332,-0.0382129833302983,
-0.0132816173022125));
#44289=CARTESIAN_POINT('Ctrl Pts',(0.0024388779838377,-0.0383691032055443,
-0.0105201647771034));
#44290=CARTESIAN_POINT('Ctrl Pts',(-1.92546192460681E-5,-0.0385252230807903,
-0.00922808595817392));
#44291=CARTESIAN_POINT('Ctrl Pts',(-0.00246039170159155,-0.0386813429560364,
-0.0105522478882585));
#44292=CARTESIAN_POINT('Ctrl Pts',(-0.00271775238336546,-0.0388374628312823,
-0.0133171754567261));
#44293=CARTESIAN_POINT('Ctrl Pts',(-0.000563448104565397,-0.0389935827065284,
-0.0150695329082345));
#44294=CARTESIAN_POINT('Ctrl Pts',(0.00209157012908443,-0.0391497025817744,
-0.0142530712913992));
#44295=CARTESIAN_POINT('Ctrl Pts',(0.00288906432226327,-0.0393058224570205,
-0.0115943779139539));
#44296=CARTESIAN_POINT('Ctrl Pts',(0.00112494460107805,-0.0394619423322664,
-0.00944923592136359));
#44297=CARTESIAN_POINT('Ctrl Pts',(-0.00164299188658567,-0.0396180915523031,
-0.00972899208793168));
#44298=CARTESIAN_POINT('Ctrl Pts',(-0.00250844206789525,-0.0397222008139244,
-0.011356728213131));
#44299=CARTESIAN_POINT('Ctrl Pts',(-0.00250795369641337,-0.0397742701171305,
-0.012177240533185));
#44300=CARTESIAN_POINT('Ctrl Pts',(-0.0019834686101001,-0.0337838939496779,
-0.0109391303497317));
#44301=CARTESIAN_POINT('Ctrl Pts',(-0.00238802079301359,-0.0338359534638493,
-0.0115879146973241));
#44302=CARTESIAN_POINT('Ctrl Pts',(-0.00250544824731082,-0.0339400529364361,
-0.0133018357928247));
#44303=CARTESIAN_POINT('Ctrl Pts',(-0.000453864554152591,-0.0340961923674382,
-0.0148871568173055));
#44304=CARTESIAN_POINT('Ctrl Pts',(0.00199883496163867,-0.0342523122426843,
-0.01405964482454));
#44305=CARTESIAN_POINT('Ctrl Pts',(0.00267825522038416,-0.0344084321179303,
-0.0115634497137735));
#44306=CARTESIAN_POINT('Ctrl Pts',(0.000980371056086661,-0.0345645519931763,
-0.00960911625164863));
#44307=CARTESIAN_POINT('Ctrl Pts',(-0.0015874095971264,-0.0347206718684224,
-0.00993362075422743));
#44308=CARTESIAN_POINT('Ctrl Pts',(-0.00274645929126248,-0.0348767917436684,
-0.0122476594435127));
#44309=CARTESIAN_POINT('Ctrl Pts',(-0.0014679757071952,-0.0350329116189144,
-0.0144982039436755));
#44310=CARTESIAN_POINT('Ctrl Pts',(0.00111331071076243,-0.0351890314941604,
-0.0146875394993302));
#44311=CARTESIAN_POINT('Ctrl Pts',(0.00270654714132937,-0.0353451513694065,
-0.0126478165426109));
#44312=CARTESIAN_POINT('Ctrl Pts',(0.00189771510376056,-0.0355012712446524,
-0.0101891927860523));
#44313=CARTESIAN_POINT('Ctrl Pts',(-0.000595335933750003,-0.0356573911198985,
-0.00949374817166546));
#44314=CARTESIAN_POINT('Ctrl Pts',(-0.00256002809144039,-0.0358135109951445,
-0.0111786635536604));
#44315=CARTESIAN_POINT('Ctrl Pts',(-0.00225269356689315,-0.0359696308703904,
-0.013748589848799));
#44316=CARTESIAN_POINT('Ctrl Pts',(5.39066252202786E-5,-0.0361257507456365,
-0.0149227095153369));
#44317=CARTESIAN_POINT('Ctrl Pts',(0.0023126649444763,-0.0362818706208825,
-0.013658994776367));
#44318=CARTESIAN_POINT('Ctrl Pts',(0.00251893231661951,-0.0364379904961286,
-0.0110789908561722));
#44319=CARTESIAN_POINT('Ctrl Pts',(0.000489646593118128,-0.0365941103713746,
-0.00947245302274003));
#44320=CARTESIAN_POINT('Ctrl Pts',(-0.00197420064429818,-0.0367502302466206,
-0.0102651835039456));
#44321=CARTESIAN_POINT('Ctrl Pts',(-0.00268594425285817,-0.0369063501218667,
-0.0127536341037145));
#44322=CARTESIAN_POINT('Ctrl Pts',(-0.00101391150120779,-0.0370624699971127,
-0.0147293039401408));
#44323=CARTESIAN_POINT('Ctrl Pts',(0.00155796787677828,-0.0372185898723587,
-0.0144387857428698));
#44324=CARTESIAN_POINT('Ctrl Pts',(0.00274715055946227,-0.0373747097476047,
-0.0121399140621891));
#44325=CARTESIAN_POINT('Ctrl Pts',(0.00149823584764362,-0.0375308296228507,
-0.00987293895670145));
#44326=CARTESIAN_POINT('Ctrl Pts',(-0.00108036269772037,-0.0376869494980968,
-0.00964980003258555));
#44327=CARTESIAN_POINT('Ctrl Pts',(-0.00270014079022842,-0.0378430693733427,
-0.0116685359250327));
#44328=CARTESIAN_POINT('Ctrl Pts',(-0.00192353978793748,-0.0379991892485887,
-0.0141375126365903));
#44329=CARTESIAN_POINT('Ctrl Pts',(0.000560196895942137,-0.0381553091238348,
-0.0148655227824418));
#44330=CARTESIAN_POINT('Ctrl Pts',(0.00254677100273285,-0.0383114289990809,
-0.0132064376853053));
#44331=CARTESIAN_POINT('Ctrl Pts',(0.00227306148961988,-0.0384675488743268,
-0.0106327331245048));
#44332=CARTESIAN_POINT('Ctrl Pts',(-1.79455199462971E-5,-0.0386236687495729,
-0.00942850125053447));
#44333=CARTESIAN_POINT('Ctrl Pts',(-0.00229311251457843,-0.0387797886248189,
-0.0106626349420281));
#44334=CARTESIAN_POINT('Ctrl Pts',(-0.00253297554116661,-0.0389359085000649,
-0.0132395782820071));
#44335=CARTESIAN_POINT('Ctrl Pts',(-0.000525139919411454,-0.0390920283753109,
-0.0148727949765153));
#44336=CARTESIAN_POINT('Ctrl Pts',(0.0019493666943436,-0.039248148250557,
-0.0141118436409913));
#44337=CARTESIAN_POINT('Ctrl Pts',(0.00269264017941473,-0.0394042681258029,
-0.0116339117522181));
#44338=CARTESIAN_POINT('Ctrl Pts',(0.00104846091834516,-0.039560388001049,
-0.00963461548342703));
#44339=CARTESIAN_POINT('Ctrl Pts',(-0.00153128676789282,-0.0397165372210856,
-0.00989535135169256));
#44340=CARTESIAN_POINT('Ctrl Pts',(-0.00233789599203442,-0.039820646482707,
-0.0114124195797767));
#44341=CARTESIAN_POINT('Ctrl Pts',(-0.00233744082436491,-0.039872715785913,
-0.0121771462158908));
#44342=CARTESIAN_POINT('Ctrl Pts',(-0.00183877749073539,-0.0338823396184605,
-0.0110293474699636));
#44343=CARTESIAN_POINT('Ctrl Pts',(-0.00221381818660586,-0.0339343991326318,
-0.0116308039531261));
#44344=CARTESIAN_POINT('Ctrl Pts',(-0.00232267948073303,-0.0340384986052186,
-0.0132196970242115));
#44345=CARTESIAN_POINT('Ctrl Pts',(-0.000420755802117943,-0.0341946380362207,
-0.0146893712104127));
#44346=CARTESIAN_POINT('Ctrl Pts',(0.00185302288951808,-0.0343507579114667,
-0.0139222250010588));
#44347=CARTESIAN_POINT('Ctrl Pts',(0.00248288043915068,-0.0345068777867127,
-0.0116081236541615));
#44348=CARTESIAN_POINT('Ctrl Pts',(0.000908854428711957,-0.0346629976619587,
-0.00979635594518588));
#44349=CARTESIAN_POINT('Ctrl Pts',(-0.00147161040054275,-0.0348191175372048,
-0.0100971883213302));
#44350=CARTESIAN_POINT('Ctrl Pts',(-0.00254610912331991,-0.0349752374124508,
-0.0122424212899195));
#44351=CARTESIAN_POINT('Ctrl Pts',(-0.00136088903731159,-0.0351313572876969,
-0.014328791877145));
#44352=CARTESIAN_POINT('Ctrl Pts',(0.00103209633100332,-0.0352874771629428,
-0.014504315682342));
#44353=CARTESIAN_POINT('Ctrl Pts',(0.00250910850605269,-0.0354435970381888,
-0.0126133875168781));
#44354=CARTESIAN_POINT('Ctrl Pts',(0.00175927957662378,-0.0355997169134349,
-0.0103341167491299));
#44355=CARTESIAN_POINT('Ctrl Pts',(-0.000551907052539744,-0.0357558367886809,
-0.00968940379704389));
#44356=CARTESIAN_POINT('Ctrl Pts',(-0.00237327780546691,-0.035911956663927,
-0.0112514070787846));
#44357=CARTESIAN_POINT('Ctrl Pts',(-0.00208836288269695,-0.036068076539173,
-0.0136338610285404));
#44358=CARTESIAN_POINT('Ctrl Pts',(4.99742161543771E-5,-0.036224196414419,
-0.014722330391386));
#44359=CARTESIAN_POINT('Ctrl Pts',(0.00214395943644463,-0.036380316289665,
-0.0135508017849357));
#44360=CARTESIAN_POINT('Ctrl Pts',(0.00233517990700753,-0.036536436164911,
-0.0111590053580572));
#44361=CARTESIAN_POINT('Ctrl Pts',(0.000453927593941321,-0.036692556040157,
-0.00966966209792823));
#44362=CARTESIAN_POINT('Ctrl Pts',(-0.00183018560941461,-0.036848675915403,
-0.0104045640558609));
#44363=CARTESIAN_POINT('Ctrl Pts',(-0.00249000856800876,-0.0370047957906491,
-0.0127114858424534));
#44364=CARTESIAN_POINT('Ctrl Pts',(-0.000939948147666684,-0.0371609156658951,
-0.0145430334685901));
#44365=CARTESIAN_POINT('Ctrl Pts',(0.00144431641041405,-0.0373170355411411,
-0.0142737081467419));
#44366=CARTESIAN_POINT('Ctrl Pts',(0.00254674996452071,-0.0374731554163872,
-0.0121425357757755));
#44367=CARTESIAN_POINT('Ctrl Pts',(0.00138894174499737,-0.0376292752916331,
-0.0100409331717302));
#44368=CARTESIAN_POINT('Ctrl Pts',(-0.00100155182707838,-0.0377853951668792,
-0.00983407190410951));
#44369=CARTESIAN_POINT('Ctrl Pts',(-0.00250316948884707,-0.0379415150421252,
-0.0117055439807884));
#44370=CARTESIAN_POINT('Ctrl Pts',(-0.00178322038805286,-0.0380976349173713,
-0.0139944124706875));
#44371=CARTESIAN_POINT('Ctrl Pts',(0.000519331355884811,-0.0382537547926173,
-0.0146693153465899));
#44372=CARTESIAN_POINT('Ctrl Pts',(0.00236098780189238,-0.0384098746678633,
-0.0131312580683982));
#44373=CARTESIAN_POINT('Ctrl Pts',(0.00210724499540203,-0.0385659945431093,
-0.0107453014719063));
#44374=CARTESIAN_POINT('Ctrl Pts',(-1.66364206465234E-5,-0.0387221144183553,
-0.00962891654289501));
#44375=CARTESIAN_POINT('Ctrl Pts',(-0.00212583332756533,-0.0388782342936013,
-0.0107730219957976));
#44376=CARTESIAN_POINT('Ctrl Pts',(-0.00234819869896776,-0.0390343541688473,
-0.013161981107288));
#44377=CARTESIAN_POINT('Ctrl Pts',(-0.000486831734257513,-0.0391904740440934,
-0.0146760570447959));
#44378=CARTESIAN_POINT('Ctrl Pts',(0.00180716325960277,-0.0393465939193394,
-0.0139706159905834));
#44379=CARTESIAN_POINT('Ctrl Pts',(0.00249621603656618,-0.0395027137945854,
-0.0116734455904824));
#44380=CARTESIAN_POINT('Ctrl Pts',(0.000971977235612279,-0.0396588336698314,
-0.00981999504549048));
#44381=CARTESIAN_POINT('Ctrl Pts',(-0.00141958164919996,-0.039814982889868,
-0.0100617106154535));
#44382=CARTESIAN_POINT('Ctrl Pts',(-0.00216734991617357,-0.0399190921514895,
-0.0114681109464222));
#44383=CARTESIAN_POINT('Ctrl Pts',(-0.00216692795231646,-0.0399711614546955,
-0.0121770518985966));
#44384=CARTESIAN_POINT('Ctrl Pts',(-0.00169408637137068,-0.033980785287243,
-0.0111195645901954));
#44385=CARTESIAN_POINT('Ctrl Pts',(-0.00203961558019815,-0.0340328448014143,
-0.0116736932089283));
#44386=CARTESIAN_POINT('Ctrl Pts',(-0.00213991071415524,-0.0341369442740011,
-0.0131375582555982));
#44387=CARTESIAN_POINT('Ctrl Pts',(-0.000387647050083297,-0.0342930837050033,
-0.01449158560352));
#44388=CARTESIAN_POINT('Ctrl Pts',(0.00170721081739751,-0.0344492035802493,
-0.0137848051775777));
#44389=CARTESIAN_POINT('Ctrl Pts',(0.00228750565791722,-0.0346053234554953,
-0.0116527975945495));
#44390=CARTESIAN_POINT('Ctrl Pts',(0.000837337801337254,-0.0347614433307413,
-0.00998359563872313));
#44391=CARTESIAN_POINT('Ctrl Pts',(-0.0013558112039591,-0.0349175632059874,
-0.0102607558884331));
#44392=CARTESIAN_POINT('Ctrl Pts',(-0.00234575895537733,-0.0350736830812333,
-0.0122371831363263));
#44393=CARTESIAN_POINT('Ctrl Pts',(-0.00125380236742799,-0.0352298029564794,
-0.0141593798106144));
#44394=CARTESIAN_POINT('Ctrl Pts',(0.000950881951244222,-0.0353859228317254,
-0.0143210918653538));
#44395=CARTESIAN_POINT('Ctrl Pts',(0.00231166987077602,-0.0355420427069714,
-0.0125789584911453));
#44396=CARTESIAN_POINT('Ctrl Pts',(0.00162084404948703,-0.0356981625822174,
-0.0104790407122077));
#44397=CARTESIAN_POINT('Ctrl Pts',(-0.000508478171329484,-0.0358542824574634,
-0.00988505942242233));
#44398=CARTESIAN_POINT('Ctrl Pts',(-0.00218652751949343,-0.0360104023327094,
-0.0113241506039089));
#44399=CARTESIAN_POINT('Ctrl Pts',(-0.00192403219850073,-0.0361665222079555,
-0.013519132208282));
#44400=CARTESIAN_POINT('Ctrl Pts',(4.60418070884753E-5,-0.0363226420832015,
-0.0145219512674351));
#44401=CARTESIAN_POINT('Ctrl Pts',(0.00197525392841297,-0.0364787619584476,
-0.0134426087935045));
#44402=CARTESIAN_POINT('Ctrl Pts',(0.00215142749739555,-0.0366348818336936,
-0.0112390198599422));
#44403=CARTESIAN_POINT('Ctrl Pts',(0.000418208594764515,-0.0367910017089396,
-0.00986687117311645));
#44404=CARTESIAN_POINT('Ctrl Pts',(-0.00168617057453104,-0.0369471215841856,
-0.0105439446077764));
#44405=CARTESIAN_POINT('Ctrl Pts',(-0.00229407288315936,-0.0371032414594316,
-0.0126693375811922));
#44406=CARTESIAN_POINT('Ctrl Pts',(-0.000865984794125582,-0.0372593613346777,
-0.0143567629970394));
#44407=CARTESIAN_POINT('Ctrl Pts',(0.00133066494404982,-0.0374154812099236,
-0.014108630550614));
#44408=CARTESIAN_POINT('Ctrl Pts',(0.00234634936957914,-0.0375716010851697,
-0.0121451574893616));
#44409=CARTESIAN_POINT('Ctrl Pts',(0.00127964764235112,-0.0377277209604157,
-0.010208927386759));
#44410=CARTESIAN_POINT('Ctrl Pts',(-0.000922740956436404,-0.0378838408356617,
-0.0100183437756335));
#44411=CARTESIAN_POINT('Ctrl Pts',(-0.00230619818746574,-0.0380399607109077,
-0.0117425520365441));
#44412=CARTESIAN_POINT('Ctrl Pts',(-0.00164290098816823,-0.0381960805861538,
-0.0138513123047845));
#44413=CARTESIAN_POINT('Ctrl Pts',(0.000478465815827482,-0.0383522004613998,
-0.014473107910738));
#44414=CARTESIAN_POINT('Ctrl Pts',(0.0021752046010519,-0.0385083203366458,
-0.0130560784514912));
#44415=CARTESIAN_POINT('Ctrl Pts',(0.0019414285011842,-0.0386644402118919,
-0.0108578698193078));
#44416=CARTESIAN_POINT('Ctrl Pts',(-1.53273213467499E-5,-0.0388205600871378,
-0.00982933183525555));
#44417=CARTESIAN_POINT('Ctrl Pts',(-0.00195855414055221,-0.0389766799623838,
-0.0108834090495671));
#44418=CARTESIAN_POINT('Ctrl Pts',(-0.00216342185676891,-0.0391327998376299,
-0.0130843839325688));
#44419=CARTESIAN_POINT('Ctrl Pts',(-0.000448523549103574,-0.0392889197128759,
-0.0144793191130766));
#44420=CARTESIAN_POINT('Ctrl Pts',(0.00166495982486194,-0.0394450395881219,
-0.0138293883401754));
#44421=CARTESIAN_POINT('Ctrl Pts',(0.00229979189371764,-0.039601159463368,
-0.0117129794287466));
#44422=CARTESIAN_POINT('Ctrl Pts',(0.000895493552879401,-0.039757279338614,
-0.010005374607554));
#44423=CARTESIAN_POINT('Ctrl Pts',(-0.00130787653050712,-0.0399134285586506,
-0.0102280698792143));
#44424=CARTESIAN_POINT('Ctrl Pts',(-0.00199680384031273,-0.0400175378202719,
-0.0115238023130677));
#44425=CARTESIAN_POINT('Ctrl Pts',(-0.001996415080268,-0.040069607123478,
-0.0121769575813024));
#44426=CARTESIAN_POINT('Origin',(0.,-0.0462787743898723,-0.0121758532865581));
#50052=UNCERTAINTY_MEASURE_WITH_UNIT(LENGTH_MEASURE(1.E-5),#50082,
'DISTANCE_ACCURACY_VALUE',
'Maximum model space distance between geometric entities at asserted c
onnectivities');
#50059=UNCERTAINTY_MEASURE_WITH_UNIT(LENGTH_MEASURE(1.E-5),#50082,
'DISTANCE_ACCURACY_VALUE',
'Maximum model space distance between geometric entities at asserted c
onnectivities');
#50074=(
GEOMETRIC_REPRESENTATION_CONTEXT(3)
GLOBAL_UNCERTAINTY_ASSIGNED_CONTEXT((#50052))
GLOBAL_UNIT_ASSIGNED_CONTEXT((#50082,#50083,#50084))
REPRESENTATION_CONTEXT('','3D')
);
#50081=(
GEOMETRIC_REPRESENTATION_CONTEXT(3)
GLOBAL_UNCERTAINTY_ASSIGNED_CONTEXT((#50059))
GLOBAL_UNIT_ASSIGNED_CONTEXT((#50082,#50083,#50084))
REPRESENTATION_CONTEXT('','3D')
);
#50082=(
LENGTH_UNIT()
NAMED_UNIT(*)
SI_UNIT($,.METRE.)
);
#50083=(
NAMED_UNIT(*)
PLANE_ANGLE_UNIT()
SI_UNIT($,.RADIAN.)
);
#50084=(
NAMED_UNIT(*)
SI_UNIT($,.STERADIAN.)
SOLID_ANGLE_UNIT()
);
#50099=SHAPE_DEFINITION_REPRESENTATION(#50120,#50161);
#50120=PRODUCT_DEFINITION_SHAPE('',$,#50183);
#50161=SHAPE_REPRESENTATION('',(#10679),#50074);
#50168=PRODUCT_DEFINITION_CONTEXT('part definition',#50233,'design');
#50183=PRODUCT_DEFINITION('Brass Thermal Extrusion Nozzle',
'Brass Thermal Extrusion Nozzle',#50204,#50168);
#50204=PRODUCT_DEFINITION_FORMATION('',$,#50249);
#50233=APPLICATION_CONTEXT('Managed model based 3d engineering');
#50234=PRODUCT_CONTEXT('part definition',#50233,'mechanical');
#50249=PRODUCT('Brass Thermal Extrusion Nozzle',
'Brass Thermal Extrusion Nozzle',
'LEGAL AND USAGE DISCLAIMER: this Data/Model is provided \X2\201C\X0\A
S IS\X2\201D\X0\ for informational and representational only. It is a 
geometric approximation and is NOT engineered, certified, or guarantee
d for dimensional accuracy, exact tolerances, or production-level prec
ision. Vendor disclaims all implied warranties including fitness for a
 particular purpose. DO NOT USE FOR DIRECT PHYSICAL MANUFACTURING, AUT
OMATED PRODUCTION, OR SAFETY-CRITICAL SYSTEMS without independent engi
neering verification and resolution of any design discrepancies.',(#50234));
#50259=PRESENTATION_STYLE_ASSIGNMENT((#50266));
#50266=SURFACE_STYLE_USAGE(.BOTH.,#50273);
#50273=SURFACE_SIDE_STYLE('',(#50280));
#50280=SURFACE_STYLE_FILL_AREA(#50287);
#50287=FILL_AREA_STYLE('Opaque(246,246,243)',(#50294));
#50294=FILL_AREA_STYLE_COLOUR('Opaque(246,246,243)',#50301);
#50301=COLOUR_RGB('Opaque(246,246,243)',0.964705882352941,0.964705882352941,
0.952941176470588);
ENDSEC;
END-ISO-10303-21;
